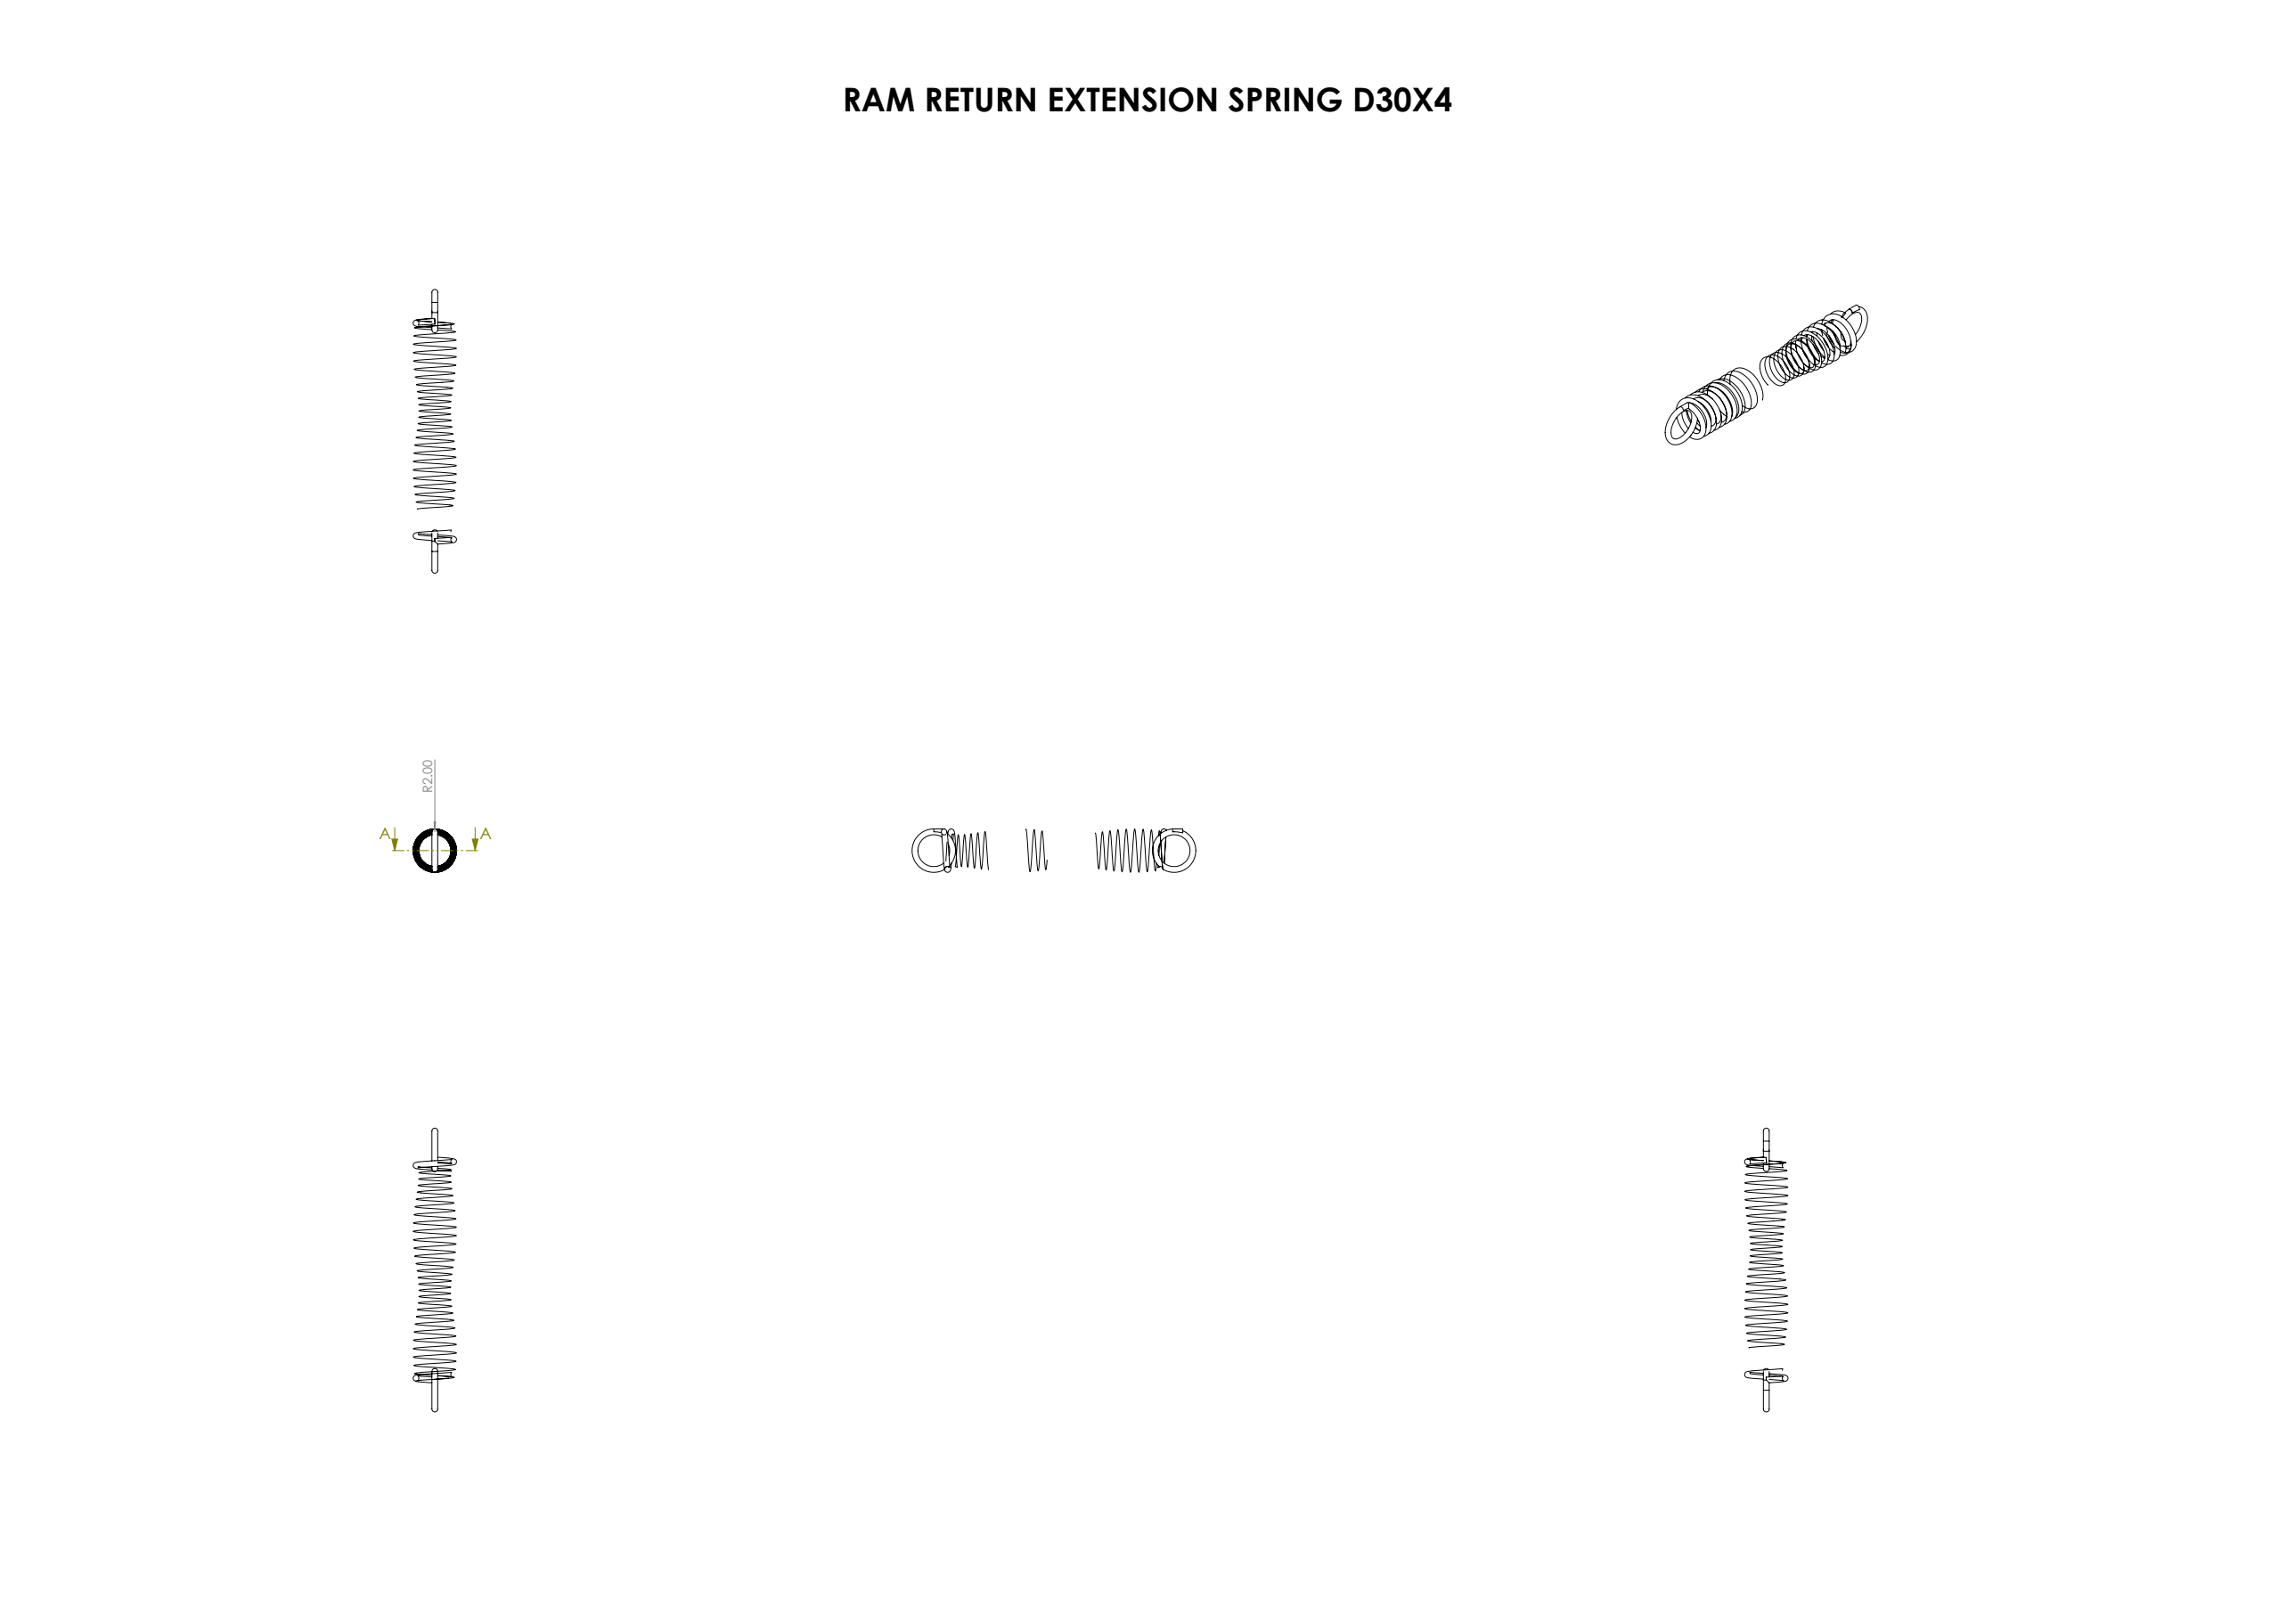
ISO-10303-21;
HEADER;
/* Generated by software containing ST-Developer
 * from STEP Tools, Inc. (www.steptools.com) 
 */

FILE_DESCRIPTION(
/* description */ (''),
/* implementation_level */ '2;1');

FILE_NAME(
/* name */ '14_Ram_Return_Extension_Spring_D30x4.step',
/* time_stamp */ '2026-10-20T10:03:03-07:00',
/* author */ (''),
/* organization */ (''),
/* preprocessor_version */ 'ST-DEVELOPER v20.2',
/* originating_system */ 'Autodesk Translation Framework v15.15.0.0',
/* authorisation */ '');

FILE_SCHEMA (('AUTOMOTIVE_DESIGN { 1 0 10303 214 3 1 1 }'));
ENDSEC;

DATA;
#10=MECHANICAL_DESIGN_GEOMETRIC_PRESENTATION_REPRESENTATION('',(#536),#71492);
#378=TOROIDAL_SURFACE('',#30165,1.30000000000001,0.199999999999999);
#379=TOROIDAL_SURFACE('',#30175,1.29999999999998,0.199999999999999);
#393=SHAPE_REPRESENTATION_RELATIONSHIP('SRR','None',#71614,#412);
#412=ADVANCED_BREP_SHAPE_REPRESENTATION('',(#431),#71484);
#431=MANIFOLD_SOLID_BREP('Spring',#28470);
#536=STYLED_ITEM('',(#71887),#431);
#890=B_SPLINE_CURVE_WITH_KNOTS('',3,(#50566,#50567,#50568,#50569,#50570,
#50571,#50572,#50573,#50574,#50575,#50576,#50577),.UNSPECIFIED.,.F.,.F.,
(4,2,2,2,2,4),(-0.933147704973241,-0.868188382212497,-0.834902175531159,
-0.786275576815645,-0.713790971965885,-0.697816473428944),.UNSPECIFIED.);
#891=B_SPLINE_CURVE_WITH_KNOTS('',3,(#50579,#50580,#50581,#50582,#50583,
#50584),.UNSPECIFIED.,.F.,.F.,(4,2,4),(1.52674033862511,1.66437329412415,
1.90849204295496),.UNSPECIFIED.);
#892=B_SPLINE_CURVE_WITH_KNOTS('',3,(#50585,#50586,#50587,#50588,#50589,
#50590,#50591,#50592,#50593,#50594,#50595,#50596,#50597,#50598,#50599,#50600,
#50601,#50602,#50603,#50604,#50605,#50606,#50607,#50608,#50609,#50610,#50611,
#50612,#50613,#50614,#50615,#50616,#50617,#50618,#50619,#50620,#50621,#50622,
#50623,#50624),.UNSPECIFIED.,.F.,.F.,(4,2,2,2,2,2,2,2,2,2,2,2,2,2,2,2,2,
2,2,4),(-0.697816473428944,-0.641492100456325,-0.561892654258354,-0.487270261093736,
-0.415523326738581,-0.352999977835186,-0.297288562200619,-0.245809461273269,
-0.188090467029938,-0.125165205371812,-0.0693938271837363,-0.0288166579795215,
-0.011031688571819,-0.00807673967083518,-0.00722367058716677,-0.00670135601612909,
-0.00622856149277745,-0.00563313335098952,-0.00468105421360917,0.),
 .UNSPECIFIED.);
#893=B_SPLINE_CURVE_WITH_KNOTS('',3,(#50626,#50627,#50628,#50629,#50630,
#50631,#50632,#50633,#50634,#50635,#50636,#50637,#50638,#50639,#50640,#50641,
#50642,#50643,#50644,#50645,#50646,#50647,#50648,#50649,#50650,#50651,#50652,
#50653,#50654,#50655,#50656,#50657,#50658,#50659,#50660,#50661,#50662,#50663,
#50664,#50665,#50666,#50667,#50668,#50669,#50670,#50671,#50672,#50673,#50674,
#50675,#50676,#50677,#50678,#50679,#50680,#50681,#50682,#50683,#50684,#50685,
#50686,#50687,#50688,#50689,#50690,#50691,#50692,#50693,#50694,#50695,#50696,
#50697,#50698,#50699,#50700,#50701,#50702,#50703),.UNSPECIFIED.,.T.,.F.,
(4,2,2,2,2,2,2,2,2,2,2,2,2,2,2,2,2,2,2,2,2,2,2,2,2,2,2,2,2,2,2,2,2,2,2,
2,2,2,4),(-1.16741385635012,-1.10893818912616,-1.06985976541729,-1.01498651099856,
-0.957285325740818,-0.898716427496627,-0.845101968396542,-0.7947628116729,
-0.745735950293246,-0.70071813649017,-0.666843371188012,-0.652997165338416,
-0.650589913669786,-0.649860176796543,-0.649408501557424,-0.649035642498711,
-0.64859072183499,-0.64786537956541,-0.645071095706766,-0.607574421195404,
-0.548734010794119,-0.48697591956556,-0.422962984513004,-0.359428990992207,
-0.305338489109769,-0.258926095287273,-0.213872662481025,-0.174949340171218,
-0.126693953481541,-0.0878751286972278,-0.0691962799768968,-0.066111534629531,
-0.0652308285619241,-0.0646975390346177,-0.0642131862427494,-0.0636068772368167,
-0.0626447206708484,-0.0580389183869797,0.),.UNSPECIFIED.);
#894=B_SPLINE_CURVE_WITH_KNOTS('',3,(#50706,#50707,#50708,#50709,#50710,
#50711),.UNSPECIFIED.,.F.,.F.,(4,2,4),(0.,0.505462201201323,0.508054856552492),
 .UNSPECIFIED.);
#895=B_SPLINE_CURVE_WITH_KNOTS('',3,(#50713,#50714,#50715,#50716,#50717,
#50718,#50719,#50720,#50721,#50722,#50723,#50724,#50725,#50726,#50727,#50728,
#50729,#50730,#50731),.UNSPECIFIED.,.F.,.F.,(4,2,2,2,3,2,2,2,4),(-0.23884634225481,
-0.226840467123682,-0.146855278175233,-0.0717726254858313,0.,0.0717726254858312,
0.146855278175234,0.226840467123682,0.238846342254813),.UNSPECIFIED.);
#896=B_SPLINE_CURVE_WITH_KNOTS('',3,(#50733,#50734,#50735,#50736,#50737,
#50738),.UNSPECIFIED.,.F.,.F.,(4,2,4),(-0.00355989556968658,0.,0.694034650560975),
 .UNSPECIFIED.);
#897=B_SPLINE_CURVE_WITH_KNOTS('',3,(#50740,#50741,#50742,#50743,#50744,
#50745),.UNSPECIFIED.,.F.,.F.,(4,2,4),(0.,0.0964705143506219,0.100030271138855),
 .UNSPECIFIED.);
#898=B_SPLINE_CURVE_WITH_KNOTS('',3,(#50747,#50748,#50749,#50750,#50751,
#50752,#50753,#50754,#50755,#50756,#50757,#50758,#50759,#50760,#50761,#50762,
#50763,#50764,#50765),.UNSPECIFIED.,.F.,.F.,(4,2,2,2,3,2,2,2,4),(0.891901698199051,
0.964304578588269,1.03849807176645,1.11257300217037,1.18656345354505,1.26055390491972,
1.33462883532365,1.40882232850183,1.48122520889105),.UNSPECIFIED.);
#899=B_SPLINE_CURVE_WITH_KNOTS('',3,(#50766,#50767,#50768,#50769,#50770,
#50771),.UNSPECIFIED.,.F.,.F.,(4,2,4),(-0.00355989556973241,0.,0.0964742753718417),
 .UNSPECIFIED.);
#900=B_SPLINE_CURVE_WITH_KNOTS('',3,(#50787,#50788,#50789,#50790,#50791,
#50792),.UNSPECIFIED.,.F.,.F.,(4,2,4),(9.80464399094971E-6,0.571610756625481,
0.573957203361489),.UNSPECIFIED.);
#901=B_SPLINE_CURVE_WITH_KNOTS('',3,(#50794,#50795,#50796,#50797,#50798,
#50799,#50800,#50801,#50802,#50803,#50804),.UNSPECIFIED.,.F.,.F.,(4,3,2,
2,4),(-0.000224177666558713,0.,0.070831562509613,0.146325160065373,0.2126836341045),
 .UNSPECIFIED.);
#902=B_SPLINE_CURVE_WITH_KNOTS('',3,(#50806,#50807,#50808,#50809,#50810,
#50811),.UNSPECIFIED.,.F.,.F.,(4,2,4),(5.93567910240686,6.07331205917363,
6.14204532250066),.UNSPECIFIED.);
#903=B_SPLINE_CURVE_WITH_KNOTS('',3,(#50813,#50814,#50815,#50816,#50817,
#50818,#50819,#50820,#50821,#50822,#50823,#50824,#50825,#50826,#50827,#50828,
#50829,#50830,#50831,#50832,#50833,#50834,#50835,#50836,#50837,#50838),
 .UNSPECIFIED.,.F.,.F.,(4,2,2,2,2,2,2,2,2,2,2,2,4),(-0.217220359894287,
-0.188091234086745,-0.125165638249208,-0.0693942084995795,-0.0288171491726731,
-0.0110319711967647,-0.00807696643551894,-0.00722387847193592,-0.00670155176446524,
-0.00622874591968683,-0.00563330291795246,-0.0046811987490239,0.),
 .UNSPECIFIED.);
#904=B_SPLINE_CURVE_WITH_KNOTS('',3,(#50840,#50841,#50842,#50843,#50844,
#50845,#50846,#50847,#50848,#50849,#50850,#50851,#50852,#50853,#50854,#50855,
#50856,#50857),.UNSPECIFIED.,.F.,.F.,(4,2,2,2,2,2,2,2,4),(-0.631559418815847,
-0.620592602298802,-0.55666742562014,-0.487473041324762,-0.420697012696697,
-0.353000616097942,-0.297289069423837,-0.245809975607455,-0.217220359894287),
 .UNSPECIFIED.);
#905=B_SPLINE_CURVE_WITH_KNOTS('',3,(#50858,#50859,#50860,#50861,#50862,
#50863),.UNSPECIFIED.,.F.,.F.,(4,2,4),(-0.00341976532710713,0.,0.574420226027791),
 .UNSPECIFIED.);
#906=B_SPLINE_CURVE_WITH_KNOTS('',3,(#50865,#50866,#50867,#50868,#50869,
#50870,#50871,#50872,#50873,#50874,#50875,#50876,#50877,#50878,#50879,#50880,
#50881,#50882,#50883,#50884,#50885,#50886,#50887,#50888,#50889,#50890,#50891,
#50892,#50893,#50894,#50895,#50896,#50897,#50898,#50899,#50900,#50901,#50902,
#50903,#50904,#50905,#50906,#50907,#50908,#50909,#50910,#50911,#50912,#50913,
#50914,#50915,#50916,#50917,#50918,#50919,#50920,#50921,#50922,#50923,#50924,
#50925,#50926,#50927,#50928,#50929,#50930,#50931,#50932,#50933,#50934,#50935,
#50936,#50937,#50938,#50939,#50940,#50941,#50942),.UNSPECIFIED.,.T.,.F.,
(4,2,2,2,2,2,2,2,2,2,2,2,2,2,2,2,2,2,2,2,2,2,2,2,2,2,2,2,2,2,2,2,2,2,2,
2,2,2,4),(-1.17168724851018,-1.13237503013972,-1.09879160541631,-1.03889691152247,
-0.981512507143146,-0.933213815656585,-0.888967230915786,-0.842464807937823,
-0.794362427770576,-0.753634236924923,-0.729805391435721,-0.726300945076248,
-0.725393129119785,-0.724861929520477,-0.724439462673908,-0.723953337160863,
-0.723043143227618,-0.7198098911947,-0.676758603427299,-0.614155893881885,
-0.553909544915966,-0.497500965420826,-0.437567654472521,-0.378252271962478,
-0.324152481036834,-0.273011005634134,-0.22337038625395,-0.178756642448113,
-0.146924605801202,-0.134819177627514,-0.133668424425745,-0.133121159543081,
-0.132739051473177,-0.132344954721629,-0.131807139835994,-0.130466280257678,
-0.116500318328084,-0.0541945170664063,0.),.UNSPECIFIED.);
#907=B_SPLINE_CURVE_WITH_KNOTS('',3,(#50950,#50951,#50952,#50953,#50954,
#50955,#50956,#50957,#50958,#50959,#50960,#50961,#50962,#50963,#50964,#50965),
 .UNSPECIFIED.,.F.,.F.,(4,2,2,2,2,2,2,4),(-0.892813994576797,-0.891702748036019,
-0.737380938279843,-0.613095387365794,-0.519181223685694,-0.442588537124146,
-0.369088033168532,-0.363543775985196),.UNSPECIFIED.);
#908=B_SPLINE_CURVE_WITH_KNOTS('',3,(#56488,#56489,#56490,#56491,#56492,
#56493,#56494,#56495,#56496,#56497,#56498,#56499,#56500,#56501,#56502,#56503,
#56504,#56505,#56506,#56507,#56508,#56509,#56510,#56511,#56512,#56513,#56514,
#56515,#56516,#56517,#56518,#56519,#56520,#56521,#56522,#56523,#56524,#56525,
#56526,#56527,#56528,#56529,#56530,#56531,#56532,#56533,#56534,#56535,#56536,
#56537,#56538,#56539,#56540,#56541,#56542,#56543,#56544,#56545,#56546,#56547,
#56548,#56549,#56550,#56551,#56552,#56553,#56554,#56555,#56556,#56557,#56558,
#56559,#56560,#56561,#56562,#56563,#56564,#56565,#56566,#56567,#56568,#56569,
#56570,#56571,#56572,#56573,#56574,#56575,#56576,#56577,#56578,#56579,#56580,
#56581,#56582,#56583,#56584,#56585,#56586,#56587,#56588,#56589,#56590,#56591,
#56592,#56593,#56594,#56595,#56596,#56597,#56598,#56599,#56600,#56601,#56602,
#56603,#56604,#56605,#56606,#56607,#56608,#56609,#56610,#56611,#56612,#56613,
#56614,#56615,#56616,#56617,#56618,#56619,#56620,#56621,#56622,#56623,#56624,
#56625,#56626,#56627,#56628,#56629,#56630,#56631,#56632,#56633,#56634,#56635,
#56636,#56637,#56638,#56639,#56640,#56641,#56642,#56643,#56644,#56645,#56646,
#56647,#56648,#56649,#56650,#56651,#56652,#56653,#56654,#56655,#56656,#56657,
#56658,#56659,#56660,#56661,#56662,#56663,#56664,#56665,#56666,#56667,#56668,
#56669,#56670,#56671,#56672,#56673,#56674,#56675,#56676,#56677,#56678,#56679,
#56680,#56681,#56682,#56683,#56684,#56685,#56686,#56687,#56688,#56689,#56690,
#56691,#56692,#56693,#56694,#56695,#56696,#56697,#56698,#56699,#56700,#56701,
#56702,#56703,#56704,#56705,#56706,#56707,#56708,#56709,#56710,#56711,#56712,
#56713,#56714,#56715,#56716,#56717,#56718,#56719,#56720,#56721,#56722,#56723,
#56724,#56725,#56726,#56727,#56728,#56729,#56730,#56731,#56732,#56733,#56734,
#56735,#56736,#56737,#56738,#56739,#56740,#56741,#56742,#56743,#56744,#56745,
#56746,#56747,#56748,#56749,#56750,#56751,#56752,#56753,#56754,#56755,#56756,
#56757,#56758,#56759,#56760,#56761,#56762,#56763,#56764,#56765,#56766,#56767,
#56768,#56769,#56770,#56771,#56772,#56773,#56774,#56775,#56776,#56777,#56778,
#56779,#56780,#56781,#56782,#56783,#56784,#56785,#56786,#56787,#56788,#56789,
#56790,#56791,#56792,#56793,#56794,#56795,#56796,#56797,#56798,#56799,#56800,
#56801,#56802,#56803,#56804,#56805,#56806,#56807,#56808,#56809,#56810,#56811,
#56812,#56813,#56814,#56815,#56816,#56817,#56818,#56819,#56820,#56821,#56822,
#56823,#56824,#56825,#56826,#56827,#56828,#56829,#56830,#56831,#56832,#56833,
#56834,#56835,#56836,#56837,#56838,#56839,#56840,#56841,#56842,#56843,#56844,
#56845,#56846,#56847,#56848,#56849,#56850,#56851,#56852,#56853,#56854,#56855,
#56856,#56857,#56858,#56859,#56860,#56861,#56862,#56863,#56864,#56865,#56866,
#56867,#56868,#56869,#56870,#56871,#56872,#56873,#56874,#56875,#56876,#56877,
#56878,#56879,#56880,#56881,#56882,#56883,#56884,#56885,#56886,#56887,#56888,
#56889,#56890,#56891,#56892,#56893,#56894,#56895,#56896,#56897,#56898,#56899,
#56900,#56901,#56902,#56903,#56904,#56905,#56906,#56907,#56908,#56909,#56910,
#56911,#56912,#56913,#56914,#56915,#56916,#56917,#56918,#56919,#56920,#56921,
#56922,#56923,#56924,#56925,#56926,#56927,#56928,#56929,#56930,#56931,#56932,
#56933,#56934,#56935,#56936,#56937,#56938,#56939,#56940,#56941,#56942,#56943,
#56944,#56945,#56946,#56947,#56948,#56949,#56950,#56951,#56952,#56953,#56954,
#56955,#56956,#56957,#56958,#56959,#56960,#56961,#56962,#56963,#56964,#56965,
#56966,#56967,#56968,#56969,#56970,#56971,#56972,#56973,#56974,#56975,#56976,
#56977,#56978,#56979,#56980,#56981,#56982,#56983,#56984,#56985,#56986,#56987,
#56988,#56989),.UNSPECIFIED.,.F.,.F.,(4,1,1,1,1,1,1,1,1,1,1,1,1,1,1,1,1,
1,1,1,1,1,1,1,1,1,1,1,1,1,1,1,1,1,1,1,1,1,1,1,1,1,1,1,1,1,1,1,1,1,1,1,1,
1,1,1,1,1,1,1,1,1,1,1,1,1,1,1,1,1,1,1,1,1,1,1,1,1,1,1,1,1,1,1,1,1,1,1,1,
1,1,1,1,1,1,1,1,1,1,1,1,1,1,1,1,1,1,1,1,1,1,1,1,1,1,1,1,1,1,1,1,1,1,1,1,
1,1,1,1,1,1,1,1,1,1,1,1,1,1,1,1,1,1,1,1,1,1,1,1,1,1,1,1,1,1,1,1,1,1,1,1,
1,1,1,1,1,1,1,1,1,1,1,1,1,1,1,1,1,1,1,1,1,1,1,1,1,1,1,1,1,1,1,1,1,1,1,1,
1,1,1,1,1,1,1,1,1,1,1,1,1,1,1,1,1,1,1,1,1,1,1,1,1,1,1,1,1,1,1,1,1,1,1,1,
1,1,1,1,1,1,1,1,1,1,1,1,1,1,1,1,1,1,1,1,1,1,1,1,1,1,1,1,1,1,1,1,1,1,1,1,
1,1,1,1,1,1,1,1,1,1,1,1,1,1,1,1,1,1,1,1,1,1,1,1,1,1,1,1,1,1,1,1,1,1,1,1,
1,1,1,1,1,1,1,1,1,1,1,1,1,1,1,1,1,1,1,1,1,1,1,1,1,1,1,1,1,1,1,1,1,1,1,1,
1,1,1,1,1,1,1,1,1,1,1,1,1,1,1,1,1,1,1,1,1,1,1,1,1,1,1,1,1,1,1,1,1,1,1,1,
1,1,1,1,1,1,1,1,1,1,1,1,1,1,1,1,1,1,1,1,1,1,1,1,1,1,1,1,1,1,1,1,1,1,1,1,
1,1,1,1,1,1,1,1,1,1,1,1,1,1,1,1,1,1,1,1,1,1,1,1,1,1,1,1,1,1,1,1,1,1,1,1,
1,1,1,1,1,1,1,1,1,1,1,1,1,1,1,1,1,1,1,1,1,1,1,1,1,1,1,1,1,1,1,1,1,1,1,1,
1,1,1,1,1,1,1,1,1,1,1,1,1,1,4),(0.000669054243018642,0.00167410714285714,
0.00223214285714286,0.00334821428571429,0.00446428571428571,0.00558035714285714,
0.00669642857142857,0.00892857142857143,0.0111607142857143,0.0133928571428571,
0.015625,0.0178571428571429,0.0200892857142857,0.0223214285714286,0.0245535714285714,
0.0267857142857143,0.0290178571428571,0.03125,0.0334821428571429,0.0357142857142857,
0.0379464285714286,0.0401785714285714,0.0424107142857143,0.0446428571428571,
0.046875,0.0491071428571428,0.0513392857142857,0.0535714285714286,0.0558035714285714,
0.0580357142857143,0.0602678571428571,0.0625,0.0647321428571428,0.0669642857142857,
0.0680803571428572,0.0691964285714286,0.0714285714285714,0.0736607142857143,
0.0758928571428571,0.078125,0.0803571428571428,0.0825892857142857,0.0848214285714286,
0.0870535714285714,0.0892857142857143,0.0915178571428571,0.09375,0.0959821428571428,
0.0982142857142857,0.100446428571429,0.102678571428571,0.104910714285714,
0.107142857142857,0.109375,0.111607142857143,0.113839285714286,0.116071428571429,
0.118303571428571,0.119419642857143,0.120535714285714,0.122767857142857,
0.125,0.127232142857143,0.129464285714286,0.131696428571429,0.133928571428571,
0.136160714285714,0.138392857142857,0.140625,0.142857142857143,0.144345238095238,
0.145833333333333,0.146205357142857,0.146577380952381,0.146949404761905,
0.147321428571429,0.148809523809524,0.150297619047619,0.151785714285714,
0.15327380952381,0.154761904761905,0.15625,0.157738095238095,0.160714285714286,
0.162202380952381,0.162946428571429,0.163690476190476,0.165178571428571,
0.165550595238095,0.165922619047619,0.166294642857143,0.166480654761905,
0.166666666666667,0.169312169312169,0.171957671957672,0.172839506172839,
0.173721340388007,0.174162257495591,0.174603174603175,0.177248677248677,
0.17989417989418,0.182539682539683,0.18452380952381,0.186507936507937,0.188492063492063,
0.19047619047619,0.191468253968254,0.192460317460317,0.193452380952381,
0.193948412698413,0.194444444444444,0.196428571428571,0.198412698412698,
0.200396825396825,0.202380952380952,0.202876984126984,0.203373015873016,
0.204365079365079,0.206349206349206,0.206597222222222,0.206845238095238,
0.207093253968254,0.20734126984127,0.207589285714286,0.207837301587302,
0.208333333333333,0.21031746031746,0.212301587301587,0.214285714285714,
0.216269841269841,0.218253968253968,0.220238095238095,0.222222222222222,
0.222883597883598,0.223544973544974,0.224867724867725,0.227513227513228,
0.23015873015873,0.232804232804233,0.235449735449735,0.238095238095238,
0.239583333333333,0.241071428571429,0.244047619047619,0.247023809523809,
0.25,0.25297619047619,0.255952380952381,0.258928571428571,0.260416666666667,
0.261904761904762,0.263392857142857,0.264880952380952,0.267857142857143,
0.270833333333333,0.273809523809524,0.276785714285714,0.279761904761905,
0.282738095238095,0.285714285714286,0.288690476190476,0.291666666666667,
0.294642857142857,0.297619047619048,0.300595238095238,0.303571428571429,
0.306547619047619,0.30952380952381,0.3125,0.31547619047619,0.318452380952381,
0.321428571428571,0.324404761904762,0.327380952380952,0.328869047619048,
0.330357142857143,0.333333333333333,0.336309523809524,0.339285714285714,
0.342261904761905,0.345238095238095,0.348214285714286,0.351190476190476,
0.354166666666667,0.357142857142857,0.360119047619048,0.363095238095238,
0.366071428571428,0.367559523809524,0.369047619047619,0.370535714285714,
0.37202380952381,0.373511904761905,0.375,0.376488095238095,0.37797619047619,
0.378720238095238,0.379464285714286,0.380952380952381,0.383928571428571,
0.386904761904762,0.389880952380952,0.391369047619048,0.392113095238095,
0.392857142857143,0.394345238095238,0.395833333333333,0.398809523809524,
0.401785714285714,0.404761904761905,0.407738095238095,0.40922619047619,
0.410714285714286,0.411458333333333,0.411830357142857,0.412202380952381,
0.412946428571429,0.413690476190476,0.415178571428571,0.416666666666667,
0.418154761904762,0.419642857142857,0.421130952380952,0.422619047619048,
0.424107142857143,0.425595238095238,0.427083333333333,0.427827380952381,
0.428571428571429,0.430803571428571,0.433035714285714,0.435267857142857,
0.4375,0.439732142857143,0.441964285714286,0.444196428571429,0.446428571428571,
0.447544642857143,0.448660714285714,0.450892857142857,0.453125,0.455357142857143,
0.457589285714286,0.459821428571429,0.462053571428571,0.464285714285714,
0.466517857142857,0.46875,0.470982142857143,0.472098214285714,0.473214285714286,
0.475446428571429,0.477678571428571,0.479910714285714,0.482142857142857,
0.484375,0.486607142857143,0.488839285714286,0.491071428571429,0.493303571428571,
0.495535714285714,0.497767857142857,0.5,0.502232142857143,0.504464285714286,
0.506696428571429,0.508928571428571,0.511160714285714,0.513392857142857,
0.515625,0.517857142857143,0.520089285714286,0.522321428571428,0.524553571428571,
0.526785714285714,0.529017857142857,0.53125,0.533482142857143,0.535714285714286,
0.537946428571429,0.540178571428571,0.542410714285714,0.544642857142857,
0.545200892857143,0.545758928571429,0.546875,0.549107142857143,0.551339285714286,
0.553571428571429,0.555803571428571,0.558035714285714,0.560267857142857,
0.5625,0.564732142857143,0.566964285714286,0.569196428571429,0.571428571428571,
0.573660714285714,0.575892857142857,0.578125,0.580357142857143,0.582589285714286,
0.584821428571428,0.587053571428571,0.589285714285714,0.591517857142857,
0.59375,0.595982142857143,0.598214285714286,0.600446428571428,0.602678571428571,
0.604910714285714,0.607142857142857,0.609375,0.611607142857143,0.613839285714286,
0.616071428571429,0.618303571428571,0.620535714285714,0.622767857142857,
0.625,0.627232142857143,0.629464285714286,0.631696428571429,0.633928571428571,
0.636160714285714,0.638392857142857,0.640625,0.642857142857143,0.644345238095238,
0.645833333333333,0.648809523809524,0.651785714285714,0.654761904761905,
0.657738095238095,0.660714285714286,0.663690476190476,0.665178571428571,
0.666666666666667,0.667989417989418,0.669312169312169,0.671957671957672,
0.674603174603175,0.675925925925926,0.677248677248677,0.67989417989418,
0.682539682539682,0.684523809523809,0.686507936507936,0.688492063492063,
0.69047619047619,0.692460317460317,0.694444444444444,0.696428571428571,
0.697420634920635,0.698412698412698,0.701058201058201,0.703703703703704,
0.705026455026455,0.706349206349206,0.707671957671958,0.71031746031746,
0.712301587301587,0.714285714285714,0.716517857142857,0.71875,0.720982142857143,
0.72265625,0.723214285714286,0.724702380952381,0.726190476190476,0.727678571428571,
0.729166666666667,0.730654761904762,0.732142857142857,0.733258928571428,
0.734375,0.736607142857143,0.738839285714286,0.741071428571428,0.743303571428571,
0.745535714285714,0.747767857142857,0.75,0.752232142857143,0.754464285714286,
0.756696428571428,0.758928571428571,0.761160714285714,0.763392857142857,
0.765625,0.767857142857143,0.770089285714286,0.772321428571428,0.774553571428571,
0.776785714285714,0.779017857142857,0.78125,0.783482142857143,0.785714285714286,
0.787946428571428,0.790178571428571,0.792410714285714,0.794642857142857,
0.796875,0.799107142857143,0.801339285714286,0.803571428571428,0.805803571428571,
0.808035714285714,0.810267857142857,0.8125,0.814732142857143,0.816964285714286,
0.819196428571429,0.821428571428571,0.823660714285714,0.825892857142857,
0.828125,0.830357142857143,0.832589285714286,0.834821428571428,0.837053571428571,
0.839285714285714,0.841517857142857,0.84375,0.845982142857143,0.848214285714286,
0.850446428571428,0.852678571428571,0.854910714285714,0.857142857142857,
0.859375,0.861607142857143,0.863839285714286,0.866071428571429,0.868303571428571,
0.870535714285714,0.872767857142857,0.875,0.877232142857143,0.879464285714286,
0.881696428571429,0.883928571428571,0.886160714285714,0.888392857142857,
0.890625,0.892857142857143,0.895089285714286,0.897321428571428,0.899553571428571,
0.901785714285714,0.904017857142857,0.90625,0.908482142857143,0.910714285714286,
0.912946428571429,0.915178571428571,0.917410714285714,0.919642857142857,
0.921875,0.922991071428571,0.924107142857143,0.926339285714286,0.928571428571429,
0.930803571428571,0.933035714285714,0.935267857142857,0.9375,0.939732142857143,
0.941964285714286,0.944196428571429,0.946428571428571,0.948660714285714,
0.950892857142857,0.953125,0.955357142857143,0.957589285714286,0.959821428571429,
0.962053571428571,0.964285714285714,0.966517857142857,0.96875,0.970982142857143,
0.973214285714286,0.975446428571429,0.977678571428572,0.979910714285714,
0.982142857142857,0.984375,0.986607142857143,0.988839285714286,0.991071428571429,
0.993303571428571,0.994419642857143,0.995535714285714,0.996651785714286,
0.997767857142857,0.998883928571429,0.999194256023389),.UNSPECIFIED.);
#1461=B_SPLINE_SURFACE_WITH_KNOTS('',3,3,((#50966,#50967,#50968,#50969,
#50970,#50971,#50972,#50973,#50974,#50975,#50976,#50977,#50978,#50979,#50980,
#50981,#50982,#50983,#50984,#50985,#50986,#50987,#50988,#50989,#50990,#50991,
#50992,#50993,#50994,#50995,#50996,#50997,#50998,#50999,#51000,#51001,#51002,
#51003,#51004,#51005,#51006,#51007,#51008,#51009,#51010,#51011,#51012,#51013,
#51014,#51015,#51016,#51017,#51018,#51019,#51020,#51021,#51022,#51023,#51024,
#51025,#51026,#51027,#51028,#51029,#51030,#51031,#51032,#51033,#51034,#51035,
#51036,#51037,#51038,#51039,#51040,#51041,#51042,#51043,#51044,#51045,#51046,
#51047,#51048,#51049,#51050,#51051,#51052,#51053,#51054,#51055,#51056,#51057,
#51058,#51059,#51060,#51061,#51062,#51063,#51064,#51065,#51066,#51067,#51068,
#51069,#51070,#51071,#51072,#51073,#51074,#51075,#51076,#51077,#51078,#51079,
#51080,#51081,#51082,#51083,#51084,#51085,#51086,#51087,#51088,#51089,#51090,
#51091,#51092,#51093,#51094,#51095,#51096,#51097,#51098,#51099,#51100,#51101,
#51102,#51103,#51104,#51105,#51106,#51107,#51108,#51109,#51110,#51111,#51112,
#51113,#51114,#51115,#51116,#51117,#51118,#51119,#51120,#51121,#51122,#51123,
#51124,#51125,#51126,#51127,#51128,#51129,#51130,#51131,#51132,#51133,#51134,
#51135,#51136,#51137,#51138,#51139,#51140,#51141,#51142,#51143,#51144,#51145,
#51146,#51147,#51148,#51149,#51150,#51151,#51152,#51153,#51154,#51155,#51156,
#51157,#51158,#51159,#51160,#51161,#51162,#51163,#51164,#51165,#51166,#51167,
#51168,#51169,#51170,#51171,#51172,#51173,#51174,#51175,#51176,#51177,#51178,
#51179,#51180,#51181,#51182,#51183,#51184,#51185,#51186,#51187,#51188,#51189,
#51190,#51191,#51192,#51193,#51194,#51195,#51196,#51197,#51198,#51199,#51200,
#51201,#51202,#51203,#51204,#51205,#51206,#51207,#51208,#51209,#51210,#51211,
#51212,#51213,#51214,#51215,#51216,#51217,#51218,#51219,#51220,#51221,#51222,
#51223,#51224,#51225,#51226,#51227,#51228,#51229,#51230,#51231,#51232,#51233,
#51234,#51235,#51236,#51237,#51238,#51239,#51240,#51241,#51242,#51243,#51244,
#51245,#51246,#51247,#51248,#51249,#51250,#51251,#51252,#51253,#51254,#51255,
#51256,#51257,#51258,#51259,#51260,#51261,#51262,#51263,#51264,#51265,#51266,
#51267,#51268,#51269,#51270,#51271,#51272,#51273,#51274,#51275,#51276,#51277,
#51278,#51279,#51280,#51281,#51282,#51283,#51284,#51285,#51286,#51287,#51288,
#51289,#51290,#51291,#51292,#51293,#51294,#51295,#51296,#51297,#51298,#51299,
#51300,#51301,#51302,#51303,#51304,#51305,#51306,#51307,#51308,#51309,#51310,
#51311,#51312,#51313,#51314,#51315,#51316,#51317,#51318,#51319,#51320,#51321,
#51322,#51323,#51324,#51325,#51326,#51327,#51328,#51329,#51330,#51331,#51332,
#51333,#51334,#51335,#51336,#51337,#51338,#51339,#51340,#51341,#51342,#51343,
#51344,#51345,#51346,#51347,#51348,#51349,#51350,#51351,#51352,#51353,#51354,
#51355,#51356,#51357,#51358,#51359,#51360,#51361,#51362,#51363,#51364,#51365,
#51366,#51367,#51368,#51369,#51370,#51371,#51372,#51373,#51374,#51375,#51376,
#51377,#51378,#51379,#51380,#51381,#51382,#51383,#51384,#51385,#51386,#51387,
#51388,#51389,#51390,#51391,#51392,#51393,#51394,#51395,#51396,#51397,#51398,
#51399,#51400,#51401,#51402,#51403,#51404,#51405,#51406,#51407,#51408,#51409,
#51410,#51411,#51412,#51413,#51414,#51415,#51416,#51417,#51418,#51419,#51420,
#51421,#51422,#51423,#51424,#51425,#51426,#51427,#51428,#51429,#51430,#51431,
#51432,#51433,#51434,#51435,#51436,#51437,#51438,#51439,#51440,#51441,#51442,
#51443,#51444,#51445,#51446,#51447,#51448,#51449,#51450,#51451,#51452,#51453,
#51454,#51455,#51456,#51457,#51458,#51459,#51460,#51461,#51462,#51463,#51464,
#51465,#51466,#51467),(#51468,#51469,#51470,#51471,#51472,#51473,#51474,
#51475,#51476,#51477,#51478,#51479,#51480,#51481,#51482,#51483,#51484,#51485,
#51486,#51487,#51488,#51489,#51490,#51491,#51492,#51493,#51494,#51495,#51496,
#51497,#51498,#51499,#51500,#51501,#51502,#51503,#51504,#51505,#51506,#51507,
#51508,#51509,#51510,#51511,#51512,#51513,#51514,#51515,#51516,#51517,#51518,
#51519,#51520,#51521,#51522,#51523,#51524,#51525,#51526,#51527,#51528,#51529,
#51530,#51531,#51532,#51533,#51534,#51535,#51536,#51537,#51538,#51539,#51540,
#51541,#51542,#51543,#51544,#51545,#51546,#51547,#51548,#51549,#51550,#51551,
#51552,#51553,#51554,#51555,#51556,#51557,#51558,#51559,#51560,#51561,#51562,
#51563,#51564,#51565,#51566,#51567,#51568,#51569,#51570,#51571,#51572,#51573,
#51574,#51575,#51576,#51577,#51578,#51579,#51580,#51581,#51582,#51583,#51584,
#51585,#51586,#51587,#51588,#51589,#51590,#51591,#51592,#51593,#51594,#51595,
#51596,#51597,#51598,#51599,#51600,#51601,#51602,#51603,#51604,#51605,#51606,
#51607,#51608,#51609,#51610,#51611,#51612,#51613,#51614,#51615,#51616,#51617,
#51618,#51619,#51620,#51621,#51622,#51623,#51624,#51625,#51626,#51627,#51628,
#51629,#51630,#51631,#51632,#51633,#51634,#51635,#51636,#51637,#51638,#51639,
#51640,#51641,#51642,#51643,#51644,#51645,#51646,#51647,#51648,#51649,#51650,
#51651,#51652,#51653,#51654,#51655,#51656,#51657,#51658,#51659,#51660,#51661,
#51662,#51663,#51664,#51665,#51666,#51667,#51668,#51669,#51670,#51671,#51672,
#51673,#51674,#51675,#51676,#51677,#51678,#51679,#51680,#51681,#51682,#51683,
#51684,#51685,#51686,#51687,#51688,#51689,#51690,#51691,#51692,#51693,#51694,
#51695,#51696,#51697,#51698,#51699,#51700,#51701,#51702,#51703,#51704,#51705,
#51706,#51707,#51708,#51709,#51710,#51711,#51712,#51713,#51714,#51715,#51716,
#51717,#51718,#51719,#51720,#51721,#51722,#51723,#51724,#51725,#51726,#51727,
#51728,#51729,#51730,#51731,#51732,#51733,#51734,#51735,#51736,#51737,#51738,
#51739,#51740,#51741,#51742,#51743,#51744,#51745,#51746,#51747,#51748,#51749,
#51750,#51751,#51752,#51753,#51754,#51755,#51756,#51757,#51758,#51759,#51760,
#51761,#51762,#51763,#51764,#51765,#51766,#51767,#51768,#51769,#51770,#51771,
#51772,#51773,#51774,#51775,#51776,#51777,#51778,#51779,#51780,#51781,#51782,
#51783,#51784,#51785,#51786,#51787,#51788,#51789,#51790,#51791,#51792,#51793,
#51794,#51795,#51796,#51797,#51798,#51799,#51800,#51801,#51802,#51803,#51804,
#51805,#51806,#51807,#51808,#51809,#51810,#51811,#51812,#51813,#51814,#51815,
#51816,#51817,#51818,#51819,#51820,#51821,#51822,#51823,#51824,#51825,#51826,
#51827,#51828,#51829,#51830,#51831,#51832,#51833,#51834,#51835,#51836,#51837,
#51838,#51839,#51840,#51841,#51842,#51843,#51844,#51845,#51846,#51847,#51848,
#51849,#51850,#51851,#51852,#51853,#51854,#51855,#51856,#51857,#51858,#51859,
#51860,#51861,#51862,#51863,#51864,#51865,#51866,#51867,#51868,#51869,#51870,
#51871,#51872,#51873,#51874,#51875,#51876,#51877,#51878,#51879,#51880,#51881,
#51882,#51883,#51884,#51885,#51886,#51887,#51888,#51889,#51890,#51891,#51892,
#51893,#51894,#51895,#51896,#51897,#51898,#51899,#51900,#51901,#51902,#51903,
#51904,#51905,#51906,#51907,#51908,#51909,#51910,#51911,#51912,#51913,#51914,
#51915,#51916,#51917,#51918,#51919,#51920,#51921,#51922,#51923,#51924,#51925,
#51926,#51927,#51928,#51929,#51930,#51931,#51932,#51933,#51934,#51935,#51936,
#51937,#51938,#51939,#51940,#51941,#51942,#51943,#51944,#51945,#51946,#51947,
#51948,#51949,#51950,#51951,#51952,#51953,#51954,#51955,#51956,#51957,#51958,
#51959,#51960,#51961,#51962,#51963,#51964,#51965,#51966,#51967,#51968,#51969),
(#51970,#51971,#51972,#51973,#51974,#51975,#51976,#51977,#51978,#51979,
#51980,#51981,#51982,#51983,#51984,#51985,#51986,#51987,#51988,#51989,#51990,
#51991,#51992,#51993,#51994,#51995,#51996,#51997,#51998,#51999,#52000,#52001,
#52002,#52003,#52004,#52005,#52006,#52007,#52008,#52009,#52010,#52011,#52012,
#52013,#52014,#52015,#52016,#52017,#52018,#52019,#52020,#52021,#52022,#52023,
#52024,#52025,#52026,#52027,#52028,#52029,#52030,#52031,#52032,#52033,#52034,
#52035,#52036,#52037,#52038,#52039,#52040,#52041,#52042,#52043,#52044,#52045,
#52046,#52047,#52048,#52049,#52050,#52051,#52052,#52053,#52054,#52055,#52056,
#52057,#52058,#52059,#52060,#52061,#52062,#52063,#52064,#52065,#52066,#52067,
#52068,#52069,#52070,#52071,#52072,#52073,#52074,#52075,#52076,#52077,#52078,
#52079,#52080,#52081,#52082,#52083,#52084,#52085,#52086,#52087,#52088,#52089,
#52090,#52091,#52092,#52093,#52094,#52095,#52096,#52097,#52098,#52099,#52100,
#52101,#52102,#52103,#52104,#52105,#52106,#52107,#52108,#52109,#52110,#52111,
#52112,#52113,#52114,#52115,#52116,#52117,#52118,#52119,#52120,#52121,#52122,
#52123,#52124,#52125,#52126,#52127,#52128,#52129,#52130,#52131,#52132,#52133,
#52134,#52135,#52136,#52137,#52138,#52139,#52140,#52141,#52142,#52143,#52144,
#52145,#52146,#52147,#52148,#52149,#52150,#52151,#52152,#52153,#52154,#52155,
#52156,#52157,#52158,#52159,#52160,#52161,#52162,#52163,#52164,#52165,#52166,
#52167,#52168,#52169,#52170,#52171,#52172,#52173,#52174,#52175,#52176,#52177,
#52178,#52179,#52180,#52181,#52182,#52183,#52184,#52185,#52186,#52187,#52188,
#52189,#52190,#52191,#52192,#52193,#52194,#52195,#52196,#52197,#52198,#52199,
#52200,#52201,#52202,#52203,#52204,#52205,#52206,#52207,#52208,#52209,#52210,
#52211,#52212,#52213,#52214,#52215,#52216,#52217,#52218,#52219,#52220,#52221,
#52222,#52223,#52224,#52225,#52226,#52227,#52228,#52229,#52230,#52231,#52232,
#52233,#52234,#52235,#52236,#52237,#52238,#52239,#52240,#52241,#52242,#52243,
#52244,#52245,#52246,#52247,#52248,#52249,#52250,#52251,#52252,#52253,#52254,
#52255,#52256,#52257,#52258,#52259,#52260,#52261,#52262,#52263,#52264,#52265,
#52266,#52267,#52268,#52269,#52270,#52271,#52272,#52273,#52274,#52275,#52276,
#52277,#52278,#52279,#52280,#52281,#52282,#52283,#52284,#52285,#52286,#52287,
#52288,#52289,#52290,#52291,#52292,#52293,#52294,#52295,#52296,#52297,#52298,
#52299,#52300,#52301,#52302,#52303,#52304,#52305,#52306,#52307,#52308,#52309,
#52310,#52311,#52312,#52313,#52314,#52315,#52316,#52317,#52318,#52319,#52320,
#52321,#52322,#52323,#52324,#52325,#52326,#52327,#52328,#52329,#52330,#52331,
#52332,#52333,#52334,#52335,#52336,#52337,#52338,#52339,#52340,#52341,#52342,
#52343,#52344,#52345,#52346,#52347,#52348,#52349,#52350,#52351,#52352,#52353,
#52354,#52355,#52356,#52357,#52358,#52359,#52360,#52361,#52362,#52363,#52364,
#52365,#52366,#52367,#52368,#52369,#52370,#52371,#52372,#52373,#52374,#52375,
#52376,#52377,#52378,#52379,#52380,#52381,#52382,#52383,#52384,#52385,#52386,
#52387,#52388,#52389,#52390,#52391,#52392,#52393,#52394,#52395,#52396,#52397,
#52398,#52399,#52400,#52401,#52402,#52403,#52404,#52405,#52406,#52407,#52408,
#52409,#52410,#52411,#52412,#52413,#52414,#52415,#52416,#52417,#52418,#52419,
#52420,#52421,#52422,#52423,#52424,#52425,#52426,#52427,#52428,#52429,#52430,
#52431,#52432,#52433,#52434,#52435,#52436,#52437,#52438,#52439,#52440,#52441,
#52442,#52443,#52444,#52445,#52446,#52447,#52448,#52449,#52450,#52451,#52452,
#52453,#52454,#52455,#52456,#52457,#52458,#52459,#52460,#52461,#52462,#52463,
#52464,#52465,#52466,#52467,#52468,#52469,#52470,#52471),(#52472,#52473,
#52474,#52475,#52476,#52477,#52478,#52479,#52480,#52481,#52482,#52483,#52484,
#52485,#52486,#52487,#52488,#52489,#52490,#52491,#52492,#52493,#52494,#52495,
#52496,#52497,#52498,#52499,#52500,#52501,#52502,#52503,#52504,#52505,#52506,
#52507,#52508,#52509,#52510,#52511,#52512,#52513,#52514,#52515,#52516,#52517,
#52518,#52519,#52520,#52521,#52522,#52523,#52524,#52525,#52526,#52527,#52528,
#52529,#52530,#52531,#52532,#52533,#52534,#52535,#52536,#52537,#52538,#52539,
#52540,#52541,#52542,#52543,#52544,#52545,#52546,#52547,#52548,#52549,#52550,
#52551,#52552,#52553,#52554,#52555,#52556,#52557,#52558,#52559,#52560,#52561,
#52562,#52563,#52564,#52565,#52566,#52567,#52568,#52569,#52570,#52571,#52572,
#52573,#52574,#52575,#52576,#52577,#52578,#52579,#52580,#52581,#52582,#52583,
#52584,#52585,#52586,#52587,#52588,#52589,#52590,#52591,#52592,#52593,#52594,
#52595,#52596,#52597,#52598,#52599,#52600,#52601,#52602,#52603,#52604,#52605,
#52606,#52607,#52608,#52609,#52610,#52611,#52612,#52613,#52614,#52615,#52616,
#52617,#52618,#52619,#52620,#52621,#52622,#52623,#52624,#52625,#52626,#52627,
#52628,#52629,#52630,#52631,#52632,#52633,#52634,#52635,#52636,#52637,#52638,
#52639,#52640,#52641,#52642,#52643,#52644,#52645,#52646,#52647,#52648,#52649,
#52650,#52651,#52652,#52653,#52654,#52655,#52656,#52657,#52658,#52659,#52660,
#52661,#52662,#52663,#52664,#52665,#52666,#52667,#52668,#52669,#52670,#52671,
#52672,#52673,#52674,#52675,#52676,#52677,#52678,#52679,#52680,#52681,#52682,
#52683,#52684,#52685,#52686,#52687,#52688,#52689,#52690,#52691,#52692,#52693,
#52694,#52695,#52696,#52697,#52698,#52699,#52700,#52701,#52702,#52703,#52704,
#52705,#52706,#52707,#52708,#52709,#52710,#52711,#52712,#52713,#52714,#52715,
#52716,#52717,#52718,#52719,#52720,#52721,#52722,#52723,#52724,#52725,#52726,
#52727,#52728,#52729,#52730,#52731,#52732,#52733,#52734,#52735,#52736,#52737,
#52738,#52739,#52740,#52741,#52742,#52743,#52744,#52745,#52746,#52747,#52748,
#52749,#52750,#52751,#52752,#52753,#52754,#52755,#52756,#52757,#52758,#52759,
#52760,#52761,#52762,#52763,#52764,#52765,#52766,#52767,#52768,#52769,#52770,
#52771,#52772,#52773,#52774,#52775,#52776,#52777,#52778,#52779,#52780,#52781,
#52782,#52783,#52784,#52785,#52786,#52787,#52788,#52789,#52790,#52791,#52792,
#52793,#52794,#52795,#52796,#52797,#52798,#52799,#52800,#52801,#52802,#52803,
#52804,#52805,#52806,#52807,#52808,#52809,#52810,#52811,#52812,#52813,#52814,
#52815,#52816,#52817,#52818,#52819,#52820,#52821,#52822,#52823,#52824,#52825,
#52826,#52827,#52828,#52829,#52830,#52831,#52832,#52833,#52834,#52835,#52836,
#52837,#52838,#52839,#52840,#52841,#52842,#52843,#52844,#52845,#52846,#52847,
#52848,#52849,#52850,#52851,#52852,#52853,#52854,#52855,#52856,#52857,#52858,
#52859,#52860,#52861,#52862,#52863,#52864,#52865,#52866,#52867,#52868,#52869,
#52870,#52871,#52872,#52873,#52874,#52875,#52876,#52877,#52878,#52879,#52880,
#52881,#52882,#52883,#52884,#52885,#52886,#52887,#52888,#52889,#52890,#52891,
#52892,#52893,#52894,#52895,#52896,#52897,#52898,#52899,#52900,#52901,#52902,
#52903,#52904,#52905,#52906,#52907,#52908,#52909,#52910,#52911,#52912,#52913,
#52914,#52915,#52916,#52917,#52918,#52919,#52920,#52921,#52922,#52923,#52924,
#52925,#52926,#52927,#52928,#52929,#52930,#52931,#52932,#52933,#52934,#52935,
#52936,#52937,#52938,#52939,#52940,#52941,#52942,#52943,#52944,#52945,#52946,
#52947,#52948,#52949,#52950,#52951,#52952,#52953,#52954,#52955,#52956,#52957,
#52958,#52959,#52960,#52961,#52962,#52963,#52964,#52965,#52966,#52967,#52968,
#52969,#52970,#52971,#52972,#52973),(#52974,#52975,#52976,#52977,#52978,
#52979,#52980,#52981,#52982,#52983,#52984,#52985,#52986,#52987,#52988,#52989,
#52990,#52991,#52992,#52993,#52994,#52995,#52996,#52997,#52998,#52999,#53000,
#53001,#53002,#53003,#53004,#53005,#53006,#53007,#53008,#53009,#53010,#53011,
#53012,#53013,#53014,#53015,#53016,#53017,#53018,#53019,#53020,#53021,#53022,
#53023,#53024,#53025,#53026,#53027,#53028,#53029,#53030,#53031,#53032,#53033,
#53034,#53035,#53036,#53037,#53038,#53039,#53040,#53041,#53042,#53043,#53044,
#53045,#53046,#53047,#53048,#53049,#53050,#53051,#53052,#53053,#53054,#53055,
#53056,#53057,#53058,#53059,#53060,#53061,#53062,#53063,#53064,#53065,#53066,
#53067,#53068,#53069,#53070,#53071,#53072,#53073,#53074,#53075,#53076,#53077,
#53078,#53079,#53080,#53081,#53082,#53083,#53084,#53085,#53086,#53087,#53088,
#53089,#53090,#53091,#53092,#53093,#53094,#53095,#53096,#53097,#53098,#53099,
#53100,#53101,#53102,#53103,#53104,#53105,#53106,#53107,#53108,#53109,#53110,
#53111,#53112,#53113,#53114,#53115,#53116,#53117,#53118,#53119,#53120,#53121,
#53122,#53123,#53124,#53125,#53126,#53127,#53128,#53129,#53130,#53131,#53132,
#53133,#53134,#53135,#53136,#53137,#53138,#53139,#53140,#53141,#53142,#53143,
#53144,#53145,#53146,#53147,#53148,#53149,#53150,#53151,#53152,#53153,#53154,
#53155,#53156,#53157,#53158,#53159,#53160,#53161,#53162,#53163,#53164,#53165,
#53166,#53167,#53168,#53169,#53170,#53171,#53172,#53173,#53174,#53175,#53176,
#53177,#53178,#53179,#53180,#53181,#53182,#53183,#53184,#53185,#53186,#53187,
#53188,#53189,#53190,#53191,#53192,#53193,#53194,#53195,#53196,#53197,#53198,
#53199,#53200,#53201,#53202,#53203,#53204,#53205,#53206,#53207,#53208,#53209,
#53210,#53211,#53212,#53213,#53214,#53215,#53216,#53217,#53218,#53219,#53220,
#53221,#53222,#53223,#53224,#53225,#53226,#53227,#53228,#53229,#53230,#53231,
#53232,#53233,#53234,#53235,#53236,#53237,#53238,#53239,#53240,#53241,#53242,
#53243,#53244,#53245,#53246,#53247,#53248,#53249,#53250,#53251,#53252,#53253,
#53254,#53255,#53256,#53257,#53258,#53259,#53260,#53261,#53262,#53263,#53264,
#53265,#53266,#53267,#53268,#53269,#53270,#53271,#53272,#53273,#53274,#53275,
#53276,#53277,#53278,#53279,#53280,#53281,#53282,#53283,#53284,#53285,#53286,
#53287,#53288,#53289,#53290,#53291,#53292,#53293,#53294,#53295,#53296,#53297,
#53298,#53299,#53300,#53301,#53302,#53303,#53304,#53305,#53306,#53307,#53308,
#53309,#53310,#53311,#53312,#53313,#53314,#53315,#53316,#53317,#53318,#53319,
#53320,#53321,#53322,#53323,#53324,#53325,#53326,#53327,#53328,#53329,#53330,
#53331,#53332,#53333,#53334,#53335,#53336,#53337,#53338,#53339,#53340,#53341,
#53342,#53343,#53344,#53345,#53346,#53347,#53348,#53349,#53350,#53351,#53352,
#53353,#53354,#53355,#53356,#53357,#53358,#53359,#53360,#53361,#53362,#53363,
#53364,#53365,#53366,#53367,#53368,#53369,#53370,#53371,#53372,#53373,#53374,
#53375,#53376,#53377,#53378,#53379,#53380,#53381,#53382,#53383,#53384,#53385,
#53386,#53387,#53388,#53389,#53390,#53391,#53392,#53393,#53394,#53395,#53396,
#53397,#53398,#53399,#53400,#53401,#53402,#53403,#53404,#53405,#53406,#53407,
#53408,#53409,#53410,#53411,#53412,#53413,#53414,#53415,#53416,#53417,#53418,
#53419,#53420,#53421,#53422,#53423,#53424,#53425,#53426,#53427,#53428,#53429,
#53430,#53431,#53432,#53433,#53434,#53435,#53436,#53437,#53438,#53439,#53440,
#53441,#53442,#53443,#53444,#53445,#53446,#53447,#53448,#53449,#53450,#53451,
#53452,#53453,#53454,#53455,#53456,#53457,#53458,#53459,#53460,#53461,#53462,
#53463,#53464,#53465,#53466,#53467,#53468,#53469,#53470,#53471,#53472,#53473,
#53474,#53475),(#53476,#53477,#53478,#53479,#53480,#53481,#53482,#53483,
#53484,#53485,#53486,#53487,#53488,#53489,#53490,#53491,#53492,#53493,#53494,
#53495,#53496,#53497,#53498,#53499,#53500,#53501,#53502,#53503,#53504,#53505,
#53506,#53507,#53508,#53509,#53510,#53511,#53512,#53513,#53514,#53515,#53516,
#53517,#53518,#53519,#53520,#53521,#53522,#53523,#53524,#53525,#53526,#53527,
#53528,#53529,#53530,#53531,#53532,#53533,#53534,#53535,#53536,#53537,#53538,
#53539,#53540,#53541,#53542,#53543,#53544,#53545,#53546,#53547,#53548,#53549,
#53550,#53551,#53552,#53553,#53554,#53555,#53556,#53557,#53558,#53559,#53560,
#53561,#53562,#53563,#53564,#53565,#53566,#53567,#53568,#53569,#53570,#53571,
#53572,#53573,#53574,#53575,#53576,#53577,#53578,#53579,#53580,#53581,#53582,
#53583,#53584,#53585,#53586,#53587,#53588,#53589,#53590,#53591,#53592,#53593,
#53594,#53595,#53596,#53597,#53598,#53599,#53600,#53601,#53602,#53603,#53604,
#53605,#53606,#53607,#53608,#53609,#53610,#53611,#53612,#53613,#53614,#53615,
#53616,#53617,#53618,#53619,#53620,#53621,#53622,#53623,#53624,#53625,#53626,
#53627,#53628,#53629,#53630,#53631,#53632,#53633,#53634,#53635,#53636,#53637,
#53638,#53639,#53640,#53641,#53642,#53643,#53644,#53645,#53646,#53647,#53648,
#53649,#53650,#53651,#53652,#53653,#53654,#53655,#53656,#53657,#53658,#53659,
#53660,#53661,#53662,#53663,#53664,#53665,#53666,#53667,#53668,#53669,#53670,
#53671,#53672,#53673,#53674,#53675,#53676,#53677,#53678,#53679,#53680,#53681,
#53682,#53683,#53684,#53685,#53686,#53687,#53688,#53689,#53690,#53691,#53692,
#53693,#53694,#53695,#53696,#53697,#53698,#53699,#53700,#53701,#53702,#53703,
#53704,#53705,#53706,#53707,#53708,#53709,#53710,#53711,#53712,#53713,#53714,
#53715,#53716,#53717,#53718,#53719,#53720,#53721,#53722,#53723,#53724,#53725,
#53726,#53727,#53728,#53729,#53730,#53731,#53732,#53733,#53734,#53735,#53736,
#53737,#53738,#53739,#53740,#53741,#53742,#53743,#53744,#53745,#53746,#53747,
#53748,#53749,#53750,#53751,#53752,#53753,#53754,#53755,#53756,#53757,#53758,
#53759,#53760,#53761,#53762,#53763,#53764,#53765,#53766,#53767,#53768,#53769,
#53770,#53771,#53772,#53773,#53774,#53775,#53776,#53777,#53778,#53779,#53780,
#53781,#53782,#53783,#53784,#53785,#53786,#53787,#53788,#53789,#53790,#53791,
#53792,#53793,#53794,#53795,#53796,#53797,#53798,#53799,#53800,#53801,#53802,
#53803,#53804,#53805,#53806,#53807,#53808,#53809,#53810,#53811,#53812,#53813,
#53814,#53815,#53816,#53817,#53818,#53819,#53820,#53821,#53822,#53823,#53824,
#53825,#53826,#53827,#53828,#53829,#53830,#53831,#53832,#53833,#53834,#53835,
#53836,#53837,#53838,#53839,#53840,#53841,#53842,#53843,#53844,#53845,#53846,
#53847,#53848,#53849,#53850,#53851,#53852,#53853,#53854,#53855,#53856,#53857,
#53858,#53859,#53860,#53861,#53862,#53863,#53864,#53865,#53866,#53867,#53868,
#53869,#53870,#53871,#53872,#53873,#53874,#53875,#53876,#53877,#53878,#53879,
#53880,#53881,#53882,#53883,#53884,#53885,#53886,#53887,#53888,#53889,#53890,
#53891,#53892,#53893,#53894,#53895,#53896,#53897,#53898,#53899,#53900,#53901,
#53902,#53903,#53904,#53905,#53906,#53907,#53908,#53909,#53910,#53911,#53912,
#53913,#53914,#53915,#53916,#53917,#53918,#53919,#53920,#53921,#53922,#53923,
#53924,#53925,#53926,#53927,#53928,#53929,#53930,#53931,#53932,#53933,#53934,
#53935,#53936,#53937,#53938,#53939,#53940,#53941,#53942,#53943,#53944,#53945,
#53946,#53947,#53948,#53949,#53950,#53951,#53952,#53953,#53954,#53955,#53956,
#53957,#53958,#53959,#53960,#53961,#53962,#53963,#53964,#53965,#53966,#53967,
#53968,#53969,#53970,#53971,#53972,#53973,#53974,#53975,#53976,#53977),
(#53978,#53979,#53980,#53981,#53982,#53983,#53984,#53985,#53986,#53987,
#53988,#53989,#53990,#53991,#53992,#53993,#53994,#53995,#53996,#53997,#53998,
#53999,#54000,#54001,#54002,#54003,#54004,#54005,#54006,#54007,#54008,#54009,
#54010,#54011,#54012,#54013,#54014,#54015,#54016,#54017,#54018,#54019,#54020,
#54021,#54022,#54023,#54024,#54025,#54026,#54027,#54028,#54029,#54030,#54031,
#54032,#54033,#54034,#54035,#54036,#54037,#54038,#54039,#54040,#54041,#54042,
#54043,#54044,#54045,#54046,#54047,#54048,#54049,#54050,#54051,#54052,#54053,
#54054,#54055,#54056,#54057,#54058,#54059,#54060,#54061,#54062,#54063,#54064,
#54065,#54066,#54067,#54068,#54069,#54070,#54071,#54072,#54073,#54074,#54075,
#54076,#54077,#54078,#54079,#54080,#54081,#54082,#54083,#54084,#54085,#54086,
#54087,#54088,#54089,#54090,#54091,#54092,#54093,#54094,#54095,#54096,#54097,
#54098,#54099,#54100,#54101,#54102,#54103,#54104,#54105,#54106,#54107,#54108,
#54109,#54110,#54111,#54112,#54113,#54114,#54115,#54116,#54117,#54118,#54119,
#54120,#54121,#54122,#54123,#54124,#54125,#54126,#54127,#54128,#54129,#54130,
#54131,#54132,#54133,#54134,#54135,#54136,#54137,#54138,#54139,#54140,#54141,
#54142,#54143,#54144,#54145,#54146,#54147,#54148,#54149,#54150,#54151,#54152,
#54153,#54154,#54155,#54156,#54157,#54158,#54159,#54160,#54161,#54162,#54163,
#54164,#54165,#54166,#54167,#54168,#54169,#54170,#54171,#54172,#54173,#54174,
#54175,#54176,#54177,#54178,#54179,#54180,#54181,#54182,#54183,#54184,#54185,
#54186,#54187,#54188,#54189,#54190,#54191,#54192,#54193,#54194,#54195,#54196,
#54197,#54198,#54199,#54200,#54201,#54202,#54203,#54204,#54205,#54206,#54207,
#54208,#54209,#54210,#54211,#54212,#54213,#54214,#54215,#54216,#54217,#54218,
#54219,#54220,#54221,#54222,#54223,#54224,#54225,#54226,#54227,#54228,#54229,
#54230,#54231,#54232,#54233,#54234,#54235,#54236,#54237,#54238,#54239,#54240,
#54241,#54242,#54243,#54244,#54245,#54246,#54247,#54248,#54249,#54250,#54251,
#54252,#54253,#54254,#54255,#54256,#54257,#54258,#54259,#54260,#54261,#54262,
#54263,#54264,#54265,#54266,#54267,#54268,#54269,#54270,#54271,#54272,#54273,
#54274,#54275,#54276,#54277,#54278,#54279,#54280,#54281,#54282,#54283,#54284,
#54285,#54286,#54287,#54288,#54289,#54290,#54291,#54292,#54293,#54294,#54295,
#54296,#54297,#54298,#54299,#54300,#54301,#54302,#54303,#54304,#54305,#54306,
#54307,#54308,#54309,#54310,#54311,#54312,#54313,#54314,#54315,#54316,#54317,
#54318,#54319,#54320,#54321,#54322,#54323,#54324,#54325,#54326,#54327,#54328,
#54329,#54330,#54331,#54332,#54333,#54334,#54335,#54336,#54337,#54338,#54339,
#54340,#54341,#54342,#54343,#54344,#54345,#54346,#54347,#54348,#54349,#54350,
#54351,#54352,#54353,#54354,#54355,#54356,#54357,#54358,#54359,#54360,#54361,
#54362,#54363,#54364,#54365,#54366,#54367,#54368,#54369,#54370,#54371,#54372,
#54373,#54374,#54375,#54376,#54377,#54378,#54379,#54380,#54381,#54382,#54383,
#54384,#54385,#54386,#54387,#54388,#54389,#54390,#54391,#54392,#54393,#54394,
#54395,#54396,#54397,#54398,#54399,#54400,#54401,#54402,#54403,#54404,#54405,
#54406,#54407,#54408,#54409,#54410,#54411,#54412,#54413,#54414,#54415,#54416,
#54417,#54418,#54419,#54420,#54421,#54422,#54423,#54424,#54425,#54426,#54427,
#54428,#54429,#54430,#54431,#54432,#54433,#54434,#54435,#54436,#54437,#54438,
#54439,#54440,#54441,#54442,#54443,#54444,#54445,#54446,#54447,#54448,#54449,
#54450,#54451,#54452,#54453,#54454,#54455,#54456,#54457,#54458,#54459,#54460,
#54461,#54462,#54463,#54464,#54465,#54466,#54467,#54468,#54469,#54470,#54471,
#54472,#54473,#54474,#54475,#54476,#54477,#54478,#54479),(#54480,#54481,
#54482,#54483,#54484,#54485,#54486,#54487,#54488,#54489,#54490,#54491,#54492,
#54493,#54494,#54495,#54496,#54497,#54498,#54499,#54500,#54501,#54502,#54503,
#54504,#54505,#54506,#54507,#54508,#54509,#54510,#54511,#54512,#54513,#54514,
#54515,#54516,#54517,#54518,#54519,#54520,#54521,#54522,#54523,#54524,#54525,
#54526,#54527,#54528,#54529,#54530,#54531,#54532,#54533,#54534,#54535,#54536,
#54537,#54538,#54539,#54540,#54541,#54542,#54543,#54544,#54545,#54546,#54547,
#54548,#54549,#54550,#54551,#54552,#54553,#54554,#54555,#54556,#54557,#54558,
#54559,#54560,#54561,#54562,#54563,#54564,#54565,#54566,#54567,#54568,#54569,
#54570,#54571,#54572,#54573,#54574,#54575,#54576,#54577,#54578,#54579,#54580,
#54581,#54582,#54583,#54584,#54585,#54586,#54587,#54588,#54589,#54590,#54591,
#54592,#54593,#54594,#54595,#54596,#54597,#54598,#54599,#54600,#54601,#54602,
#54603,#54604,#54605,#54606,#54607,#54608,#54609,#54610,#54611,#54612,#54613,
#54614,#54615,#54616,#54617,#54618,#54619,#54620,#54621,#54622,#54623,#54624,
#54625,#54626,#54627,#54628,#54629,#54630,#54631,#54632,#54633,#54634,#54635,
#54636,#54637,#54638,#54639,#54640,#54641,#54642,#54643,#54644,#54645,#54646,
#54647,#54648,#54649,#54650,#54651,#54652,#54653,#54654,#54655,#54656,#54657,
#54658,#54659,#54660,#54661,#54662,#54663,#54664,#54665,#54666,#54667,#54668,
#54669,#54670,#54671,#54672,#54673,#54674,#54675,#54676,#54677,#54678,#54679,
#54680,#54681,#54682,#54683,#54684,#54685,#54686,#54687,#54688,#54689,#54690,
#54691,#54692,#54693,#54694,#54695,#54696,#54697,#54698,#54699,#54700,#54701,
#54702,#54703,#54704,#54705,#54706,#54707,#54708,#54709,#54710,#54711,#54712,
#54713,#54714,#54715,#54716,#54717,#54718,#54719,#54720,#54721,#54722,#54723,
#54724,#54725,#54726,#54727,#54728,#54729,#54730,#54731,#54732,#54733,#54734,
#54735,#54736,#54737,#54738,#54739,#54740,#54741,#54742,#54743,#54744,#54745,
#54746,#54747,#54748,#54749,#54750,#54751,#54752,#54753,#54754,#54755,#54756,
#54757,#54758,#54759,#54760,#54761,#54762,#54763,#54764,#54765,#54766,#54767,
#54768,#54769,#54770,#54771,#54772,#54773,#54774,#54775,#54776,#54777,#54778,
#54779,#54780,#54781,#54782,#54783,#54784,#54785,#54786,#54787,#54788,#54789,
#54790,#54791,#54792,#54793,#54794,#54795,#54796,#54797,#54798,#54799,#54800,
#54801,#54802,#54803,#54804,#54805,#54806,#54807,#54808,#54809,#54810,#54811,
#54812,#54813,#54814,#54815,#54816,#54817,#54818,#54819,#54820,#54821,#54822,
#54823,#54824,#54825,#54826,#54827,#54828,#54829,#54830,#54831,#54832,#54833,
#54834,#54835,#54836,#54837,#54838,#54839,#54840,#54841,#54842,#54843,#54844,
#54845,#54846,#54847,#54848,#54849,#54850,#54851,#54852,#54853,#54854,#54855,
#54856,#54857,#54858,#54859,#54860,#54861,#54862,#54863,#54864,#54865,#54866,
#54867,#54868,#54869,#54870,#54871,#54872,#54873,#54874,#54875,#54876,#54877,
#54878,#54879,#54880,#54881,#54882,#54883,#54884,#54885,#54886,#54887,#54888,
#54889,#54890,#54891,#54892,#54893,#54894,#54895,#54896,#54897,#54898,#54899,
#54900,#54901,#54902,#54903,#54904,#54905,#54906,#54907,#54908,#54909,#54910,
#54911,#54912,#54913,#54914,#54915,#54916,#54917,#54918,#54919,#54920,#54921,
#54922,#54923,#54924,#54925,#54926,#54927,#54928,#54929,#54930,#54931,#54932,
#54933,#54934,#54935,#54936,#54937,#54938,#54939,#54940,#54941,#54942,#54943,
#54944,#54945,#54946,#54947,#54948,#54949,#54950,#54951,#54952,#54953,#54954,
#54955,#54956,#54957,#54958,#54959,#54960,#54961,#54962,#54963,#54964,#54965,
#54966,#54967,#54968,#54969,#54970,#54971,#54972,#54973,#54974,#54975,#54976,
#54977,#54978,#54979,#54980,#54981),(#54982,#54983,#54984,#54985,#54986,
#54987,#54988,#54989,#54990,#54991,#54992,#54993,#54994,#54995,#54996,#54997,
#54998,#54999,#55000,#55001,#55002,#55003,#55004,#55005,#55006,#55007,#55008,
#55009,#55010,#55011,#55012,#55013,#55014,#55015,#55016,#55017,#55018,#55019,
#55020,#55021,#55022,#55023,#55024,#55025,#55026,#55027,#55028,#55029,#55030,
#55031,#55032,#55033,#55034,#55035,#55036,#55037,#55038,#55039,#55040,#55041,
#55042,#55043,#55044,#55045,#55046,#55047,#55048,#55049,#55050,#55051,#55052,
#55053,#55054,#55055,#55056,#55057,#55058,#55059,#55060,#55061,#55062,#55063,
#55064,#55065,#55066,#55067,#55068,#55069,#55070,#55071,#55072,#55073,#55074,
#55075,#55076,#55077,#55078,#55079,#55080,#55081,#55082,#55083,#55084,#55085,
#55086,#55087,#55088,#55089,#55090,#55091,#55092,#55093,#55094,#55095,#55096,
#55097,#55098,#55099,#55100,#55101,#55102,#55103,#55104,#55105,#55106,#55107,
#55108,#55109,#55110,#55111,#55112,#55113,#55114,#55115,#55116,#55117,#55118,
#55119,#55120,#55121,#55122,#55123,#55124,#55125,#55126,#55127,#55128,#55129,
#55130,#55131,#55132,#55133,#55134,#55135,#55136,#55137,#55138,#55139,#55140,
#55141,#55142,#55143,#55144,#55145,#55146,#55147,#55148,#55149,#55150,#55151,
#55152,#55153,#55154,#55155,#55156,#55157,#55158,#55159,#55160,#55161,#55162,
#55163,#55164,#55165,#55166,#55167,#55168,#55169,#55170,#55171,#55172,#55173,
#55174,#55175,#55176,#55177,#55178,#55179,#55180,#55181,#55182,#55183,#55184,
#55185,#55186,#55187,#55188,#55189,#55190,#55191,#55192,#55193,#55194,#55195,
#55196,#55197,#55198,#55199,#55200,#55201,#55202,#55203,#55204,#55205,#55206,
#55207,#55208,#55209,#55210,#55211,#55212,#55213,#55214,#55215,#55216,#55217,
#55218,#55219,#55220,#55221,#55222,#55223,#55224,#55225,#55226,#55227,#55228,
#55229,#55230,#55231,#55232,#55233,#55234,#55235,#55236,#55237,#55238,#55239,
#55240,#55241,#55242,#55243,#55244,#55245,#55246,#55247,#55248,#55249,#55250,
#55251,#55252,#55253,#55254,#55255,#55256,#55257,#55258,#55259,#55260,#55261,
#55262,#55263,#55264,#55265,#55266,#55267,#55268,#55269,#55270,#55271,#55272,
#55273,#55274,#55275,#55276,#55277,#55278,#55279,#55280,#55281,#55282,#55283,
#55284,#55285,#55286,#55287,#55288,#55289,#55290,#55291,#55292,#55293,#55294,
#55295,#55296,#55297,#55298,#55299,#55300,#55301,#55302,#55303,#55304,#55305,
#55306,#55307,#55308,#55309,#55310,#55311,#55312,#55313,#55314,#55315,#55316,
#55317,#55318,#55319,#55320,#55321,#55322,#55323,#55324,#55325,#55326,#55327,
#55328,#55329,#55330,#55331,#55332,#55333,#55334,#55335,#55336,#55337,#55338,
#55339,#55340,#55341,#55342,#55343,#55344,#55345,#55346,#55347,#55348,#55349,
#55350,#55351,#55352,#55353,#55354,#55355,#55356,#55357,#55358,#55359,#55360,
#55361,#55362,#55363,#55364,#55365,#55366,#55367,#55368,#55369,#55370,#55371,
#55372,#55373,#55374,#55375,#55376,#55377,#55378,#55379,#55380,#55381,#55382,
#55383,#55384,#55385,#55386,#55387,#55388,#55389,#55390,#55391,#55392,#55393,
#55394,#55395,#55396,#55397,#55398,#55399,#55400,#55401,#55402,#55403,#55404,
#55405,#55406,#55407,#55408,#55409,#55410,#55411,#55412,#55413,#55414,#55415,
#55416,#55417,#55418,#55419,#55420,#55421,#55422,#55423,#55424,#55425,#55426,
#55427,#55428,#55429,#55430,#55431,#55432,#55433,#55434,#55435,#55436,#55437,
#55438,#55439,#55440,#55441,#55442,#55443,#55444,#55445,#55446,#55447,#55448,
#55449,#55450,#55451,#55452,#55453,#55454,#55455,#55456,#55457,#55458,#55459,
#55460,#55461,#55462,#55463,#55464,#55465,#55466,#55467,#55468,#55469,#55470,
#55471,#55472,#55473,#55474,#55475,#55476,#55477,#55478,#55479,#55480,#55481,
#55482,#55483),(#55484,#55485,#55486,#55487,#55488,#55489,#55490,#55491,
#55492,#55493,#55494,#55495,#55496,#55497,#55498,#55499,#55500,#55501,#55502,
#55503,#55504,#55505,#55506,#55507,#55508,#55509,#55510,#55511,#55512,#55513,
#55514,#55515,#55516,#55517,#55518,#55519,#55520,#55521,#55522,#55523,#55524,
#55525,#55526,#55527,#55528,#55529,#55530,#55531,#55532,#55533,#55534,#55535,
#55536,#55537,#55538,#55539,#55540,#55541,#55542,#55543,#55544,#55545,#55546,
#55547,#55548,#55549,#55550,#55551,#55552,#55553,#55554,#55555,#55556,#55557,
#55558,#55559,#55560,#55561,#55562,#55563,#55564,#55565,#55566,#55567,#55568,
#55569,#55570,#55571,#55572,#55573,#55574,#55575,#55576,#55577,#55578,#55579,
#55580,#55581,#55582,#55583,#55584,#55585,#55586,#55587,#55588,#55589,#55590,
#55591,#55592,#55593,#55594,#55595,#55596,#55597,#55598,#55599,#55600,#55601,
#55602,#55603,#55604,#55605,#55606,#55607,#55608,#55609,#55610,#55611,#55612,
#55613,#55614,#55615,#55616,#55617,#55618,#55619,#55620,#55621,#55622,#55623,
#55624,#55625,#55626,#55627,#55628,#55629,#55630,#55631,#55632,#55633,#55634,
#55635,#55636,#55637,#55638,#55639,#55640,#55641,#55642,#55643,#55644,#55645,
#55646,#55647,#55648,#55649,#55650,#55651,#55652,#55653,#55654,#55655,#55656,
#55657,#55658,#55659,#55660,#55661,#55662,#55663,#55664,#55665,#55666,#55667,
#55668,#55669,#55670,#55671,#55672,#55673,#55674,#55675,#55676,#55677,#55678,
#55679,#55680,#55681,#55682,#55683,#55684,#55685,#55686,#55687,#55688,#55689,
#55690,#55691,#55692,#55693,#55694,#55695,#55696,#55697,#55698,#55699,#55700,
#55701,#55702,#55703,#55704,#55705,#55706,#55707,#55708,#55709,#55710,#55711,
#55712,#55713,#55714,#55715,#55716,#55717,#55718,#55719,#55720,#55721,#55722,
#55723,#55724,#55725,#55726,#55727,#55728,#55729,#55730,#55731,#55732,#55733,
#55734,#55735,#55736,#55737,#55738,#55739,#55740,#55741,#55742,#55743,#55744,
#55745,#55746,#55747,#55748,#55749,#55750,#55751,#55752,#55753,#55754,#55755,
#55756,#55757,#55758,#55759,#55760,#55761,#55762,#55763,#55764,#55765,#55766,
#55767,#55768,#55769,#55770,#55771,#55772,#55773,#55774,#55775,#55776,#55777,
#55778,#55779,#55780,#55781,#55782,#55783,#55784,#55785,#55786,#55787,#55788,
#55789,#55790,#55791,#55792,#55793,#55794,#55795,#55796,#55797,#55798,#55799,
#55800,#55801,#55802,#55803,#55804,#55805,#55806,#55807,#55808,#55809,#55810,
#55811,#55812,#55813,#55814,#55815,#55816,#55817,#55818,#55819,#55820,#55821,
#55822,#55823,#55824,#55825,#55826,#55827,#55828,#55829,#55830,#55831,#55832,
#55833,#55834,#55835,#55836,#55837,#55838,#55839,#55840,#55841,#55842,#55843,
#55844,#55845,#55846,#55847,#55848,#55849,#55850,#55851,#55852,#55853,#55854,
#55855,#55856,#55857,#55858,#55859,#55860,#55861,#55862,#55863,#55864,#55865,
#55866,#55867,#55868,#55869,#55870,#55871,#55872,#55873,#55874,#55875,#55876,
#55877,#55878,#55879,#55880,#55881,#55882,#55883,#55884,#55885,#55886,#55887,
#55888,#55889,#55890,#55891,#55892,#55893,#55894,#55895,#55896,#55897,#55898,
#55899,#55900,#55901,#55902,#55903,#55904,#55905,#55906,#55907,#55908,#55909,
#55910,#55911,#55912,#55913,#55914,#55915,#55916,#55917,#55918,#55919,#55920,
#55921,#55922,#55923,#55924,#55925,#55926,#55927,#55928,#55929,#55930,#55931,
#55932,#55933,#55934,#55935,#55936,#55937,#55938,#55939,#55940,#55941,#55942,
#55943,#55944,#55945,#55946,#55947,#55948,#55949,#55950,#55951,#55952,#55953,
#55954,#55955,#55956,#55957,#55958,#55959,#55960,#55961,#55962,#55963,#55964,
#55965,#55966,#55967,#55968,#55969,#55970,#55971,#55972,#55973,#55974,#55975,
#55976,#55977,#55978,#55979,#55980,#55981,#55982,#55983,#55984,#55985),
(#55986,#55987,#55988,#55989,#55990,#55991,#55992,#55993,#55994,#55995,
#55996,#55997,#55998,#55999,#56000,#56001,#56002,#56003,#56004,#56005,#56006,
#56007,#56008,#56009,#56010,#56011,#56012,#56013,#56014,#56015,#56016,#56017,
#56018,#56019,#56020,#56021,#56022,#56023,#56024,#56025,#56026,#56027,#56028,
#56029,#56030,#56031,#56032,#56033,#56034,#56035,#56036,#56037,#56038,#56039,
#56040,#56041,#56042,#56043,#56044,#56045,#56046,#56047,#56048,#56049,#56050,
#56051,#56052,#56053,#56054,#56055,#56056,#56057,#56058,#56059,#56060,#56061,
#56062,#56063,#56064,#56065,#56066,#56067,#56068,#56069,#56070,#56071,#56072,
#56073,#56074,#56075,#56076,#56077,#56078,#56079,#56080,#56081,#56082,#56083,
#56084,#56085,#56086,#56087,#56088,#56089,#56090,#56091,#56092,#56093,#56094,
#56095,#56096,#56097,#56098,#56099,#56100,#56101,#56102,#56103,#56104,#56105,
#56106,#56107,#56108,#56109,#56110,#56111,#56112,#56113,#56114,#56115,#56116,
#56117,#56118,#56119,#56120,#56121,#56122,#56123,#56124,#56125,#56126,#56127,
#56128,#56129,#56130,#56131,#56132,#56133,#56134,#56135,#56136,#56137,#56138,
#56139,#56140,#56141,#56142,#56143,#56144,#56145,#56146,#56147,#56148,#56149,
#56150,#56151,#56152,#56153,#56154,#56155,#56156,#56157,#56158,#56159,#56160,
#56161,#56162,#56163,#56164,#56165,#56166,#56167,#56168,#56169,#56170,#56171,
#56172,#56173,#56174,#56175,#56176,#56177,#56178,#56179,#56180,#56181,#56182,
#56183,#56184,#56185,#56186,#56187,#56188,#56189,#56190,#56191,#56192,#56193,
#56194,#56195,#56196,#56197,#56198,#56199,#56200,#56201,#56202,#56203,#56204,
#56205,#56206,#56207,#56208,#56209,#56210,#56211,#56212,#56213,#56214,#56215,
#56216,#56217,#56218,#56219,#56220,#56221,#56222,#56223,#56224,#56225,#56226,
#56227,#56228,#56229,#56230,#56231,#56232,#56233,#56234,#56235,#56236,#56237,
#56238,#56239,#56240,#56241,#56242,#56243,#56244,#56245,#56246,#56247,#56248,
#56249,#56250,#56251,#56252,#56253,#56254,#56255,#56256,#56257,#56258,#56259,
#56260,#56261,#56262,#56263,#56264,#56265,#56266,#56267,#56268,#56269,#56270,
#56271,#56272,#56273,#56274,#56275,#56276,#56277,#56278,#56279,#56280,#56281,
#56282,#56283,#56284,#56285,#56286,#56287,#56288,#56289,#56290,#56291,#56292,
#56293,#56294,#56295,#56296,#56297,#56298,#56299,#56300,#56301,#56302,#56303,
#56304,#56305,#56306,#56307,#56308,#56309,#56310,#56311,#56312,#56313,#56314,
#56315,#56316,#56317,#56318,#56319,#56320,#56321,#56322,#56323,#56324,#56325,
#56326,#56327,#56328,#56329,#56330,#56331,#56332,#56333,#56334,#56335,#56336,
#56337,#56338,#56339,#56340,#56341,#56342,#56343,#56344,#56345,#56346,#56347,
#56348,#56349,#56350,#56351,#56352,#56353,#56354,#56355,#56356,#56357,#56358,
#56359,#56360,#56361,#56362,#56363,#56364,#56365,#56366,#56367,#56368,#56369,
#56370,#56371,#56372,#56373,#56374,#56375,#56376,#56377,#56378,#56379,#56380,
#56381,#56382,#56383,#56384,#56385,#56386,#56387,#56388,#56389,#56390,#56391,
#56392,#56393,#56394,#56395,#56396,#56397,#56398,#56399,#56400,#56401,#56402,
#56403,#56404,#56405,#56406,#56407,#56408,#56409,#56410,#56411,#56412,#56413,
#56414,#56415,#56416,#56417,#56418,#56419,#56420,#56421,#56422,#56423,#56424,
#56425,#56426,#56427,#56428,#56429,#56430,#56431,#56432,#56433,#56434,#56435,
#56436,#56437,#56438,#56439,#56440,#56441,#56442,#56443,#56444,#56445,#56446,
#56447,#56448,#56449,#56450,#56451,#56452,#56453,#56454,#56455,#56456,#56457,
#56458,#56459,#56460,#56461,#56462,#56463,#56464,#56465,#56466,#56467,#56468,
#56469,#56470,#56471,#56472,#56473,#56474,#56475,#56476,#56477,#56478,#56479,
#56480,#56481,#56482,#56483,#56484,#56485,#56486,#56487)),.UNSPECIFIED.,
 .T.,.F.,.F.,(4,1,1,1,1,1,1,1,4),(4,1,1,1,1,1,1,1,1,1,1,1,1,1,1,1,1,1,1,
1,1,1,1,1,1,1,1,1,1,1,1,1,1,1,1,1,1,1,1,1,1,1,1,1,1,1,1,1,1,1,1,1,1,1,1,
1,1,1,1,1,1,1,1,1,1,1,1,1,1,1,1,1,1,1,1,1,1,1,1,1,1,1,1,1,1,1,1,1,1,1,1,
1,1,1,1,1,1,1,1,1,1,1,1,1,1,1,1,1,1,1,1,1,1,1,1,1,1,1,1,1,1,1,1,1,1,1,1,
1,1,1,1,1,1,1,1,1,1,1,1,1,1,1,1,1,1,1,1,1,1,1,1,1,1,1,1,1,1,1,1,1,1,1,1,
1,1,1,1,1,1,1,1,1,1,1,1,1,1,1,1,1,1,1,1,1,1,1,1,1,1,1,1,1,1,1,1,1,1,1,1,
1,1,1,1,1,1,1,1,1,1,1,1,1,1,1,1,1,1,1,1,1,1,1,1,1,1,1,1,1,1,1,1,1,1,1,1,
1,1,1,1,1,1,1,1,1,1,1,1,1,1,1,1,1,1,1,1,1,1,1,1,1,1,1,1,1,1,1,1,1,1,1,1,
1,1,1,1,1,1,1,1,1,1,1,1,1,1,1,1,1,1,1,1,1,1,1,1,1,1,1,1,1,1,1,1,1,1,1,1,
1,1,1,1,1,1,1,1,1,1,1,1,1,1,1,1,1,1,1,1,1,1,1,1,1,1,1,1,1,1,1,1,1,1,1,1,
1,1,1,1,1,1,1,1,1,1,1,1,1,1,1,1,1,1,1,1,1,1,1,1,1,1,1,1,1,1,1,1,1,1,1,1,
1,1,1,1,1,1,1,1,1,1,1,1,1,1,1,1,1,1,1,1,1,1,1,1,1,1,1,1,1,1,1,1,1,1,1,1,
1,1,1,1,1,1,1,1,1,1,1,1,1,1,1,1,1,1,1,1,1,1,1,1,1,1,1,1,1,1,1,1,1,1,1,1,
1,1,1,1,1,1,1,1,1,1,1,1,1,1,1,1,1,1,1,1,1,1,1,1,1,1,1,1,1,1,1,1,1,1,1,1,
1,1,1,1,1,1,1,1,1,1,1,1,4),(-3.14159265358979,-2.24399475256414,-1.34639685153848,
-0.448798950512828,0.448798950512828,1.34639685153848,1.5707963267949,2.24399475256414,
3.14159265358979),(0.,0.00167410714285714,0.00223214285714286,0.00334821428571429,
0.00446428571428571,0.00558035714285714,0.00669642857142857,0.00892857142857143,
0.0111607142857143,0.0133928571428571,0.015625,0.0178571428571429,0.0200892857142857,
0.0223214285714286,0.0245535714285714,0.0267857142857143,0.0290178571428571,
0.03125,0.0334821428571429,0.0357142857142857,0.0379464285714286,0.0401785714285714,
0.0424107142857143,0.0446428571428571,0.046875,0.0491071428571428,0.0513392857142857,
0.0535714285714286,0.0558035714285714,0.0580357142857143,0.0602678571428571,
0.0625,0.0647321428571428,0.0669642857142857,0.0680803571428572,0.0691964285714286,
0.0714285714285714,0.0736607142857143,0.0758928571428571,0.078125,0.0803571428571428,
0.0825892857142857,0.0848214285714286,0.0870535714285714,0.0892857142857143,
0.0915178571428571,0.09375,0.0959821428571428,0.0982142857142857,0.100446428571429,
0.102678571428571,0.104910714285714,0.107142857142857,0.109375,0.111607142857143,
0.113839285714286,0.116071428571429,0.118303571428571,0.119419642857143,
0.120535714285714,0.122767857142857,0.125,0.127232142857143,0.129464285714286,
0.131696428571429,0.133928571428571,0.136160714285714,0.138392857142857,
0.140625,0.142857142857143,0.144345238095238,0.145833333333333,0.146205357142857,
0.146577380952381,0.146949404761905,0.147321428571429,0.148809523809524,
0.150297619047619,0.151785714285714,0.15327380952381,0.154761904761905,
0.15625,0.157738095238095,0.160714285714286,0.162202380952381,0.162946428571429,
0.163690476190476,0.165178571428571,0.165550595238095,0.165922619047619,
0.166294642857143,0.166480654761905,0.166666666666667,0.169312169312169,
0.171957671957672,0.172839506172839,0.173721340388007,0.174162257495591,
0.174603174603175,0.177248677248677,0.17989417989418,0.182539682539683,
0.18452380952381,0.186507936507937,0.188492063492063,0.19047619047619,0.191468253968254,
0.192460317460317,0.193452380952381,0.193948412698413,0.194444444444444,
0.196428571428571,0.198412698412698,0.200396825396825,0.202380952380952,
0.202876984126984,0.203373015873016,0.204365079365079,0.206349206349206,
0.206597222222222,0.206845238095238,0.207093253968254,0.20734126984127,
0.207589285714286,0.207837301587302,0.208333333333333,0.21031746031746,
0.212301587301587,0.214285714285714,0.216269841269841,0.218253968253968,
0.220238095238095,0.222222222222222,0.222883597883598,0.223544973544974,
0.224867724867725,0.227513227513228,0.23015873015873,0.232804232804233,
0.235449735449735,0.238095238095238,0.239583333333333,0.241071428571429,
0.244047619047619,0.247023809523809,0.25,0.25297619047619,0.255952380952381,
0.258928571428571,0.260416666666667,0.261904761904762,0.263392857142857,
0.264880952380952,0.267857142857143,0.270833333333333,0.273809523809524,
0.276785714285714,0.279761904761905,0.282738095238095,0.285714285714286,
0.288690476190476,0.291666666666667,0.294642857142857,0.297619047619048,
0.300595238095238,0.303571428571429,0.306547619047619,0.30952380952381,
0.3125,0.31547619047619,0.318452380952381,0.321428571428571,0.324404761904762,
0.327380952380952,0.328869047619048,0.330357142857143,0.333333333333333,
0.336309523809524,0.339285714285714,0.342261904761905,0.345238095238095,
0.348214285714286,0.351190476190476,0.354166666666667,0.357142857142857,
0.360119047619048,0.363095238095238,0.366071428571428,0.367559523809524,
0.369047619047619,0.370535714285714,0.37202380952381,0.373511904761905,
0.375,0.376488095238095,0.37797619047619,0.378720238095238,0.379464285714286,
0.380952380952381,0.383928571428571,0.386904761904762,0.389880952380952,
0.391369047619048,0.392113095238095,0.392857142857143,0.394345238095238,
0.395833333333333,0.398809523809524,0.401785714285714,0.404761904761905,
0.407738095238095,0.40922619047619,0.410714285714286,0.411458333333333,
0.411830357142857,0.412202380952381,0.412946428571429,0.413690476190476,
0.415178571428571,0.416666666666667,0.418154761904762,0.419642857142857,
0.421130952380952,0.422619047619048,0.424107142857143,0.425595238095238,
0.427083333333333,0.427827380952381,0.428571428571429,0.430803571428571,
0.433035714285714,0.435267857142857,0.4375,0.439732142857143,0.441964285714286,
0.444196428571429,0.446428571428571,0.447544642857143,0.448660714285714,
0.450892857142857,0.453125,0.455357142857143,0.457589285714286,0.459821428571429,
0.462053571428571,0.464285714285714,0.466517857142857,0.46875,0.470982142857143,
0.472098214285714,0.473214285714286,0.475446428571429,0.477678571428571,
0.479910714285714,0.482142857142857,0.484375,0.486607142857143,0.488839285714286,
0.491071428571429,0.493303571428571,0.495535714285714,0.497767857142857,
0.5,0.502232142857143,0.504464285714286,0.506696428571429,0.508928571428571,
0.511160714285714,0.513392857142857,0.515625,0.517857142857143,0.520089285714286,
0.522321428571428,0.524553571428571,0.526785714285714,0.529017857142857,
0.53125,0.533482142857143,0.535714285714286,0.537946428571429,0.540178571428571,
0.542410714285714,0.544642857142857,0.545200892857143,0.545758928571429,
0.546875,0.549107142857143,0.551339285714286,0.553571428571429,0.555803571428571,
0.558035714285714,0.560267857142857,0.5625,0.564732142857143,0.566964285714286,
0.569196428571429,0.571428571428571,0.573660714285714,0.575892857142857,
0.578125,0.580357142857143,0.582589285714286,0.584821428571428,0.587053571428571,
0.589285714285714,0.591517857142857,0.59375,0.595982142857143,0.598214285714286,
0.600446428571428,0.602678571428571,0.604910714285714,0.607142857142857,
0.609375,0.611607142857143,0.613839285714286,0.616071428571429,0.618303571428571,
0.620535714285714,0.622767857142857,0.625,0.627232142857143,0.629464285714286,
0.631696428571429,0.633928571428571,0.636160714285714,0.638392857142857,
0.640625,0.642857142857143,0.644345238095238,0.645833333333333,0.648809523809524,
0.651785714285714,0.654761904761905,0.657738095238095,0.660714285714286,
0.663690476190476,0.665178571428571,0.666666666666667,0.667989417989418,
0.669312169312169,0.671957671957672,0.674603174603175,0.675925925925926,
0.677248677248677,0.67989417989418,0.682539682539682,0.684523809523809,
0.686507936507936,0.688492063492063,0.69047619047619,0.692460317460317,
0.694444444444444,0.696428571428571,0.697420634920635,0.698412698412698,
0.701058201058201,0.703703703703704,0.705026455026455,0.706349206349206,
0.707671957671958,0.71031746031746,0.712301587301587,0.714285714285714,
0.716517857142857,0.71875,0.720982142857143,0.72265625,0.723214285714286,
0.724702380952381,0.726190476190476,0.727678571428571,0.729166666666667,
0.730654761904762,0.732142857142857,0.733258928571428,0.734375,0.736607142857143,
0.738839285714286,0.741071428571428,0.743303571428571,0.745535714285714,
0.747767857142857,0.75,0.752232142857143,0.754464285714286,0.756696428571428,
0.758928571428571,0.761160714285714,0.763392857142857,0.765625,0.767857142857143,
0.770089285714286,0.772321428571428,0.774553571428571,0.776785714285714,
0.779017857142857,0.78125,0.783482142857143,0.785714285714286,0.787946428571428,
0.790178571428571,0.792410714285714,0.794642857142857,0.796875,0.799107142857143,
0.801339285714286,0.803571428571428,0.805803571428571,0.808035714285714,
0.810267857142857,0.8125,0.814732142857143,0.816964285714286,0.819196428571429,
0.821428571428571,0.823660714285714,0.825892857142857,0.828125,0.830357142857143,
0.832589285714286,0.834821428571428,0.837053571428571,0.839285714285714,
0.841517857142857,0.84375,0.845982142857143,0.848214285714286,0.850446428571428,
0.852678571428571,0.854910714285714,0.857142857142857,0.859375,0.861607142857143,
0.863839285714286,0.866071428571429,0.868303571428571,0.870535714285714,
0.872767857142857,0.875,0.877232142857143,0.879464285714286,0.881696428571429,
0.883928571428571,0.886160714285714,0.888392857142857,0.890625,0.892857142857143,
0.895089285714286,0.897321428571428,0.899553571428571,0.901785714285714,
0.904017857142857,0.90625,0.908482142857143,0.910714285714286,0.912946428571429,
0.915178571428571,0.917410714285714,0.919642857142857,0.921875,0.922991071428571,
0.924107142857143,0.926339285714286,0.928571428571429,0.930803571428571,
0.933035714285714,0.935267857142857,0.9375,0.939732142857143,0.941964285714286,
0.944196428571429,0.946428571428571,0.948660714285714,0.950892857142857,
0.953125,0.955357142857143,0.957589285714286,0.959821428571429,0.962053571428571,
0.964285714285714,0.966517857142857,0.96875,0.970982142857143,0.973214285714286,
0.975446428571429,0.977678571428572,0.979910714285714,0.982142857142857,
0.984375,0.986607142857143,0.988839285714286,0.991071428571429,0.993303571428571,
0.994419642857143,0.995535714285714,0.996651785714286,0.997767857142857,
0.998883928571429,1.),.UNSPECIFIED.);
#1682=CYLINDRICAL_SURFACE('',#30170,0.199999999999999);
#1683=CYLINDRICAL_SURFACE('',#30183,0.199999999999999);
#1967=FACE_BOUND('',#5744,.T.);
#1968=FACE_BOUND('',#5745,.T.);
#1969=FACE_BOUND('',#5746,.T.);
#1970=FACE_BOUND('',#5752,.T.);
#1971=FACE_BOUND('',#5753,.T.);
#1972=FACE_BOUND('',#5758,.T.);
#1973=FACE_BOUND('',#5759,.T.);
#2523=CIRCLE('',#30166,0.199999999999999);
#2524=CIRCLE('',#30167,1.10000000000001);
#2525=CIRCLE('',#30169,0.199999999999999);
#2526=CIRCLE('',#30171,0.199999999999999);
#2527=CIRCLE('',#30174,0.2);
#2528=CIRCLE('',#30176,0.199999999999999);
#2529=CIRCLE('',#30177,1.09999999999999);
#2530=CIRCLE('',#30178,0.199999999999999);
#2531=CIRCLE('',#30180,0.2);
#2532=CIRCLE('',#30182,0.199999999999999);
#4070=FACE_OUTER_BOUND('',#5743,.T.);
#4071=FACE_OUTER_BOUND('',#5747,.T.);
#4072=FACE_OUTER_BOUND('',#5748,.T.);
#4073=FACE_OUTER_BOUND('',#5749,.T.);
#4074=FACE_OUTER_BOUND('',#5750,.T.);
#4075=FACE_OUTER_BOUND('',#5751,.T.);
#4076=FACE_OUTER_BOUND('',#5754,.T.);
#4077=FACE_OUTER_BOUND('',#5755,.T.);
#4078=FACE_OUTER_BOUND('',#5756,.T.);
#4079=FACE_OUTER_BOUND('',#5757,.T.);
#5743=EDGE_LOOP('',(#23601,#23602,#23603,#23604));
#5744=EDGE_LOOP('',(#23605,#23606,#23607));
#5745=EDGE_LOOP('',(#23608));
#5746=EDGE_LOOP('',(#23609,#23610,#23611,#23612,#23613,#23614));
#5747=EDGE_LOOP('',(#23615,#23616));
#5748=EDGE_LOOP('',(#23617,#23618,#23619,#23620,#23621,#23622));
#5749=EDGE_LOOP('',(#23623,#23624));
#5750=EDGE_LOOP('',(#23625,#23626));
#5751=EDGE_LOOP('',(#23627,#23628,#23629,#23630));
#5752=EDGE_LOOP('',(#23631,#23632,#23633,#23634,#23635,#23636,#23637));
#5753=EDGE_LOOP('',(#23638));
#5754=EDGE_LOOP('',(#23639,#23640,#23641));
#5755=EDGE_LOOP('',(#23642,#23643,#23644));
#5756=EDGE_LOOP('',(#23645,#23646,#23647,#23648,#23649));
#5757=EDGE_LOOP('',(#23650,#23651,#23652,#23653,#23654,#23655,#23656,#23657,
#23658));
#5758=EDGE_LOOP('',(#23659));
#5759=EDGE_LOOP('',(#23660));
#8242=LINE('',#50945,#10730);
#10730=VECTOR('',#35779,1.);
#13057=VERTEX_POINT('',#50561);
#13058=VERTEX_POINT('',#50564);
#13059=VERTEX_POINT('',#50565);
#13060=VERTEX_POINT('',#50578);
#13061=VERTEX_POINT('',#50625);
#13062=VERTEX_POINT('',#50704);
#13063=VERTEX_POINT('',#50705);
#13064=VERTEX_POINT('',#50712);
#13065=VERTEX_POINT('',#50732);
#13066=VERTEX_POINT('',#50739);
#13067=VERTEX_POINT('',#50746);
#13068=VERTEX_POINT('',#50780);
#13069=VERTEX_POINT('',#50783);
#13070=VERTEX_POINT('',#50784);
#13071=VERTEX_POINT('',#50786);
#13072=VERTEX_POINT('',#50793);
#13073=VERTEX_POINT('',#50805);
#13074=VERTEX_POINT('',#50812);
#13075=VERTEX_POINT('',#50839);
#13076=VERTEX_POINT('',#50864);
#13077=VERTEX_POINT('',#50944);
#16684=EDGE_CURVE('',#13057,#13057,#2523,.T.);
#16685=EDGE_CURVE('',#13057,#13057,#2524,.T.);
#16686=EDGE_CURVE('',#13058,#13059,#890,.T.);
#16687=EDGE_CURVE('',#13060,#13058,#891,.T.);
#16688=EDGE_CURVE('',#13059,#13060,#892,.T.);
#16689=EDGE_CURVE('',#13061,#13061,#893,.T.);
#16690=EDGE_CURVE('',#13062,#13063,#894,.T.);
#16691=EDGE_CURVE('',#13064,#13062,#895,.T.);
#16692=EDGE_CURVE('',#13065,#13064,#896,.T.);
#16693=EDGE_CURVE('',#13066,#13065,#897,.T.);
#16694=EDGE_CURVE('',#13067,#13066,#898,.T.);
#16695=EDGE_CURVE('',#13063,#13067,#899,.T.);
#16696=EDGE_CURVE('',#13066,#13067,#2525,.T.);
#16697=EDGE_CURVE('',#13064,#13062,#2526,.T.);
#16698=EDGE_CURVE('',#13060,#13058,#2527,.T.);
#16699=EDGE_CURVE('',#13068,#13068,#2528,.T.);
#16700=EDGE_CURVE('',#13068,#13068,#2529,.T.);
#16701=EDGE_CURVE('',#13069,#13070,#2530,.T.);
#16702=EDGE_CURVE('',#13071,#13070,#900,.T.);
#16703=EDGE_CURVE('',#13072,#13071,#901,.T.);
#16704=EDGE_CURVE('',#13073,#13072,#902,.T.);
#16705=EDGE_CURVE('',#13074,#13073,#903,.T.);
#16706=EDGE_CURVE('',#13075,#13074,#904,.T.);
#16707=EDGE_CURVE('',#13069,#13075,#905,.T.);
#16708=EDGE_CURVE('',#13076,#13076,#906,.T.);
#16709=EDGE_CURVE('',#13072,#13077,#8242,.T.);
#16710=EDGE_CURVE('',#13077,#13073,#2531,.T.);
#16711=EDGE_CURVE('',#13077,#13071,#2532,.T.);
#16712=EDGE_CURVE('',#13077,#13075,#907,.T.);
#16713=EDGE_CURVE('',#13059,#13074,#908,.T.);
#23601=ORIENTED_EDGE('',*,*,#16684,.F.);
#23602=ORIENTED_EDGE('',*,*,#16685,.T.);
#23603=ORIENTED_EDGE('',*,*,#16684,.T.);
#23604=ORIENTED_EDGE('',*,*,#16685,.F.);
#23605=ORIENTED_EDGE('',*,*,#16686,.F.);
#23606=ORIENTED_EDGE('',*,*,#16687,.F.);
#23607=ORIENTED_EDGE('',*,*,#16688,.F.);
#23608=ORIENTED_EDGE('',*,*,#16689,.F.);
#23609=ORIENTED_EDGE('',*,*,#16690,.F.);
#23610=ORIENTED_EDGE('',*,*,#16691,.F.);
#23611=ORIENTED_EDGE('',*,*,#16692,.F.);
#23612=ORIENTED_EDGE('',*,*,#16693,.F.);
#23613=ORIENTED_EDGE('',*,*,#16694,.F.);
#23614=ORIENTED_EDGE('',*,*,#16695,.F.);
#23615=ORIENTED_EDGE('',*,*,#16694,.T.);
#23616=ORIENTED_EDGE('',*,*,#16696,.T.);
#23617=ORIENTED_EDGE('',*,*,#16690,.T.);
#23618=ORIENTED_EDGE('',*,*,#16695,.T.);
#23619=ORIENTED_EDGE('',*,*,#16696,.F.);
#23620=ORIENTED_EDGE('',*,*,#16693,.T.);
#23621=ORIENTED_EDGE('',*,*,#16692,.T.);
#23622=ORIENTED_EDGE('',*,*,#16697,.T.);
#23623=ORIENTED_EDGE('',*,*,#16691,.T.);
#23624=ORIENTED_EDGE('',*,*,#16697,.F.);
#23625=ORIENTED_EDGE('',*,*,#16687,.T.);
#23626=ORIENTED_EDGE('',*,*,#16698,.F.);
#23627=ORIENTED_EDGE('',*,*,#16699,.F.);
#23628=ORIENTED_EDGE('',*,*,#16700,.T.);
#23629=ORIENTED_EDGE('',*,*,#16699,.T.);
#23630=ORIENTED_EDGE('',*,*,#16700,.F.);
#23631=ORIENTED_EDGE('',*,*,#16701,.T.);
#23632=ORIENTED_EDGE('',*,*,#16702,.F.);
#23633=ORIENTED_EDGE('',*,*,#16703,.F.);
#23634=ORIENTED_EDGE('',*,*,#16704,.F.);
#23635=ORIENTED_EDGE('',*,*,#16705,.F.);
#23636=ORIENTED_EDGE('',*,*,#16706,.F.);
#23637=ORIENTED_EDGE('',*,*,#16707,.F.);
#23638=ORIENTED_EDGE('',*,*,#16708,.F.);
#23639=ORIENTED_EDGE('',*,*,#16704,.T.);
#23640=ORIENTED_EDGE('',*,*,#16709,.T.);
#23641=ORIENTED_EDGE('',*,*,#16710,.T.);
#23642=ORIENTED_EDGE('',*,*,#16703,.T.);
#23643=ORIENTED_EDGE('',*,*,#16711,.F.);
#23644=ORIENTED_EDGE('',*,*,#16709,.F.);
#23645=ORIENTED_EDGE('',*,*,#16702,.T.);
#23646=ORIENTED_EDGE('',*,*,#16701,.F.);
#23647=ORIENTED_EDGE('',*,*,#16707,.T.);
#23648=ORIENTED_EDGE('',*,*,#16712,.F.);
#23649=ORIENTED_EDGE('',*,*,#16711,.T.);
#23650=ORIENTED_EDGE('',*,*,#16688,.T.);
#23651=ORIENTED_EDGE('',*,*,#16698,.T.);
#23652=ORIENTED_EDGE('',*,*,#16686,.T.);
#23653=ORIENTED_EDGE('',*,*,#16713,.T.);
#23654=ORIENTED_EDGE('',*,*,#16705,.T.);
#23655=ORIENTED_EDGE('',*,*,#16710,.F.);
#23656=ORIENTED_EDGE('',*,*,#16712,.T.);
#23657=ORIENTED_EDGE('',*,*,#16706,.T.);
#23658=ORIENTED_EDGE('',*,*,#16713,.F.);
#23659=ORIENTED_EDGE('',*,*,#16689,.T.);
#23660=ORIENTED_EDGE('',*,*,#16708,.T.);
#26747=PLANE('',#30168);
#26748=PLANE('',#30172);
#26749=PLANE('',#30173);
#26750=PLANE('',#30179);
#26751=PLANE('',#30181);
#27978=ADVANCED_FACE('',(#4070,#1967,#1968,#1969),#378,.T.);
#27979=ADVANCED_FACE('',(#4071),#26747,.T.);
#27980=ADVANCED_FACE('',(#4072),#1682,.T.);
#27981=ADVANCED_FACE('',(#4073),#26748,.F.);
#27982=ADVANCED_FACE('',(#4074),#26749,.F.);
#27983=ADVANCED_FACE('',(#4075,#1970,#1971),#379,.T.);
#27984=ADVANCED_FACE('',(#4076),#26750,.T.);
#27985=ADVANCED_FACE('',(#4077),#26751,.F.);
#27986=ADVANCED_FACE('',(#4078),#1683,.T.);
#27987=ADVANCED_FACE('',(#4079,#1972,#1973),#1461,.T.);
#28470=CLOSED_SHELL('',(#27978,#27979,#27980,#27981,#27982,#27983,#27984,
#27985,#27986,#27987));
#30164=AXIS2_PLACEMENT_3D('',#50559,#35747,#35748);
#30165=AXIS2_PLACEMENT_3D('',#50560,#35749,#35750);
#30166=AXIS2_PLACEMENT_3D('',#50562,#35751,#35752);
#30167=AXIS2_PLACEMENT_3D('',#50563,#35753,#35754);
#30168=AXIS2_PLACEMENT_3D('',#50772,#35755,#35756);
#30169=AXIS2_PLACEMENT_3D('',#50773,#35757,#35758);
#30170=AXIS2_PLACEMENT_3D('',#50774,#35759,#35760);
#30171=AXIS2_PLACEMENT_3D('',#50775,#35761,#35762);
#30172=AXIS2_PLACEMENT_3D('',#50776,#35763,#35764);
#30173=AXIS2_PLACEMENT_3D('',#50777,#35765,#35766);
#30174=AXIS2_PLACEMENT_3D('',#50778,#35767,#35768);
#30175=AXIS2_PLACEMENT_3D('',#50779,#35769,#35770);
#30176=AXIS2_PLACEMENT_3D('',#50781,#35771,#35772);
#30177=AXIS2_PLACEMENT_3D('',#50782,#35773,#35774);
#30178=AXIS2_PLACEMENT_3D('',#50785,#35775,#35776);
#30179=AXIS2_PLACEMENT_3D('',#50943,#35777,#35778);
#30180=AXIS2_PLACEMENT_3D('',#50946,#35780,#35781);
#30181=AXIS2_PLACEMENT_3D('',#50947,#35782,#35783);
#30182=AXIS2_PLACEMENT_3D('',#50948,#35784,#35785);
#30183=AXIS2_PLACEMENT_3D('',#50949,#35786,#35787);
#35747=DIRECTION('axis',(0.,0.,1.));
#35748=DIRECTION('refdir',(1.,0.,0.));
#35749=DIRECTION('center_axis',(-1.,0.,0.));
#35750=DIRECTION('ref_axis',(0.,0.,1.));
#35751=DIRECTION('center_axis',(0.,-1.,1.22464679914735E-16));
#35752=DIRECTION('ref_axis',(0.,-1.22464679914735E-16,-1.));
#35753=DIRECTION('center_axis',(1.,0.,0.));
#35754=DIRECTION('ref_axis',(0.,0.,1.));
#35755=DIRECTION('center_axis',(0.,0.,1.));
#35756=DIRECTION('ref_axis',(1.,0.,0.));
#35757=DIRECTION('center_axis',(0.,0.,1.));
#35758=DIRECTION('ref_axis',(1.,0.,0.));
#35759=DIRECTION('center_axis',(0.,0.,1.));
#35760=DIRECTION('ref_axis',(6.9217303377289E-15,1.,0.));
#35761=DIRECTION('center_axis',(0.,0.,1.));
#35762=DIRECTION('ref_axis',(1.,0.,0.));
#35763=DIRECTION('center_axis',(0.,0.,1.));
#35764=DIRECTION('ref_axis',(1.,0.,0.));
#35765=DIRECTION('center_axis',(-0.998217224866142,-0.00840157766811335,
0.0590913316250743));
#35766=DIRECTION('ref_axis',(0.059089238754932,0.000497329455335615,0.998252580525979));
#35767=DIRECTION('center_axis',(-0.998217224866142,-0.00840157766811335,
0.0590913316250743));
#35768=DIRECTION('ref_axis',(0.059089238754932,0.000497329455335615,0.998252580525979));
#35769=DIRECTION('center_axis',(-1.,0.,0.));
#35770=DIRECTION('ref_axis',(0.,0.,1.));
#35771=DIRECTION('center_axis',(0.,-1.,1.22464679914735E-16));
#35772=DIRECTION('ref_axis',(0.,-1.22464679914735E-16,-1.));
#35773=DIRECTION('center_axis',(1.,0.,0.));
#35774=DIRECTION('ref_axis',(0.,0.,1.));
#35775=DIRECTION('center_axis',(0.,0.,1.));
#35776=DIRECTION('ref_axis',(1.,0.,0.));
#35777=DIRECTION('center_axis',(-0.998217224843264,0.00840157766999991,
0.059091332011291));
#35778=DIRECTION('ref_axis',(0.0434273377103988,0.781407112236281,0.622508627479124));
#35779=DIRECTION('',(0.00841628444953835,0.999964582450831,0.));
#35780=DIRECTION('center_axis',(-0.998217224843264,0.00840157766999991,
0.059091332011291));
#35781=DIRECTION('ref_axis',(0.0434273377103987,0.781407112236281,0.622508627479124));
#35782=DIRECTION('center_axis',(0.,0.,1.));
#35783=DIRECTION('ref_axis',(1.,0.,0.));
#35784=DIRECTION('center_axis',(0.,0.,1.));
#35785=DIRECTION('ref_axis',(1.,0.,0.));
#35786=DIRECTION('center_axis',(0.,0.,1.));
#35787=DIRECTION('ref_axis',(-0.116141449894828,0.993232683522007,0.));
#50559=CARTESIAN_POINT('',(0.,0.,0.));
#50560=CARTESIAN_POINT('Origin',(18.5,0.,112.2));
#50561=CARTESIAN_POINT('',(18.5,-1.3471114790621E-16,111.1));
#50562=CARTESIAN_POINT('Origin',(18.5,-1.59204083889157E-16,110.9));
#50563=CARTESIAN_POINT('Origin',(18.5,0.,112.2));
#50564=CARTESIAN_POINT('',(18.4890127645178,1.40327133104537,112.729078050442));
#50565=CARTESIAN_POINT('',(18.319456010528,1.28858936270501,112.710548943691));
#50566=CARTESIAN_POINT('Ctrl Pts',(18.4890127645179,1.40327133104537,112.729078050442));
#50567=CARTESIAN_POINT('Ctrl Pts',(18.4690263934393,1.40191965211474,112.729546131244));
#50568=CARTESIAN_POINT('Ctrl Pts',(18.4493212209946,1.39790528142896,112.728584539615));
#50569=CARTESIAN_POINT('Ctrl Pts',(18.4209570524527,1.38778681836775,112.725655461841));
#50570=CARTESIAN_POINT('Ctrl Pts',(18.4116376687533,1.38366754929998,112.724420014907));
#50571=CARTESIAN_POINT('Ctrl Pts',(18.3896234532527,1.37182981375427,112.721060426925));
#50572=CARTESIAN_POINT('Ctrl Pts',(18.3774391567708,1.36337398597481,112.718799423342));
#50573=CARTESIAN_POINT('Ctrl Pts',(18.3498687355444,1.33884907188722,112.713621176115));
#50574=CARTESIAN_POINT('Ctrl Pts',(18.336256526853,1.32144069956727,112.710998260207));
#50575=CARTESIAN_POINT('Ctrl Pts',(18.3235239190592,1.29743221003086,112.710422570251));
#50576=CARTESIAN_POINT('Ctrl Pts',(18.3214048000438,1.29303642396641,112.710425791665));
#50577=CARTESIAN_POINT('Ctrl Pts',(18.3194560105972,1.28858936267476,112.710548943694));
#50578=CARTESIAN_POINT('',(18.5113942828676,1.21414296988455,113.080274071063));
#50579=CARTESIAN_POINT('Ctrl Pts',(18.5113942828676,1.21414296988456,113.080274071063));
#50580=CARTESIAN_POINT('Ctrl Pts',(18.5088122202491,1.24297666449313,113.040755400683));
#50581=CARTESIAN_POINT('Ctrl Pts',(18.5062148178964,1.26920627329322,113.000607351763));
#50582=CARTESIAN_POINT('Ctrl Pts',(18.4991940978944,1.33379276118183,112.891190706973));
#50583=CARTESIAN_POINT('Ctrl Pts',(18.4941783520461,1.37233329581525,112.811940460321));
#50584=CARTESIAN_POINT('Ctrl Pts',(18.4890127645178,1.40327133104537,112.729078050442));
#50585=CARTESIAN_POINT('Ctrl Pts',(18.3194560105972,1.28858936267476,112.710548943694));
#50586=CARTESIAN_POINT('Ctrl Pts',(18.3125847874797,1.27290950028387,112.710983164576));
#50587=CARTESIAN_POINT('Ctrl Pts',(18.3078358917878,1.25658996219521,112.712903987457));
#50588=CARTESIAN_POINT('Ctrl Pts',(18.3004473473152,1.21660861827732,112.722513325201));
#50589=CARTESIAN_POINT('Ctrl Pts',(18.2997088045305,1.19414451241967,112.731937704259));
#50590=CARTESIAN_POINT('Ctrl Pts',(18.3004369338146,1.15445099754945,112.757978862924));
#50591=CARTESIAN_POINT('Ctrl Pts',(18.3017489050252,1.13676465318605,112.774251060074));
#50592=CARTESIAN_POINT('Ctrl Pts',(18.302877988022,1.10764815299686,112.813536422119));
#50593=CARTESIAN_POINT('Ctrl Pts',(18.3026076034137,1.09682243884728,112.835175108492));
#50594=CARTESIAN_POINT('Ctrl Pts',(18.3011018541119,1.08399515770366,112.877971837947));
#50595=CARTESIAN_POINT('Ctrl Pts',(18.3000617770382,1.08107707365306,112.8987227829));
#50596=CARTESIAN_POINT('Ctrl Pts',(18.2999496538779,1.08205742545304,112.937854988679));
#50597=CARTESIAN_POINT('Ctrl Pts',(18.3007063184796,1.08525286840353,112.955989495));
#50598=CARTESIAN_POINT('Ctrl Pts',(18.3061260446686,1.096731305641,112.989071009869));
#50599=CARTESIAN_POINT('Ctrl Pts',(18.3103918083809,1.10435368484628,113.003441617128));
#50600=CARTESIAN_POINT('Ctrl Pts',(18.3243235188135,1.12376946338441,113.030471066797));
#50601=CARTESIAN_POINT('Ctrl Pts',(18.3341715042768,1.13533680110265,113.041892724703));
#50602=CARTESIAN_POINT('Ctrl Pts',(18.3597300671205,1.15942054077883,113.060869791061));
#50603=CARTESIAN_POINT('Ctrl Pts',(18.3754928067062,1.17154637795889,113.06771640348));
#50604=CARTESIAN_POINT('Ctrl Pts',(18.4086123435342,1.19100145104539,113.076651626788));
#50605=CARTESIAN_POINT('Ctrl Pts',(18.42545279698,1.1986529463623,113.079161175487));
#50606=CARTESIAN_POINT('Ctrl Pts',(18.456006836579,1.20821075735755,113.081440251631));
#50607=CARTESIAN_POINT('Ctrl Pts',(18.4692450945303,1.21109268178609,113.081759893621));
#50608=CARTESIAN_POINT('Ctrl Pts',(18.4885594461377,1.21339556016075,113.081448360779));
#50609=CARTESIAN_POINT('Ctrl Pts',(18.4944680194924,1.21385046309689,113.081249263501));
#50610=CARTESIAN_POINT('Ctrl Pts',(18.5013683698457,1.2140880273455,113.080899240207));
#50611=CARTESIAN_POINT('Ctrl Pts',(18.5023515795956,1.21411493937423,113.080846578183));
#50612=CARTESIAN_POINT('Ctrl Pts',(18.5036186445213,1.21414067372742,113.080775120454));
#50613=CARTESIAN_POINT('Ctrl Pts',(18.5039024894183,1.21414586005045,113.080758880334));
#50614=CARTESIAN_POINT('Ctrl Pts',(18.5043601203964,1.21415328867356,113.080732322449));
#50615=CARTESIAN_POINT('Ctrl Pts',(18.5045339082962,1.21415589277799,113.080722149835));
#50616=CARTESIAN_POINT('Ctrl Pts',(18.5048650036164,1.21416044065514,113.080702603299));
#50617=CARTESIAN_POINT('Ctrl Pts',(18.5050223111988,1.2141624236228,113.080693245104));
#50618=CARTESIAN_POINT('Ctrl Pts',(18.5053777240491,1.21416650212218,113.080671940352));
#50619=CARTESIAN_POINT('Ctrl Pts',(18.5055758277641,1.21416849343679,113.080659952045));
#50620=CARTESIAN_POINT('Ctrl Pts',(18.506090684748,1.21417293573454,113.080628500922));
#50621=CARTESIAN_POINT('Ctrl Pts',(18.5064074300013,1.21417494759492,113.080608862259));
#50622=CARTESIAN_POINT('Ctrl Pts',(18.508281420334,1.21418258364059,113.080490957723));
#50623=CARTESIAN_POINT('Ctrl Pts',(18.5098382130404,1.21417149237957,113.080386007052));
#50624=CARTESIAN_POINT('Ctrl Pts',(18.5113942828676,1.21414296988457,113.080274071063));
#50625=CARTESIAN_POINT('',(18.4283983699428,-1.10353994944975,113.19629633455));
#50626=CARTESIAN_POINT('Ctrl Pts',(18.4283983699428,-1.10353994944975,113.19629633455));
#50627=CARTESIAN_POINT('Ctrl Pts',(18.4105198342568,-1.10089569222145,113.188995676694));
#50628=CARTESIAN_POINT('Ctrl Pts',(18.3941523472385,-1.0974343046632,113.178993223828));
#50629=CARTESIAN_POINT('Ctrl Pts',(18.3704482929768,-1.0926857775768,113.157487700559));
#50630=CARTESIAN_POINT('Ctrl Pts',(18.3621213729005,-1.09112416856474,113.147761481668));
#50631=CARTESIAN_POINT('Ctrl Pts',(18.3449405301417,-1.08954139537506,113.121843290511));
#50632=CARTESIAN_POINT('Ctrl Pts',(18.3377217530226,-1.09048349674533,113.105395217439));
#50633=CARTESIAN_POINT('Ctrl Pts',(18.3272950132282,-1.09831932583815,113.070458177645));
#50634=CARTESIAN_POINT('Ctrl Pts',(18.3245022186406,-1.105373859452,113.052740657108));
#50635=CARTESIAN_POINT('Ctrl Pts',(18.3225000351569,-1.12537512884119,113.019809315101));
#50636=CARTESIAN_POINT('Ctrl Pts',(18.3233523412292,-1.13826827821126,113.004880872036));
#50637=CARTESIAN_POINT('Ctrl Pts',(18.3289022498025,-1.16639544953706,112.981146943516));
#50638=CARTESIAN_POINT('Ctrl Pts',(18.3332624135526,-1.18111489654657,112.972087482887));
#50639=CARTESIAN_POINT('Ctrl Pts',(18.3462969200968,-1.21017577871147,112.95892257907));
#50640=CARTESIAN_POINT('Ctrl Pts',(18.354504490354,-1.22399099626671,112.954742637065));
#50641=CARTESIAN_POINT('Ctrl Pts',(18.3751075959529,-1.24919519347668,112.949602689716));
#50642=CARTESIAN_POINT('Ctrl Pts',(18.3870279922863,-1.26018142477218,112.948629677876));
#50643=CARTESIAN_POINT('Ctrl Pts',(18.4129303458512,-1.27763043969617,112.948272440024));
#50644=CARTESIAN_POINT('Ctrl Pts',(18.4264110510245,-1.28422160833404,112.948763783935));
#50645=CARTESIAN_POINT('Ctrl Pts',(18.4512911255684,-1.29245398632846,112.949998556834));
#50646=CARTESIAN_POINT('Ctrl Pts',(18.4623104342892,-1.29489482010847,112.950651159398));
#50647=CARTESIAN_POINT('Ctrl Pts',(18.4780470056916,-1.29677491735672,112.951605478321));
#50648=CARTESIAN_POINT('Ctrl Pts',(18.4826341413343,-1.29713514230962,112.9518872744));
#50649=CARTESIAN_POINT('Ctrl Pts',(18.4880284340617,-1.29734074235437,112.952220771697));
#50650=CARTESIAN_POINT('Ctrl Pts',(18.488827627531,-1.2973655996001,112.952270241262));
#50651=CARTESIAN_POINT('Ctrl Pts',(18.4898693403749,-1.29739070377487,112.952334798159));
#50652=CARTESIAN_POINT('Ctrl Pts',(18.4901116962636,-1.29739602991256,112.952349822748));
#50653=CARTESIAN_POINT('Ctrl Pts',(18.4905041039374,-1.29740382086684,112.952374158247));
#50654=CARTESIAN_POINT('Ctrl Pts',(18.4906541429139,-1.29740660272727,112.952383465081));
#50655=CARTESIAN_POINT('Ctrl Pts',(18.4909280661229,-1.2974113217336,112.952400460104));
#50656=CARTESIAN_POINT('Ctrl Pts',(18.4910519467619,-1.29741332159137,112.952408147421));
#50657=CARTESIAN_POINT('Ctrl Pts',(18.4913236721632,-1.29741741357458,112.952425012176));
#50658=CARTESIAN_POINT('Ctrl Pts',(18.4914715201352,-1.29741944881729,112.952434190402));
#50659=CARTESIAN_POINT('Ctrl Pts',(18.4918604345446,-1.2974242994241,112.952458338957));
#50660=CARTESIAN_POINT('Ctrl Pts',(18.4921015111322,-1.29742679784955,112.952473313199));
#50661=CARTESIAN_POINT('Ctrl Pts',(18.4932714054423,-1.29743645539092,112.952546005746));
#50662=CARTESIAN_POINT('Ctrl Pts',(18.4942003175021,-1.29743657969559,112.952603802859));
#50663=CARTESIAN_POINT('Ctrl Pts',(18.5075944890952,-1.29732965474523,112.953438376998));
#50664=CARTESIAN_POINT('Ctrl Pts',(18.5200262878613,-1.29587261084622,112.954217675423));
#50665=CARTESIAN_POINT('Ctrl Pts',(18.5512344998855,-1.28871955431818,112.956380272165));
#50666=CARTESIAN_POINT('Ctrl Pts',(18.5693512045022,-1.28113646088861,112.957809120227));
#50667=CARTESIAN_POINT('Ctrl Pts',(18.6029398590356,-1.25971666804792,112.96256925626));
#50668=CARTESIAN_POINT('Ctrl Pts',(18.6176809713591,-1.24594235305202,112.965938249525));
#50669=CARTESIAN_POINT('Ctrl Pts',(18.6422007479794,-1.21409417011734,112.977393937126));
#50670=CARTESIAN_POINT('Ctrl Pts',(18.6512073945201,-1.19667462941293,112.985433472284));
#50671=CARTESIAN_POINT('Ctrl Pts',(18.6635070263108,-1.16275079443269,113.007644142204));
#50672=CARTESIAN_POINT('Ctrl Pts',(18.6667151219446,-1.14676806040784,113.021491299409));
#50673=CARTESIAN_POINT('Ctrl Pts',(18.6681181165073,-1.12186304344204,113.05156803892));
#50674=CARTESIAN_POINT('Ctrl Pts',(18.6669824740447,-1.11233764280274,113.067026820135));
#50675=CARTESIAN_POINT('Ctrl Pts',(18.6608198607348,-1.0995005522286,113.097149717965));
#50676=CARTESIAN_POINT('Ctrl Pts',(18.6563998349178,-1.09560335823169,113.111344641313));
#50677=CARTESIAN_POINT('Ctrl Pts',(18.6435144213581,-1.09173897964326,113.138488335518));
#50678=CARTESIAN_POINT('Ctrl Pts',(18.6354331643911,-1.09172221268073,113.150854236727));
#50679=CARTESIAN_POINT('Ctrl Pts',(18.6166910806198,-1.09379506873728,113.171324492591));
#50680=CARTESIAN_POINT('Ctrl Pts',(18.6068447744918,-1.09554575910708,113.179430674276));
#50681=CARTESIAN_POINT('Ctrl Pts',(18.5825339836664,-1.09986755155098,113.194519964973));
#50682=CARTESIAN_POINT('Ctrl Pts',(18.5678269514339,-1.10245959900021,113.200594508659));
#50683=CARTESIAN_POINT('Ctrl Pts',(18.5399706841515,-1.10605222763602,113.20788137288));
#50684=CARTESIAN_POINT('Ctrl Pts',(18.5271604037061,-1.10726480039516,113.209790754062));
#50685=CARTESIAN_POINT('Ctrl Pts',(18.5080211320997,-1.10820521807391,113.210786846784));
#50686=CARTESIAN_POINT('Ctrl Pts',(18.5017820858503,-1.10837943502796,113.210822647527));
#50687=CARTESIAN_POINT('Ctrl Pts',(18.4945234270871,-1.1084222163849,113.210536072413));
#50688=CARTESIAN_POINT('Ctrl Pts',(18.4934948042869,-1.10842454994123,113.210487758034));
#50689=CARTESIAN_POINT('Ctrl Pts',(18.4921729528856,-1.10842274722134,113.210415775184));
#50690=CARTESIAN_POINT('Ctrl Pts',(18.4918793902317,-1.10842204234513,113.210399161215));
#50691=CARTESIAN_POINT('Ctrl Pts',(18.4914080950982,-1.10842042156096,113.210371480633));
#50692=CARTESIAN_POINT('Ctrl Pts',(18.491230346989,-1.10841969856969,113.210360810743));
#50693=CARTESIAN_POINT('Ctrl Pts',(18.4908911653357,-1.10841810568575,113.210340010881));
#50694=CARTESIAN_POINT('Ctrl Pts',(18.4907297304023,-1.10841725535653,113.210329921146));
#50695=CARTESIAN_POINT('Ctrl Pts',(18.4903662148411,-1.10841513294104,113.210306773437));
#50696=CARTESIAN_POINT('Ctrl Pts',(18.4901641385227,-1.1084138085915,113.210293608004));
#50697=CARTESIAN_POINT('Ctrl Pts',(18.4896414017413,-1.10841000877977,113.210258780781));
#50698=CARTESIAN_POINT('Ctrl Pts',(18.489320764701,-1.10840731400558,113.210236668325));
#50699=CARTESIAN_POINT('Ctrl Pts',(18.4874654483094,-1.10838961412012,113.210104375723));
#50700=CARTESIAN_POINT('Ctrl Pts',(18.4859319332317,-1.10836663760827,113.20997783395));
#50701=CARTESIAN_POINT('Ctrl Pts',(18.4650966690796,-1.10794123351876,113.208024364095));
#50702=CARTESIAN_POINT('Ctrl Pts',(18.4461433726562,-1.10616445698858,113.203542464532));
#50703=CARTESIAN_POINT('Ctrl Pts',(18.4283983699427,-1.10353994944975,113.19629633455));
#50704=CARTESIAN_POINT('',(18.3123644474208,1.23076923076922,111.6));
#50705=CARTESIAN_POINT('',(18.3,1.3,112.2));
#50706=CARTESIAN_POINT('Ctrl Pts',(18.3123644474208,1.23076923076924,111.6));
#50707=CARTESIAN_POINT('Ctrl Pts',(18.2984337402964,1.26852550530057,111.763610522969));
#50708=CARTESIAN_POINT('Ctrl Pts',(18.3000000038754,1.29968079467276,111.965095195088));
#50709=CARTESIAN_POINT('Ctrl Pts',(18.299999999995,1.29999918730283,112.197626492492));
#50710=CARTESIAN_POINT('Ctrl Pts',(18.3,1.3,112.198813368143));
#50711=CARTESIAN_POINT('Ctrl Pts',(18.3,1.3,112.2));
#50712=CARTESIAN_POINT('',(18.6876355525792,1.23076923076922,111.6));
#50713=CARTESIAN_POINT('Ctrl Pts',(18.6876355525792,1.23076923076922,111.6));
#50714=CARTESIAN_POINT('Ctrl Pts',(18.6863212589794,1.23473208763278,111.6));
#50715=CARTESIAN_POINT('Ctrl Pts',(18.6849243200251,1.23859136984675,111.6));
#50716=CARTESIAN_POINT('Ctrl Pts',(18.6737631989001,1.26715167689378,111.6));
#50717=CARTESIAN_POINT('Ctrl Pts',(18.6568893055075,1.29433425576249,111.6));
#50718=CARTESIAN_POINT('Ctrl Pts',(18.6213508157909,1.3318682066872,111.6));
#50719=CARTESIAN_POINT('Ctrl Pts',(18.5969013940152,1.3493098388476,111.6));
#50720=CARTESIAN_POINT('Ctrl Pts',(18.5520128528442,1.3688365799757,111.6));
#50721=CARTESIAN_POINT('Ctrl Pts',(18.5239242084953,1.37477270848677,111.6));
#50722=CARTESIAN_POINT('Ctrl Pts',(18.5,1.37477270848677,111.6));
#50723=CARTESIAN_POINT('Ctrl Pts',(18.4760757915047,1.37477270848677,111.6));
#50724=CARTESIAN_POINT('Ctrl Pts',(18.4479871471558,1.3688365799757,111.6));
#50725=CARTESIAN_POINT('Ctrl Pts',(18.4030986059848,1.3493098388476,111.6));
#50726=CARTESIAN_POINT('Ctrl Pts',(18.3786491842091,1.3318682066872,111.6));
#50727=CARTESIAN_POINT('Ctrl Pts',(18.3431106944925,1.29433425576249,111.6));
#50728=CARTESIAN_POINT('Ctrl Pts',(18.3262368010999,1.26715167689378,111.6));
#50729=CARTESIAN_POINT('Ctrl Pts',(18.3150756799749,1.23859136984675,111.6));
#50730=CARTESIAN_POINT('Ctrl Pts',(18.3136787410206,1.23473208763278,111.6));
#50731=CARTESIAN_POINT('Ctrl Pts',(18.3123644474208,1.23076923076922,111.6));
#50732=CARTESIAN_POINT('',(18.7,1.3,112.2));
#50733=CARTESIAN_POINT('Ctrl Pts',(18.7,1.3,112.2));
#50734=CARTESIAN_POINT('Ctrl Pts',(18.7,1.3,112.198813368143));
#50735=CARTESIAN_POINT('Ctrl Pts',(18.700000000005,1.29999918730283,112.197626492492));
#50736=CARTESIAN_POINT('Ctrl Pts',(18.6999999961246,1.29968079467278,111.965095195094));
#50737=CARTESIAN_POINT('Ctrl Pts',(18.7015662597039,1.26852550530162,111.763610522974));
#50738=CARTESIAN_POINT('Ctrl Pts',(18.6876355525792,1.23076923076923,111.6));
#50739=CARTESIAN_POINT('',(18.6999907542242,1.29807692307696,112.3));
#50740=CARTESIAN_POINT('Ctrl Pts',(18.6999907542242,1.29807692307696,112.3));
#50741=CARTESIAN_POINT('Ctrl Pts',(18.7000026383082,1.29931281067831,112.267866922365));
#50742=CARTESIAN_POINT('Ctrl Pts',(18.6999999994485,1.29995353020451,112.235718199897));
#50743=CARTESIAN_POINT('Ctrl Pts',(18.700000000005,1.29999918730283,112.202373507508));
#50744=CARTESIAN_POINT('Ctrl Pts',(18.7,1.3,112.201186631857));
#50745=CARTESIAN_POINT('Ctrl Pts',(18.7,1.3,112.2));
#50746=CARTESIAN_POINT('',(18.3000092457758,1.29807692307696,112.3));
#50747=CARTESIAN_POINT('Ctrl Pts',(18.3000092457758,1.29807692307696,112.3));
#50748=CARTESIAN_POINT('Ctrl Pts',(18.3002426875627,1.32242567789215,112.3));
#50749=CARTESIAN_POINT('Ctrl Pts',(18.3060316768999,1.35067447040255,112.3));
#50750=CARTESIAN_POINT('Ctrl Pts',(18.3247081897855,1.39582998875735,112.3));
#50751=CARTESIAN_POINT('Ctrl Pts',(18.3411747406685,1.42052008010624,112.3));
#50752=CARTESIAN_POINT('Ctrl Pts',(18.3760974271551,1.45549178160028,112.3));
#50753=CARTESIAN_POINT('Ctrl Pts',(18.4007210413769,1.47197246341128,112.3));
#50754=CARTESIAN_POINT('Ctrl Pts',(18.4463107520171,1.49088031549837,112.3));
#50755=CARTESIAN_POINT('Ctrl Pts',(18.4753365162084,1.49666295470959,112.3));
#50756=CARTESIAN_POINT('Ctrl Pts',(18.5,1.49666295470959,112.3));
#50757=CARTESIAN_POINT('Ctrl Pts',(18.5246634837916,1.49666295470959,112.3));
#50758=CARTESIAN_POINT('Ctrl Pts',(18.5536892479829,1.49088031549837,112.3));
#50759=CARTESIAN_POINT('Ctrl Pts',(18.5992789586231,1.47197246341128,112.3));
#50760=CARTESIAN_POINT('Ctrl Pts',(18.6239025728449,1.45549178160028,112.3));
#50761=CARTESIAN_POINT('Ctrl Pts',(18.6588252593315,1.42052008010624,112.3));
#50762=CARTESIAN_POINT('Ctrl Pts',(18.6752918102145,1.39582998875735,112.3));
#50763=CARTESIAN_POINT('Ctrl Pts',(18.6939683231001,1.35067447040255,112.3));
#50764=CARTESIAN_POINT('Ctrl Pts',(18.6997573124373,1.32242567789215,112.3));
#50765=CARTESIAN_POINT('Ctrl Pts',(18.6999907542242,1.29807692307696,112.3));
#50766=CARTESIAN_POINT('Ctrl Pts',(18.3,1.3,112.2));
#50767=CARTESIAN_POINT('Ctrl Pts',(18.3,1.3,112.201186631857));
#50768=CARTESIAN_POINT('Ctrl Pts',(18.299999999995,1.29999918730283,112.202373507508));
#50769=CARTESIAN_POINT('Ctrl Pts',(18.3000000005515,1.29995353020451,112.235718199897));
#50770=CARTESIAN_POINT('Ctrl Pts',(18.2999973616918,1.2993128106783,112.267866922365));
#50771=CARTESIAN_POINT('Ctrl Pts',(18.3000092457758,1.29807692307696,112.3));
#50772=CARTESIAN_POINT('Origin',(18.5,1.3,112.3));
#50773=CARTESIAN_POINT('Origin',(18.5,1.3,112.3));
#50774=CARTESIAN_POINT('Origin',(18.5,1.3,111.6));
#50775=CARTESIAN_POINT('Origin',(18.5,1.3,111.6));
#50776=CARTESIAN_POINT('Origin',(18.5,1.3,111.6));
#50777=CARTESIAN_POINT('Origin',(18.5,1.3,112.9));
#50778=CARTESIAN_POINT('Origin',(18.5,1.3,112.9));
#50779=CARTESIAN_POINT('Origin',(18.5,0.,128.8));
#50780=CARTESIAN_POINT('',(18.5,-1.34711147906207E-16,127.7));
#50781=CARTESIAN_POINT('Origin',(18.5,-1.59204083889153E-16,127.5));
#50782=CARTESIAN_POINT('Origin',(18.5,0.,128.8));
#50783=CARTESIAN_POINT('',(18.7,1.3,128.8));
#50784=CARTESIAN_POINT('',(18.3,1.3,128.8));
#50785=CARTESIAN_POINT('Origin',(18.5,1.3,128.8));
#50786=CARTESIAN_POINT('',(18.3235897901759,1.20576923076922,128.1));
#50787=CARTESIAN_POINT('Ctrl Pts',(18.3235897901759,1.20576923076922,128.1));
#50788=CARTESIAN_POINT('Ctrl Pts',(18.2973822762268,1.25483253644383,128.282235135363));
#50789=CARTESIAN_POINT('Ctrl Pts',(18.3000000041203,1.29963250090516,128.518892224432));
#50790=CARTESIAN_POINT('Ctrl Pts',(18.2999999999958,1.29999925015416,128.797720020479));
#50791=CARTESIAN_POINT('Ctrl Pts',(18.3,1.3,128.798860078224));
#50792=CARTESIAN_POINT('Ctrl Pts',(18.3,1.3,128.8));
#50793=CARTESIAN_POINT('',(18.5002243000221,1.32664977393096,128.1));
#50794=CARTESIAN_POINT('Ctrl Pts',(18.5002243000221,1.32664977393096,128.1));
#50795=CARTESIAN_POINT('Ctrl Pts',(18.5001494926749,1.32664986879001,128.1));
#50796=CARTESIAN_POINT('Ctrl Pts',(18.5000747258889,1.32664991614213,128.1));
#50797=CARTESIAN_POINT('Ctrl Pts',(18.5,1.32664991614213,128.1));
#50798=CARTESIAN_POINT('Ctrl Pts',(18.4763894791635,1.32664991614213,128.1));
#50799=CARTESIAN_POINT('Ctrl Pts',(18.4486985736677,1.32065396814081,128.1));
#50800=CARTESIAN_POINT('Ctrl Pts',(18.4041135913171,1.30087556631979,128.1));
#50801=CARTESIAN_POINT('Ctrl Pts',(18.3797528378326,1.28303070674698,128.1));
#50802=CARTESIAN_POINT('Ctrl Pts',(18.3476245045884,1.24833850134275,128.1));
#50803=CARTESIAN_POINT('Ctrl Pts',(18.3333992207159,1.22700388737273,128.1));
#50804=CARTESIAN_POINT('Ctrl Pts',(18.3235897901759,1.20576923076922,128.1));
#50805=CARTESIAN_POINT('',(18.4886057170625,1.21414296988327,127.919725928942));
#50806=CARTESIAN_POINT('Ctrl Pts',(18.4886057170625,1.21414296988326,127.919725928942));
#50807=CARTESIAN_POINT('Ctrl Pts',(18.4911877797212,1.24297666476934,127.9592445997));
#50808=CARTESIAN_POINT('Ctrl Pts',(18.4937851821151,1.26920627380217,127.999392649018));
#50809=CARTESIAN_POINT('Ctrl Pts',(18.4975804224297,1.30412024852119,128.058540778958));
#50810=CARTESIAN_POINT('Ctrl Pts',(18.4988856330623,1.31555196810735,128.078964066341));
#50811=CARTESIAN_POINT('Ctrl Pts',(18.5002243000221,1.32664977393097,128.1));
#50812=CARTESIAN_POINT('',(18.6702841632836,1.12955615107723,127.964633341575));
#50813=CARTESIAN_POINT('Ctrl Pts',(18.6702841630468,1.12955615106615,127.964633341765));
#50814=CARTESIAN_POINT('Ctrl Pts',(18.6653387332645,1.13522043042002,127.958790838693));
#50815=CARTESIAN_POINT('Ctrl Pts',(18.6597721606308,1.14104363370426,127.953610539743));
#50816=CARTESIAN_POINT('Ctrl Pts',(18.6402703998699,1.15942016474004,127.939130439405));
#50817=CARTESIAN_POINT('Ctrl Pts',(18.6245076173094,1.17154609064284,127.932283746225));
#50818=CARTESIAN_POINT('Ctrl Pts',(18.5913880187093,1.19100127211283,127.923348439596));
#50819=CARTESIAN_POINT('Ctrl Pts',(18.5745475659151,1.19865280082519,127.920838868829));
#50820=CARTESIAN_POINT('Ctrl Pts',(18.5439935651917,1.2082106549485,127.918559765759));
#50821=CARTESIAN_POINT('Ctrl Pts',(18.5307553501655,1.2110925974478,127.918240112273));
#50822=CARTESIAN_POINT('Ctrl Pts',(18.5114409726006,1.21339552395061,127.918551626728));
#50823=CARTESIAN_POINT('Ctrl Pts',(18.5055323311222,1.21385044304153,127.918750721917));
#50824=CARTESIAN_POINT('Ctrl Pts',(18.4986318935235,1.21408801960182,127.919100745897));
#50825=CARTESIAN_POINT('Ctrl Pts',(18.4976486652827,1.21411493333287,127.919153408432));
#50826=CARTESIAN_POINT('Ctrl Pts',(18.4963815755996,1.21414066956251,127.919224867006));
#50827=CARTESIAN_POINT('Ctrl Pts',(18.4960977244373,1.21414585629502,127.919241107366));
#50828=CARTESIAN_POINT('Ctrl Pts',(18.4956400831649,1.21415328554028,127.919267665666));
#50829=CARTESIAN_POINT('Ctrl Pts',(18.495466291215,1.21415588987324,127.91927783845));
#50830=CARTESIAN_POINT('Ctrl Pts',(18.4951351880664,1.21416043816795,127.919297385324));
#50831=CARTESIAN_POINT('Ctrl Pts',(18.4949778766776,1.21416242132666,127.919306743687));
#50832=CARTESIAN_POINT('Ctrl Pts',(18.4946224550266,1.2141665002405,127.919328048841));
#50833=CARTESIAN_POINT('Ctrl Pts',(18.4944243463601,1.21416849177246,127.919340037381));
#50834=CARTESIAN_POINT('Ctrl Pts',(18.4939094760844,1.21417293460233,127.919371489148));
#50835=CARTESIAN_POINT('Ctrl Pts',(18.4935927224993,1.21417494675346,127.919391128233));
#50836=CARTESIAN_POINT('Ctrl Pts',(18.4917186757302,1.21418258432441,127.9195090358));
#50837=CARTESIAN_POINT('Ctrl Pts',(18.490161834936,1.21417149325911,127.919613989496));
#50838=CARTESIAN_POINT('Ctrl Pts',(18.4886057170625,1.21414296988326,127.919725928942));
#50839=CARTESIAN_POINT('',(18.6933911448853,1.24901112788112,128.285080457724));
#50840=CARTESIAN_POINT('Ctrl Pts',(18.6933911448858,1.24901112788106,128.285080457724));
#50841=CARTESIAN_POINT('Ctrl Pts',(18.6941695295676,1.2455347549892,128.284393845319));
#50842=CARTESIAN_POINT('Ctrl Pts',(18.6948689918491,1.2420448951124,128.28362015538));
#50843=CARTESIAN_POINT('Ctrl Pts',(18.6991384438423,1.2181470596441,128.277703499066));
#50844=CARTESIAN_POINT('Ctrl Pts',(18.700090555879,1.19846217194705,128.269752590558));
#50845=CARTESIAN_POINT('Ctrl Pts',(18.6998883984898,1.16039199645397,128.246791255634));
#50846=CARTESIAN_POINT('Ctrl Pts',(18.6985769622911,1.14211768289233,128.231171889393));
#50847=CARTESIAN_POINT('Ctrl Pts',(18.6971943128989,1.1116295024956,128.1930989791));
#50848=CARTESIAN_POINT('Ctrl Pts',(18.6972376067016,1.10002920430251,128.171906869082));
#50849=CARTESIAN_POINT('Ctrl Pts',(18.6986757815866,1.08449168880853,128.12634150471));
#50850=CARTESIAN_POINT('Ctrl Pts',(18.6999332936667,1.08103423817092,128.102989944245));
#50851=CARTESIAN_POINT('Ctrl Pts',(18.7000503625628,1.08205735198823,128.062145569422));
#50852=CARTESIAN_POINT('Ctrl Pts',(18.6992937255094,1.08525274687609,128.044011007997));
#50853=CARTESIAN_POINT('Ctrl Pts',(18.69387406073,1.09673110860034,128.01092941677));
#50854=CARTESIAN_POINT('Ctrl Pts',(18.6896083372694,1.104353449732,127.996558781634));
#50855=CARTESIAN_POINT('Ctrl Pts',(18.6793930756325,1.11858988928783,127.976739577122));
#50856=CARTESIAN_POINT('Ctrl Pts',(18.6751379969018,1.12399678168825,127.97036763392));
#50857=CARTESIAN_POINT('Ctrl Pts',(18.6702841630468,1.12955615106615,127.964633341765));
#50858=CARTESIAN_POINT('Ctrl Pts',(18.7,1.3,128.8));
#50859=CARTESIAN_POINT('Ctrl Pts',(18.7,1.3,128.798860078224));
#50860=CARTESIAN_POINT('Ctrl Pts',(18.7000000000042,1.29999925015416,128.797720020479));
#50861=CARTESIAN_POINT('Ctrl Pts',(18.699999997155,1.29974590119044,128.605106856646));
#50862=CARTESIAN_POINT('Ctrl Pts',(18.7011229833964,1.27833652849495,128.433154157275));
#50863=CARTESIAN_POINT('Ctrl Pts',(18.6933911448853,1.24901112788118,128.285080457724));
#50864=CARTESIAN_POINT('',(18.3892924448916,-1.25128032625762,128.035075233373));
#50865=CARTESIAN_POINT('Ctrl Pts',(18.3892924448916,-1.25128032625762,128.035075233373));
#50866=CARTESIAN_POINT('Ctrl Pts',(18.3798994606449,-1.24247387220421,128.03263906063));
#50867=CARTESIAN_POINT('Ctrl Pts',(18.3716813533086,-1.23279082229575,128.029561362241));
#50868=CARTESIAN_POINT('Ctrl Pts',(18.3585843738093,-1.21376562057004,128.022036324831));
#50869=CARTESIAN_POINT('Ctrl Pts',(18.3534816661773,-1.2047112654056,128.017901894435));
#50870=CARTESIAN_POINT('Ctrl Pts',(18.3416272087126,-1.17934898870496,128.004113103988));
#50871=CARTESIAN_POINT('Ctrl Pts',(18.3368687162988,-1.1633410963693,127.99285169318));
#50872=CARTESIAN_POINT('Ctrl Pts',(18.3319858487178,-1.13523495824815,127.96592156058));
#50873=CARTESIAN_POINT('Ctrl Pts',(18.3316753585454,-1.12317339172176,127.950591366736));
#50874=CARTESIAN_POINT('Ctrl Pts',(18.3352116622682,-1.10601113755093,127.919878737263));
#50875=CARTESIAN_POINT('Ctrl Pts',(18.3384075916268,-1.10019403805833,127.905051434488));
#50876=CARTESIAN_POINT('Ctrl Pts',(18.3486564892805,-1.09329953675059,127.87665371864));
#50877=CARTESIAN_POINT('Ctrl Pts',(18.3552149615871,-1.09196650404974,127.86356771344));
#50878=CARTESIAN_POINT('Ctrl Pts',(18.3728912616988,-1.09222750541447,127.838810790113));
#50879=CARTESIAN_POINT('Ctrl Pts',(18.383771728885,-1.09393068606538,127.8279088649));
#50880=CARTESIAN_POINT('Ctrl Pts',(18.409424692351,-1.09840208445071,127.809605483562));
#50881=CARTESIAN_POINT('Ctrl Pts',(18.4238896729194,-1.10110524006805,127.802632548698));
#50882=CARTESIAN_POINT('Ctrl Pts',(18.4522867719007,-1.10518160358501,127.793659605297));
#50883=CARTESIAN_POINT('Ctrl Pts',(18.4658454196017,-1.10668775670786,127.791095337941));
#50884=CARTESIAN_POINT('Ctrl Pts',(18.4876523176408,-1.10806135716137,127.789283776043));
#50885=CARTESIAN_POINT('Ctrl Pts',(18.4957622801494,-1.10835349387855,127.789104107661));
#50886=CARTESIAN_POINT('Ctrl Pts',(18.5050575455568,-1.10842097725468,127.789444840517));
#50887=CARTESIAN_POINT('Ctrl Pts',(18.5062500731142,-1.10842463446296,127.789498891965));
#50888=CARTESIAN_POINT('Ctrl Pts',(18.5077522181175,-1.10842290541232,127.789580034198));
#50889=CARTESIAN_POINT('Ctrl Pts',(18.5080615324343,-1.10842221190459,127.78959743825));
#50890=CARTESIAN_POINT('Ctrl Pts',(18.50855223089,-1.10842057420063,127.789626155808));
#50891=CARTESIAN_POINT('Ctrl Pts',(18.5087335224116,-1.10841985313119,127.789637004744));
#50892=CARTESIAN_POINT('Ctrl Pts',(18.5090592733913,-1.10841834823437,127.789656929655));
#50893=CARTESIAN_POINT('Ctrl Pts',(18.5092037035598,-1.10841760733907,127.789665915658));
#50894=CARTESIAN_POINT('Ctrl Pts',(18.509514596913,-1.10841585336197,127.789685586428));
#50895=CARTESIAN_POINT('Ctrl Pts',(18.509681076526,-1.10841481622478,127.789696321608));
#50896=CARTESIAN_POINT('Ctrl Pts',(18.5101596687195,-1.10841155216991,127.789727764983));
#50897=CARTESIAN_POINT('Ctrl Pts',(18.510471882263,-1.10840907831999,127.789748987171));
#50898=CARTESIAN_POINT('Ctrl Pts',(18.5118942490537,-1.10839623268546,127.789848916666));
#50899=CARTESIAN_POINT('Ctrl Pts',(18.5130045279313,-1.10838184132914,127.789935912113));
#50900=CARTESIAN_POINT('Ctrl Pts',(18.5289010892121,-1.10811313058816,127.791310872672));
#50901=CARTESIAN_POINT('Ctrl Pts',(18.5435288883242,-1.10706679477448,127.794167098735));
#50902=CARTESIAN_POINT('Ctrl Pts',(18.5780645770096,-1.10298841376075,127.805135758393));
#50903=CARTESIAN_POINT('Ctrl Pts',(18.5963905684292,-1.09938262181171,127.814741468509));
#50904=CARTESIAN_POINT('Ctrl Pts',(18.6270867645603,-1.09315777119027,127.838998624416));
#50905=CARTESIAN_POINT('Ctrl Pts',(18.6395729240457,-1.09053042151983,127.853385617341));
#50906=CARTESIAN_POINT('Ctrl Pts',(18.6587003172132,-1.08984138593605,127.885720048849));
#50907=CARTESIAN_POINT('Ctrl Pts',(18.6651532160224,-1.09158743291629,127.90246539444));
#50908=CARTESIAN_POINT('Ctrl Pts',(18.6742126672308,-1.10122999609394,127.937592024301));
#50909=CARTESIAN_POINT('Ctrl Pts',(18.6764218952049,-1.10933821221676,127.95526698208));
#50910=CARTESIAN_POINT('Ctrl Pts',(18.6772210972485,-1.13106051535397,127.987174545981));
#50911=CARTESIAN_POINT('Ctrl Pts',(18.6758404085021,-1.14447798380644,128.001238995918));
#50912=CARTESIAN_POINT('Ctrl Pts',(18.6691623998671,-1.17314306545758,128.023265178206));
#50913=CARTESIAN_POINT('Ctrl Pts',(18.6642428497083,-1.18785848703717,128.031478436654));
#50914=CARTESIAN_POINT('Ctrl Pts',(18.6500295363492,-1.21660724198031,128.043222559086));
#50915=CARTESIAN_POINT('Ctrl Pts',(18.6412150739195,-1.23011383168726,128.046802507509));
#50916=CARTESIAN_POINT('Ctrl Pts',(18.6195527785074,-1.25435939432101,128.050987824865));
#50917=CARTESIAN_POINT('Ctrl Pts',(18.6071944358135,-1.26474856820655,128.051626762945));
#50918=CARTESIAN_POINT('Ctrl Pts',(18.5809477583168,-1.28077826412714,128.05155359561));
#50919=CARTESIAN_POINT('Ctrl Pts',(18.5675600416982,-1.28666191306148,128.050974310672));
#50920=CARTESIAN_POINT('Ctrl Pts',(18.5435683232137,-1.29363459637126,128.049701976543));
#50921=CARTESIAN_POINT('Ctrl Pts',(18.5333148146624,-1.29560082132902,128.049086890045));
#50922=CARTESIAN_POINT('Ctrl Pts',(18.5190012477797,-1.29700506719052,128.048213240759));
#50923=CARTESIAN_POINT('Ctrl Pts',(18.5150412649157,-1.29725470226466,128.047969337274));
#50924=CARTESIAN_POINT('Ctrl Pts',(18.5106959483058,-1.29737719199358,128.047700235014));
#50925=CARTESIAN_POINT('Ctrl Pts',(18.5103183510609,-1.29738658894726,128.047676837662));
#50926=CARTESIAN_POINT('Ctrl Pts',(18.5097606195382,-1.2973986209018,128.047642259385));
#50927=CARTESIAN_POINT('Ctrl Pts',(18.5095806912436,-1.29740221955525,128.047631101249));
#50928=CARTESIAN_POINT('Ctrl Pts',(18.5092748392951,-1.29740785409831,128.047612129049));
#50929=CARTESIAN_POINT('Ctrl Pts',(18.5091489697301,-1.29741003450508,128.047604319845));
#50930=CARTESIAN_POINT('Ctrl Pts',(18.5088930397262,-1.29741418546983,128.047588438508));
#50931=CARTESIAN_POINT('Ctrl Pts',(18.5087629747962,-1.29741614724726,128.047580366003));
#50932=CARTESIAN_POINT('Ctrl Pts',(18.5084551210459,-1.29742043962893,128.047561255371));
#50933=CARTESIAN_POINT('Ctrl Pts',(18.508277286455,-1.29742264299259,128.047550213079));
#50934=CARTESIAN_POINT('Ctrl Pts',(18.5076554909947,-1.2974293779868,128.047511593851));
#50935=CARTESIAN_POINT('Ctrl Pts',(18.5072112685641,-1.29743246690907,128.047483985686));
#50936=CARTESIAN_POINT('Ctrl Pts',(18.5021353719972,-1.29744801399593,128.047168313941));
#50937=CARTESIAN_POINT('Ctrl Pts',(18.4975003376624,-1.29727471082049,128.04687828474));
#50938=CARTESIAN_POINT('Ctrl Pts',(18.4722386482183,-1.29530419319829,128.045279066271));
#50939=CARTESIAN_POINT('Ctrl Pts',(18.4520327626891,-1.28998020248121,128.044002189889));
#50940=CARTESIAN_POINT('Ctrl Pts',(18.4170565203638,-1.27354147714406,128.040503340081));
#50941=CARTESIAN_POINT('Ctrl Pts',(18.4022413006459,-1.2634206109904,128.038433660112));
#50942=CARTESIAN_POINT('Ctrl Pts',(18.3892924448916,-1.25128032625768,128.035075233373));
#50943=CARTESIAN_POINT('Origin',(18.5,1.30000000000003,128.1));
#50944=CARTESIAN_POINT('',(18.5016832568904,1.49999291649016,128.1));
#50945=CARTESIAN_POINT('',(18.5,1.30000000000001,128.1));
#50946=CARTESIAN_POINT('Origin',(18.5,1.30000000000003,128.1));
#50947=CARTESIAN_POINT('Origin',(18.5,1.3,128.1));
#50948=CARTESIAN_POINT('Origin',(18.5,1.3,128.1));
#50949=CARTESIAN_POINT('Origin',(18.5,1.3,128.1));
#50950=CARTESIAN_POINT('Ctrl Pts',(18.5016832568899,1.49999291649016,128.1));
#50951=CARTESIAN_POINT('Ctrl Pts',(18.5019060534612,1.49999104130443,128.100197947578));
#50952=CARTESIAN_POINT('Ctrl Pts',(18.5021288480507,1.49998879380848,128.100395894012));
#50953=CARTESIAN_POINT('Ctrl Pts',(18.5332913213164,1.49962235392642,128.128082945286));
#50954=CARTESIAN_POINT('Ctrl Pts',(18.5643676714885,1.49207596231939,128.155707919539));
#50955=CARTESIAN_POINT('Ctrl Pts',(18.6158401718151,1.46508561658941,128.202366702973));
#50956=CARTESIAN_POINT('Ctrl Pts',(18.6373473722111,1.44811312339091,128.222225381534));
#50957=CARTESIAN_POINT('Ctrl Pts',(18.6687008379444,1.40953464131882,128.252332431214));
#50958=CARTESIAN_POINT('Ctrl Pts',(18.6801090859612,1.39004658705681,128.263746708316));
#50959=CARTESIAN_POINT('Ctrl Pts',(18.6945636658313,1.35009248507517,128.279386999448));
#50960=CARTESIAN_POINT('Ctrl Pts',(18.69864622317,1.33076612999911,128.284423898441));
#50961=CARTESIAN_POINT('Ctrl Pts',(18.7007458372437,1.29129390710522,128.289049365168));
#50962=CARTESIAN_POINT('Ctrl Pts',(18.6989593474376,1.27195776119289,128.288754201356));
#50963=CARTESIAN_POINT('Ctrl Pts',(18.6941136437467,1.25181280973272,128.285570187084));
#50964=CARTESIAN_POINT('Ctrl Pts',(18.6937594098627,1.25040788726464,128.285332422228));
#50965=CARTESIAN_POINT('Ctrl Pts',(18.6933911448853,1.24901112788109,128.285080457724));
#50966=CARTESIAN_POINT('Ctrl Pts',(18.488182152249,1.29990053410893,112.700349483895));
#50967=CARTESIAN_POINT('Ctrl Pts',(18.3444976430382,1.29869120157713,112.70885515658));
#50968=CARTESIAN_POINT('Ctrl Pts',(18.1626414086569,1.26954424100949,112.72020028386));
#50969=CARTESIAN_POINT('Ctrl Pts',(17.9105741471188,1.1715572059241,112.7372275449));
#50970=CARTESIAN_POINT('Ctrl Pts',(17.7147016928909,1.05680544825268,112.75142581384));
#50971=CARTESIAN_POINT('Ctrl Pts',(17.5092914781924,0.870936460786282,112.768496063499));
#50972=CARTESIAN_POINT('Ctrl Pts',(17.3452643787265,0.645338607702756,112.785608543142));
#50973=CARTESIAN_POINT('Ctrl Pts',(17.1949694671818,0.305633664533222,112.808486356608));
#50974=CARTESIAN_POINT('Ctrl Pts',(17.1504041586296,-0.163958059400556,
112.8371493128));
#50975=CARTESIAN_POINT('Ctrl Pts',(17.3295581344551,-0.704127606930189,
112.871679546659));
#50976=CARTESIAN_POINT('Ctrl Pts',(17.7163063911852,-1.12497913550319,112.906352649458));
#50977=CARTESIAN_POINT('Ctrl Pts',(18.2431925961433,-1.35205912276461,112.941152109412));
#50978=CARTESIAN_POINT('Ctrl Pts',(18.8187741112765,-1.34427642838518,112.976089285723));
#50979=CARTESIAN_POINT('Ctrl Pts',(19.3432395618757,-1.10098396627254,113.011156346434));
#50980=CARTESIAN_POINT('Ctrl Pts',(19.7238494382154,-0.663159822701633,
113.046357078694));
#50981=CARTESIAN_POINT('Ctrl Pts',(19.8931314314799,-0.105956319615994,
113.08168722595));
#50982=CARTESIAN_POINT('Ctrl Pts',(19.8197719071333,0.473908286429459,113.117148366555));
#50983=CARTESIAN_POINT('Ctrl Pts',(19.514861434432,0.975046989864885,113.152737815001));
#50984=CARTESIAN_POINT('Ctrl Pts',(19.0301258646803,1.30913564752012,113.188455340763));
#50985=CARTESIAN_POINT('Ctrl Pts',(18.4491549165285,1.416472562517,113.224299311997));
#50986=CARTESIAN_POINT('Ctrl Pts',(17.8730091730699,1.27666467315962,113.260268611474));
#50987=CARTESIAN_POINT('Ctrl Pts',(17.4026034483492,0.912474225359778,113.296361769111));
#50988=CARTESIAN_POINT('Ctrl Pts',(17.1210280345443,0.386131812194797,113.332577359437));
#50989=CARTESIAN_POINT('Ctrl Pts',(17.0788544181136,-0.211299879373549,
113.368913814958));
#50990=CARTESIAN_POINT('Ctrl Pts',(17.2850565553758,-0.775695991436841,
113.405369493798));
#50991=CARTESIAN_POINT('Ctrl Pts',(17.705146965038,-1.20803167965084,113.441942712263));
#50992=CARTESIAN_POINT('Ctrl Pts',(18.2669652505624,-1.43177932086286,113.478631613973));
#50993=CARTESIAN_POINT('Ctrl Pts',(18.8730309513044,-1.40645905314605,113.51543444437));
#50994=CARTESIAN_POINT('Ctrl Pts',(19.4175618056869,-1.13497091574588,113.55234907248));
#50995=CARTESIAN_POINT('Ctrl Pts',(19.8048480383929,-0.663350581086933,
113.589373656825));
#50996=CARTESIAN_POINT('Ctrl Pts',(19.966197057422,-0.0729778537808475,
113.626505971993));
#50997=CARTESIAN_POINT('Ctrl Pts',(19.8720657245217,0.533549954628291,113.663743893195));
#50998=CARTESIAN_POINT('Ctrl Pts',(19.5374817640394,1.0501311842453,113.701085198819));
#50999=CARTESIAN_POINT('Ctrl Pts',(19.0196808505253,1.38594482959087,113.738527490934));
#51000=CARTESIAN_POINT('Ctrl Pts',(18.5101754020758,1.46526119175664,113.769811704289));
#51001=CARTESIAN_POINT('Ctrl Pts',(18.1090240872925,1.39960741569811,113.794887075397));
#51002=CARTESIAN_POINT('Ctrl Pts',(17.729655069815,1.25220225914757,113.819994103033));
#51003=CARTESIAN_POINT('Ctrl Pts',(17.3289300722954,0.923586877948104,113.851436567131));
#51004=CARTESIAN_POINT('Ctrl Pts',(17.0504721252432,0.365805609893722,113.889258509496));
#51005=CARTESIAN_POINT('Ctrl Pts',(17.0240290762783,-0.258477757917008,
113.927168961164));
#51006=CARTESIAN_POINT('Ctrl Pts',(17.2554238425403,-0.840447617959809,
113.965165177094));
#51007=CARTESIAN_POINT('Ctrl Pts',(17.7053131011304,-1.27808626113464,114.003244380208));
#51008=CARTESIAN_POINT('Ctrl Pts',(18.2959641544648,-1.49425702735341,114.041403784502));
#51009=CARTESIAN_POINT('Ctrl Pts',(18.9246622805112,-1.4502272181577,114.079640512388));
#51010=CARTESIAN_POINT('Ctrl Pts',(19.4816239236303,-1.15267110135651,114.117951609114));
#51011=CARTESIAN_POINT('Ctrl Pts',(19.8691907107327,-0.652639427392253,
114.156334167846));
#51012=CARTESIAN_POINT('Ctrl Pts',(20.0189810591327,-0.03683256961316,114.194785080069));
#51013=CARTESIAN_POINT('Ctrl Pts',(19.9039833865991,0.587522999416328,114.2333013558));
#51014=CARTESIAN_POINT('Ctrl Pts',(19.5434230734537,1.11127572106957,114.271879839515));
#51015=CARTESIAN_POINT('Ctrl Pts',(18.9995399107886,1.44259279852258,114.310517384521));
#51016=CARTESIAN_POINT('Ctrl Pts',(18.3668596633944,1.52297273199859,114.349210799966));
#51017=CARTESIAN_POINT('Ctrl Pts',(17.7556977562459,1.33767203016567,114.387956849117));
#51018=CARTESIAN_POINT('Ctrl Pts',(17.272914349715,0.918370107647551,114.426752263094));
#51019=CARTESIAN_POINT('Ctrl Pts',(17.0031861863323,0.337753138207008,114.46559374694));
#51020=CARTESIAN_POINT('Ctrl Pts',(16.9941242219495,-0.303088855509916,
114.504477951706));
#51021=CARTESIAN_POINT('Ctrl Pts',(17.2478715429229,-0.892350566926149,
114.543401543985));
#51022=CARTESIAN_POINT('Ctrl Pts',(17.720592505509,-1.32694200600498,114.582361077963));
#51023=CARTESIAN_POINT('Ctrl Pts',(18.3301332049521,-1.53077558802408,114.621353247865));
#51024=CARTESIAN_POINT('Ctrl Pts',(18.8635057740616,-1.47820468577621,114.653870882415));
#51025=CARTESIAN_POINT('Ctrl Pts',(19.2496685905278,-1.30821665552171,114.679897931973));
#51026=CARTESIAN_POINT('Ctrl Pts',(19.5923918636366,-1.06191387672613,114.705932982827));
#51027=CARTESIAN_POINT('Ctrl Pts',(19.9091081456583,-0.628734129737697,
114.738490494062));
#51028=CARTESIAN_POINT('Ctrl Pts',(20.0436482399265,0.00136013336455928,
114.777578396996));
#51029=CARTESIAN_POINT('Ctrl Pts',(19.9090928165798,0.631655323772199,114.816681421648));
#51030=CARTESIAN_POINT('Ctrl Pts',(19.5286868815429,1.1521949790643,114.855796201813));
#51031=CARTESIAN_POINT('Ctrl Pts',(18.9687372623033,1.47200625927751,114.894919129408));
#51032=CARTESIAN_POINT('Ctrl Pts',(18.3269247722238,1.53523233022917,114.934046750203));
#51033=CARTESIAN_POINT('Ctrl Pts',(17.7152334288248,1.33076841613399,114.973175454517));
#51034=CARTESIAN_POINT('Ctrl Pts',(17.2404725580255,0.894349558877001,115.012301840373));
#51035=CARTESIAN_POINT('Ctrl Pts',(16.9853446354984,0.302108848816737,115.051422158546));
#51036=CARTESIAN_POINT('Ctrl Pts',(16.9934993376988,-0.27079628228924,115.086187634404));
#51037=CARTESIAN_POINT('Ctrl Pts',(17.1704122775008,-0.733300276011371,
115.116598560424));
#51038=CARTESIAN_POINT('Ctrl Pts',(17.3615831320585,-0.98758491633179,115.136144037193));
#51039=CARTESIAN_POINT('Ctrl Pts',(17.5154254407977,-1.13081668225498,115.149171118788));
#51040=CARTESIAN_POINT('Ctrl Pts',(17.5970581795022,-1.19692836165928,115.155684477762));
#51041=CARTESIAN_POINT('Ctrl Pts',(17.6831967780099,-1.25709479715135,115.162197134421));
#51042=CARTESIAN_POINT('Ctrl Pts',(17.8633620834074,-1.36516570458449,115.175222025971));
#51043=CARTESIAN_POINT('Ctrl Pts',(18.1604819038664,-1.47854845945174,115.194753812955));
#51044=CARTESIAN_POINT('Ctrl Pts',(18.582786890695,-1.51417568969967,115.220787745291));
#51045=CARTESIAN_POINT('Ctrl Pts',(18.9983836416472,-1.43149328105734,115.246809679889));
#51046=CARTESIAN_POINT('Ctrl Pts',(19.374473528925,-1.23714016652633,115.27282057109));
#51047=CARTESIAN_POINT('Ctrl Pts',(19.6822598946567,-0.946311359030486,
115.298817689622));
#51048=CARTESIAN_POINT('Ctrl Pts',(19.8967480474023,-0.582015055171165,
115.324801432878));
#51049=CARTESIAN_POINT('Ctrl Pts',(20.0386193688326,-0.0359715504243672,
115.359425895719));
#51050=CARTESIAN_POINT('Ctrl Pts',(19.941536265269,0.535299448860012,115.394018366274));
#51051=CARTESIAN_POINT('Ctrl Pts',(19.6668198938765,0.944384240575756,115.424255526598));
#51052=CARTESIAN_POINT('Ctrl Pts',(19.4671125145751,1.13894829771433,115.44152396901));
#51053=CARTESIAN_POINT('Ctrl Pts',(19.2416596715355,1.3035791132569,115.458786271138));
#51054=CARTESIAN_POINT('Ctrl Pts',(19.0175256336374,1.40399060754221,115.473882214218));
#51055=CARTESIAN_POINT('Ctrl Pts',(18.8150509122225,1.45460978349152,115.486814484407));
#51056=CARTESIAN_POINT('Ctrl Pts',(18.7124011810244,1.4728082953005,115.493279478184));
#51057=CARTESIAN_POINT('Ctrl Pts',(18.6259805295674,1.48196183269604,115.498665769091));
#51058=CARTESIAN_POINT('Ctrl Pts',(18.5565983881251,1.48554743331276,115.502974301951));
#51059=CARTESIAN_POINT('Ctrl Pts',(18.275006635137,1.49093350233563,115.520445423601));
#51060=CARTESIAN_POINT('Ctrl Pts',(17.7643189677256,1.36044159259875,115.552131188091));
#51061=CARTESIAN_POINT('Ctrl Pts',(17.3297966145357,0.957318076594017,115.587783846009));
#51062=CARTESIAN_POINT('Ctrl Pts',(17.1366050542202,0.593850002954031,115.613220643608));
#51063=CARTESIAN_POINT('Ctrl Pts',(17.0708721336454,0.399095376421441,115.625931295202));
#51064=CARTESIAN_POINT('Ctrl Pts',(17.0385717481457,0.238286256682236,115.636095006768));
#51065=CARTESIAN_POINT('Ctrl Pts',(17.0000053948983,-0.0873641069959773,
115.656416799589));
#51066=CARTESIAN_POINT('Ctrl Pts',(17.0954817402936,-0.627463061463085,
115.689403138097));
#51067=CARTESIAN_POINT('Ctrl Pts',(17.5683032047114,-1.2202390337612,115.734986014693));
#51068=CARTESIAN_POINT('Ctrl Pts',(18.2073749791171,-1.48915585063008,115.776682365231));
#51069=CARTESIAN_POINT('Ctrl Pts',(18.827714255502,-1.46536270236631,115.81451460932));
#51070=CARTESIAN_POINT('Ctrl Pts',(19.3387291215206,-1.24252555435953,115.848504801486));
#51071=CARTESIAN_POINT('Ctrl Pts',(19.7323390465761,-0.84870905484788,115.882433969696));
#51072=CARTESIAN_POINT('Ctrl Pts',(19.917317868452,-0.424382854990528,115.910656120296));
#51073=CARTESIAN_POINT('Ctrl Pts',(19.9647758151583,-0.0623666971425709,
115.933200950891));
#51074=CARTESIAN_POINT('Ctrl Pts',(19.9494967945027,0.210678396553568,115.950093741532));
#51075=CARTESIAN_POINT('Ctrl Pts',(19.8946537689314,0.431722595099945,115.964156440341));
#51076=CARTESIAN_POINT('Ctrl Pts',(19.8267524040723,0.599946781165768,115.975398400255));
#51077=CARTESIAN_POINT('Ctrl Pts',(19.7020401592803,0.841706463647344,115.992253058882));
#51078=CARTESIAN_POINT('Ctrl Pts',(19.4317853790293,1.15561589179994,116.017502153899));
#51079=CARTESIAN_POINT('Ctrl Pts',(18.9444409086331,1.41307035879397,116.051097502054));
#51080=CARTESIAN_POINT('Ctrl Pts',(18.3979015457458,1.47453073660614,116.084620132269));
#51081=CARTESIAN_POINT('Ctrl Pts',(18.0004069582635,1.36793073631313,116.1097063674));
#51082=CARTESIAN_POINT('Ctrl Pts',(17.763366663899,1.23962198295239,116.126406802779));
#51083=CARTESIAN_POINT('Ctrl Pts',(17.6140480708204,1.1398854968943,116.137534246267));
#51084=CARTESIAN_POINT('Ctrl Pts',(17.3790836560323,0.929981622126309,116.156989690435));
#51085=CARTESIAN_POINT('Ctrl Pts',(17.2215832331742,0.679602546844773,116.175024509631));
#51086=CARTESIAN_POINT('Ctrl Pts',(17.1450352066694,0.469669982396278,116.188878617737));
#51087=CARTESIAN_POINT('Ctrl Pts',(17.1249441446997,0.405767087289566,116.193033537477));
#51088=CARTESIAN_POINT('Ctrl Pts',(17.1079301441042,0.340970796669862,116.197187251518));
#51089=CARTESIAN_POINT('Ctrl Pts',(17.0939473695056,0.275494153967272,116.201339691278));
#51090=CARTESIAN_POINT('Ctrl Pts',(17.0830227708597,0.209443458520346,116.205490910608));
#51091=CARTESIAN_POINT('Ctrl Pts',(17.0726655652121,0.120824547382831,116.211024197657));
#51092=CARTESIAN_POINT('Ctrl Pts',(17.0610173800014,-0.124379540531134,
116.226234061721));
#51093=CARTESIAN_POINT('Ctrl Pts',(17.1369245229291,-0.5249310381429,116.251084258337));
#51094=CARTESIAN_POINT('Ctrl Pts',(17.4255200195769,-0.984001270082908,
116.284135719174));
#51095=CARTESIAN_POINT('Ctrl Pts',(17.8607605682645,-1.30506353431624,116.317102617813));
#51096=CARTESIAN_POINT('Ctrl Pts',(18.3818866043649,-1.44455243472689,116.349983938512));
#51097=CARTESIAN_POINT('Ctrl Pts',(18.916470350186,-1.38418902476214,116.382777928971));
#51098=CARTESIAN_POINT('Ctrl Pts',(19.3908578736671,-1.13333494037052,116.415483428707));
#51099=CARTESIAN_POINT('Ctrl Pts',(19.662129258784,-0.817824110576332,116.440850810503));
#51100=CARTESIAN_POINT('Ctrl Pts',(19.7921004518703,-0.556121431420674,
116.458936888485));
#51101=CARTESIAN_POINT('Ctrl Pts',(19.8690655500124,-0.335782443963777,
116.473391787428));
#51102=CARTESIAN_POINT('Ctrl Pts',(19.9308282800101,0.0701141608640084,
116.498652513443));
#51103=CARTESIAN_POINT('Ctrl Pts',(19.7975561020439,0.653379656102897,116.534635638022));
#51104=CARTESIAN_POINT('Ctrl Pts',(19.3238121146665,1.18955843336623,116.577647401962));
#51105=CARTESIAN_POINT('Ctrl Pts',(18.6542573597491,1.43288587092525,116.620488268205));
#51106=CARTESIAN_POINT('Ctrl Pts',(17.9525424324882,1.32679118729713,116.663155847902));
#51107=CARTESIAN_POINT('Ctrl Pts',(17.4716228570456,0.961996366384522,116.699450989897));
#51108=CARTESIAN_POINT('Ctrl Pts',(17.2242845453766,0.540894020126181,116.729451046567));
#51109=CARTESIAN_POINT('Ctrl Pts',(17.0944240343639,0.041457592091441,116.761140226464));
#51110=CARTESIAN_POINT('Ctrl Pts',(17.2055334687691,-0.610901669378824,
116.8006093271));
#51111=CARTESIAN_POINT('Ctrl Pts',(17.7327235525077,-1.19996474577183,116.847741724244));
#51112=CARTESIAN_POINT('Ctrl Pts',(18.4886274023919,-1.41711476065944,116.894641370113));
#51113=CARTESIAN_POINT('Ctrl Pts',(19.2403913761961,-1.19999329817096,116.941306241231));
#51114=CARTESIAN_POINT('Ctrl Pts',(19.7589583230562,-0.618976305235332,
116.987734609023));
#51115=CARTESIAN_POINT('Ctrl Pts',(19.866303857657,0.0173456111094613,117.026226666982));
#51116=CARTESIAN_POINT('Ctrl Pts',(19.7405351404932,0.500732911611066,117.05690073817));
#51117=CARTESIAN_POINT('Ctrl Pts',(19.5511427517233,0.822664799957136,117.079846452937));
#51118=CARTESIAN_POINT('Ctrl Pts',(19.2800271222083,1.07822752115069,117.102732140544));
#51119=CARTESIAN_POINT('Ctrl Pts',(18.840099008821,1.30647550082486,117.13316636068));
#51120=CARTESIAN_POINT('Ctrl Pts',(18.2057864265544,1.34185814168128,117.171058787474));
#51121=CARTESIAN_POINT('Ctrl Pts',(17.5421074842011,0.974328602971076,117.216288928054));
#51122=CARTESIAN_POINT('Ctrl Pts',(17.1777038347398,0.313792671011465,117.261278280207));
#51123=CARTESIAN_POINT('Ctrl Pts',(17.2203225463522,-0.435464225919962,
117.306027156934));
#51124=CARTESIAN_POINT('Ctrl Pts',(17.652724667813,-1.04386133116569,117.350536141848));
#51125=CARTESIAN_POINT('Ctrl Pts',(18.3388239098277,-1.32745573236693,117.39480611765));
#51126=CARTESIAN_POINT('Ctrl Pts',(19.0667149711576,-1.20320856043253,117.438838249758));
#51127=CARTESIAN_POINT('Ctrl Pts',(19.6139786084161,-0.713397943859653,
117.482633994782));
#51128=CARTESIAN_POINT('Ctrl Pts',(19.8156811381899,-0.0112791664943189,
117.526195091984));
#51129=CARTESIAN_POINT('Ctrl Pts',(19.6140022601783,0.686784214414896,117.569523562413));
#51130=CARTESIAN_POINT('Ctrl Pts',(19.0747275941947,1.16798331893147,117.612621710931));
#51131=CARTESIAN_POINT('Ctrl Pts',(18.3658643708616,1.28788138840837,117.655492120034));
#51132=CARTESIAN_POINT('Ctrl Pts',(17.7053431257873,1.01371279747136,117.69813764302));
#51133=CARTESIAN_POINT('Ctrl Pts',(17.2940790801678,0.433188982502828,117.740561406275));
#51134=CARTESIAN_POINT('Ctrl Pts',(17.2549003691858,-0.273508324804743,
117.782766808914));
#51135=CARTESIAN_POINT('Ctrl Pts',(17.5959737510632,-0.889574255288579,
117.824757505323));
#51136=CARTESIAN_POINT('Ctrl Pts',(18.2094168755739,-1.22806570874149,117.866537413039));
#51137=CARTESIAN_POINT('Ctrl Pts',(18.9055013390443,-1.18847566627298,117.908110699435));
#51138=CARTESIAN_POINT('Ctrl Pts',(19.4709991235593,-0.786645501256251,
117.949481800211));
#51139=CARTESIAN_POINT('Ctrl Pts',(19.7349121554302,-0.148494032303403,
117.990655350317));
#51140=CARTESIAN_POINT('Ctrl Pts',(19.6384296844279,0.41595364745626,118.024806143826));
#51141=CARTESIAN_POINT('Ctrl Pts',(19.3912822005401,0.783910465160815,118.052032979065));
#51142=CARTESIAN_POINT('Ctrl Pts',(19.0539455301924,1.06997780245999,118.079198326187));
#51143=CARTESIAN_POINT('Ctrl Pts',(18.5086041618223,1.22692728472169,118.113040992046));
#51144=CARTESIAN_POINT('Ctrl Pts',(17.8570681242743,1.03871258992206,118.153475788182));
#51145=CARTESIAN_POINT('Ctrl Pts',(17.4074661243136,0.535028360348281,118.193739748399));
#51146=CARTESIAN_POINT('Ctrl Pts',(17.295184410072,-0.12802353903353,118.233838994046));
#51147=CARTESIAN_POINT('Ctrl Pts',(17.5518536435643,-0.746678185841251,
118.273779650817));
#51148=CARTESIAN_POINT('Ctrl Pts',(18.09623557474,-1.13252353284961,118.313568149567));
#51149=CARTESIAN_POINT('Ctrl Pts',(18.7600131800788,-1.16944565236424,118.353211038631));
#51150=CARTESIAN_POINT('Ctrl Pts',(19.3396804878931,-0.848740522078599,
118.392715097256));
#51151=CARTESIAN_POINT('Ctrl Pts',(19.6587833880623,-0.270665095166121,
118.432087186673));
#51152=CARTESIAN_POINT('Ctrl Pts',(19.6216208701028,0.386364157140476,118.471334476116));
#51153=CARTESIAN_POINT('Ctrl Pts',(19.2416211971827,0.921545428620454,118.510464030869));
#51154=CARTESIAN_POINT('Ctrl Pts',(18.7378784200697,1.12977499085113,118.542980260458));
#51155=CARTESIAN_POINT('Ctrl Pts',(18.3152260681784,1.11706291748731,118.56894164302));
#51156=CARTESIAN_POINT('Ctrl Pts',(18.013631331558,1.02122659296196,118.588388203893));
#51157=CARTESIAN_POINT('Ctrl Pts',(17.7507020897944,0.845342251383026,118.607810663731));
#51158=CARTESIAN_POINT('Ctrl Pts',(17.5469576086983,0.604112404067775,118.62721063314));
#51159=CARTESIAN_POINT('Ctrl Pts',(17.418115189222,0.316066123273868,118.646588439489));
#51160=CARTESIAN_POINT('Ctrl Pts',(17.3740914074908,0.00406156609269027,
118.665945648007));
#51161=CARTESIAN_POINT('Ctrl Pts',(17.418105330468,-0.307731076500601,118.68528270408));
#51162=CARTESIAN_POINT('Ctrl Pts',(17.5252095909573,-0.546868258948941,
118.701381492349));
#51163=CARTESIAN_POINT('Ctrl Pts',(17.6479384162453,-0.714878730507821,
118.714251085885));
#51164=CARTESIAN_POINT('Ctrl Pts',(17.7929243818857,-0.863723509943578,
118.727115583167));
#51165=CARTESIAN_POINT('Ctrl Pts',(18.0972164483336,-1.06793358028532,118.74961267773));
#51166=CARTESIAN_POINT('Ctrl Pts',(18.6276378637832,-1.15815365828481,118.781712261723));
#51167=CARTESIAN_POINT('Ctrl Pts',(19.2238118827329,-0.91106020954,118.820176086249));
#51168=CARTESIAN_POINT('Ctrl Pts',(19.5340790733567,-0.473298914368946,
118.852189669591));
#51169=CARTESIAN_POINT('Ctrl Pts',(19.6045033571726,-0.115359348913955,
118.874582530202));
#51170=CARTESIAN_POINT('Ctrl Pts',(19.6017475647411,0.0911640829913528,
118.88737350014));
#51171=CARTESIAN_POINT('Ctrl Pts',(19.5700196370974,0.29559108219492,118.900162446911));
#51172=CARTESIAN_POINT('Ctrl Pts',(19.4770780543413,0.538342967989427,118.916143236651));
#51173=CARTESIAN_POINT('Ctrl Pts',(19.2273588011135,0.871529045839169,118.941704029868));
#51174=CARTESIAN_POINT('Ctrl Pts',(18.7588367207674,1.13058490335296,118.973640684375));
#51175=CARTESIAN_POINT('Ctrl Pts',(18.1172887995021,1.09452313569986,119.011950738852));
#51176=CARTESIAN_POINT('Ctrl Pts',(17.593388380079,0.722780783019972,119.050254797413));
#51177=CARTESIAN_POINT('Ctrl Pts',(17.3886684004257,0.228286678671025,119.082177254148));
#51178=CARTESIAN_POINT('Ctrl Pts',(17.4011923319186,-0.187547154371747,
119.107720239302));
#51179=CARTESIAN_POINT('Ctrl Pts',(17.479741012236,-0.43518291567232,119.123688362763));
#51180=CARTESIAN_POINT('Ctrl Pts',(17.5695979738663,-0.592074644579124,
119.134867535548));
#51181=CARTESIAN_POINT('Ctrl Pts',(17.6297289359476,-0.675697287840335,
119.1412564699));
#51182=CARTESIAN_POINT('Ctrl Pts',(17.6957161316275,-0.754921963867992,
119.147645877012));
#51183=CARTESIAN_POINT('Ctrl Pts',(17.7882499830905,-0.84489988474299,119.155633946795));
#51184=CARTESIAN_POINT('Ctrl Pts',(17.9550205699679,-0.966828303763707,
119.168415926821));
#51185=CARTESIAN_POINT('Ctrl Pts',(18.1925073400234,-1.07312652027406,119.184398568056));
#51186=CARTESIAN_POINT('Ctrl Pts',(18.5018237176362,-1.11680179614521,119.203585076302));
#51187=CARTESIAN_POINT('Ctrl Pts',(18.8112727437243,-1.07312083019676,119.222781017226));
#51188=CARTESIAN_POINT('Ctrl Pts',(19.0966922989243,-0.945425429896232,
119.241986576724));
#51189=CARTESIAN_POINT('Ctrl Pts',(19.3357397025375,-0.743574694906012,
119.261203548649));
#51190=CARTESIAN_POINT('Ctrl Pts',(19.5096763702265,-0.483296157484075,
119.280432047793));
#51191=CARTESIAN_POINT('Ctrl Pts',(19.604829263032,-0.184805761734769,119.299674358162));
#51192=CARTESIAN_POINT('Ctrl Pts',(19.6136282032755,0.128548869667553,119.318929822438));
#51193=CARTESIAN_POINT('Ctrl Pts',(19.5483562428395,0.381754662526241,119.334989622353));
#51194=CARTESIAN_POINT('Ctrl Pts',(19.4555027014667,0.567586338753027,119.347844753828));
#51195=CARTESIAN_POINT('Ctrl Pts',(19.3083285466207,0.781707993580481,119.363921119013));
#51196=CARTESIAN_POINT('Ctrl Pts',(19.0213883195784,1.0173014385066,119.386447876364));
#51197=CARTESIAN_POINT('Ctrl Pts',(18.5601806816014,1.14326482672377,119.415452744608));
#51198=CARTESIAN_POINT('Ctrl Pts',(18.0870469004768,1.06976794361554,119.444502870166));
#51199=CARTESIAN_POINT('Ctrl Pts',(17.6845073765261,0.809000046868888,119.473601565479));
#51200=CARTESIAN_POINT('Ctrl Pts',(17.4231181242213,0.405838898540841,119.502752060927));
#51201=CARTESIAN_POINT('Ctrl Pts',(17.3490598832109,-0.0697983875198877,
119.531957712525));
#51202=CARTESIAN_POINT('Ctrl Pts',(17.4759534440631,-0.535171725229621,
119.561221496182));
#51203=CARTESIAN_POINT('Ctrl Pts',(17.7314548399343,-0.846550437506931,
119.58565944407));
#51204=CARTESIAN_POINT('Ctrl Pts',(17.999207559364,-1.0170868157945,119.605241751292));
#51205=CARTESIAN_POINT('Ctrl Pts',(18.2967905723551,-1.12863703662001,119.624846422395));
#51206=CARTESIAN_POINT('Ctrl Pts',(18.701022235534,-1.14581433888424,119.649394327387));
#51207=CARTESIAN_POINT('Ctrl Pts',(19.1533010528138,-0.965969567310355,
119.678922596865));
#51208=CARTESIAN_POINT('Ctrl Pts',(19.4935242230618,-0.616264784255005,
119.708524488639));
#51209=CARTESIAN_POINT('Ctrl Pts',(19.6616806751607,-0.15688731828813,119.738203011753));
#51210=CARTESIAN_POINT('Ctrl Pts',(19.6274500840142,0.332402173060607,119.767961008938));
#51211=CARTESIAN_POINT('Ctrl Pts',(19.3957290628344,0.766238455283539,119.797801335606));
#51212=CARTESIAN_POINT('Ctrl Pts',(19.0059018782433,1.06845895995986,119.827726746298));
#51213=CARTESIAN_POINT('Ctrl Pts',(18.5252515327408,1.18543071772727,119.857739979944));
#51214=CARTESIAN_POINT('Ctrl Pts',(18.037234743022,1.09564506473,119.887843657137));
#51215=CARTESIAN_POINT('Ctrl Pts',(17.6956019306827,0.860470084296629,119.913007640695));
#51216=CARTESIAN_POINT('Ctrl Pts',(17.4972936032911,0.600305772965447,119.93318661626));
#51217=CARTESIAN_POINT('Ctrl Pts',(17.3569038509229,0.304279815543778,119.953397785618));
#51218=CARTESIAN_POINT('Ctrl Pts',(17.3041660284991,-0.109796929925252,
119.978723169803));
#51219=CARTESIAN_POINT('Ctrl Pts',(17.4498994353956,-0.59078091166106,120.009214030095));
#51220=CARTESIAN_POINT('Ctrl Pts',(17.7804655429487,-0.971566966837065,
120.039807705564));
#51221=CARTESIAN_POINT('Ctrl Pts',(18.2393086861239,-1.18486584665598,120.07050641441));
#51222=CARTESIAN_POINT('Ctrl Pts',(18.7470163437987,-1.1921729938516,120.101312384752));
#51223=CARTESIAN_POINT('Ctrl Pts',(19.215087635489,-0.990765643040621,120.132227714623));
#51224=CARTESIAN_POINT('Ctrl Pts',(19.5613155231427,-0.614392148089554,
120.163254460057));
#51225=CARTESIAN_POINT('Ctrl Pts',(19.7242152497417,-0.127659401515012,
120.194394583265));
#51226=CARTESIAN_POINT('Ctrl Pts',(19.6739207775415,0.385049104109546,120.225649979257));
#51227=CARTESIAN_POINT('Ctrl Pts',(19.4176458057697,0.834175476321175,120.257022460356));
#51228=CARTESIAN_POINT('Ctrl Pts',(18.998699632526,1.14061462596676,120.288513762116));
#51229=CARTESIAN_POINT('Ctrl Pts',(18.4891879156563,1.24962833189955,120.320125537776));
#51230=CARTESIAN_POINT('Ctrl Pts',(17.9776202690671,1.14060959036587,120.351859359126));
#51231=CARTESIAN_POINT('Ctrl Pts',(17.5535525982464,0.830952823101709,120.383716714854));
#51232=CARTESIAN_POINT('Ctrl Pts',(17.2919248389954,0.373308289212946,120.415699010712));
#51233=CARTESIAN_POINT('Ctrl Pts',(17.2398314509524,-0.153353235375788,
120.447807567348));
#51234=CARTESIAN_POINT('Ctrl Pts',(17.4080575955601,-0.657352082285856,
120.480043619757));
#51235=CARTESIAN_POINT('Ctrl Pts',(17.7689006127485,-1.05024513051325,120.512408315922));
#51236=CARTESIAN_POINT('Ctrl Pts',(18.2607097297302,-1.26233444597482,120.544902716827));
#51237=CARTESIAN_POINT('Ctrl Pts',(18.7984052352737,-1.25502080659343,120.577527795704));
#51238=CARTESIAN_POINT('Ctrl Pts',(19.2881848794747,-1.0278144553583,120.610284437319));
#51239=CARTESIAN_POINT('Ctrl Pts',(19.6438781749597,-0.61873033468329,120.643173436616));
#51240=CARTESIAN_POINT('Ctrl Pts',(19.8020987090859,-0.0979461688159152,
120.676195498978));
#51241=CARTESIAN_POINT('Ctrl Pts',(19.7335320823132,0.444227716269205,120.709351239055));
#51242=CARTESIAN_POINT('Ctrl Pts',(19.4483480211883,0.912997875362089,120.742641182014));
#51243=CARTESIAN_POINT('Ctrl Pts',(18.9947430992497,1.22566304840365,120.776065760162));
#51244=CARTESIAN_POINT('Ctrl Pts',(18.4508057834443,1.32618611440986,120.809625317582));
#51245=CARTESIAN_POINT('Ctrl Pts',(17.9110852264692,1.19525527808251,120.843320100399));
#51246=CARTESIAN_POINT('Ctrl Pts',(17.4701505494149,0.853917314146234,120.877150274951));
#51247=CARTESIAN_POINT('Ctrl Pts',(17.2060388865232,0.360310149126953,120.911115893666));
#51248=CARTESIAN_POINT('Ctrl Pts',(17.1664153816519,-0.200398871563149,
120.945216959522));
#51249=CARTESIAN_POINT('Ctrl Pts',(17.3116264220795,-0.597882955951257,
120.970894211169));
#51250=CARTESIAN_POINT('Ctrl Pts',(17.4713230749973,-0.824292723162997,
120.988054644643));
#51251=CARTESIAN_POINT('Ctrl Pts',(17.5930295495418,-0.963403094471689,
120.999506127854));
#51252=CARTESIAN_POINT('Ctrl Pts',(17.8429222056168,-1.17180944522949,121.019575839724));
#51253=CARTESIAN_POINT('Ctrl Pts',(18.2831358555107,-1.3472696457857,121.048331046648));
#51254=CARTESIAN_POINT('Ctrl Pts',(18.8536622082132,-1.32345121615729,121.082971735828));
#51255=CARTESIAN_POINT('Ctrl Pts',(19.3666123501032,-1.06776818445665,121.11774633767));
#51256=CARTESIAN_POINT('Ctrl Pts',(19.7318189194698,-0.623135744515387,
121.152654299799));
#51257=CARTESIAN_POINT('Ctrl Pts',(19.8841229814082,-0.0660261383455702,
121.187694946127));
#51258=CARTESIAN_POINT('Ctrl Pts',(19.7952691811095,0.506861240356869,121.22286752838));
#51259=CARTESIAN_POINT('Ctrl Pts',(19.4789909654556,0.995298037449156,121.258171199464));
#51260=CARTESIAN_POINT('Ctrl Pts',(18.9889997447394,1.31312136899922,121.293605027892));
#51261=CARTESIAN_POINT('Ctrl Pts',(18.4098258930854,1.40341469896206,121.329167991327));
#51262=CARTESIAN_POINT('Ctrl Pts',(17.8422514541543,1.2487159173822,121.364858980876));
#51263=CARTESIAN_POINT('Ctrl Pts',(17.3857498366357,0.874358654879244,121.400676801254));
#51264=CARTESIAN_POINT('Ctrl Pts',(17.1210452069084,0.344343613450397,121.436620170121));
#51265=CARTESIAN_POINT('Ctrl Pts',(17.0958251015548,-0.249607404749667,
121.472687721701));
#51266=CARTESIAN_POINT('Ctrl Pts',(17.3161507636215,-0.803935931388206,
121.508878001574));
#51267=CARTESIAN_POINT('Ctrl Pts',(17.7451068582081,-1.22131693446959,121.545189480257));
#51268=CARTESIAN_POINT('Ctrl Pts',(18.3089795239874,-1.42776624833079,121.581620531396));
#51269=CARTESIAN_POINT('Ctrl Pts',(18.9099344796403,-1.38575758159487,121.618169476059));
#51270=CARTESIAN_POINT('Ctrl Pts',(19.443003408243,-1.10105588624391,121.654834501032));
#51271=CARTESIAN_POINT('Ctrl Pts',(19.814447080578,-0.621956720707161,121.691613814933));
#51272=CARTESIAN_POINT('Ctrl Pts',(19.9582412943487,-0.0311460741792062,
121.728505359742));
#51273=CARTESIAN_POINT('Ctrl Pts',(19.8478423707596,0.568675584892993,121.765507307081));
#51274=CARTESIAN_POINT('Ctrl Pts',(19.5010738542693,1.07254435780881,121.802617407826));
#51275=CARTESIAN_POINT('Ctrl Pts',(18.9772465487843,1.39174398963045,121.839833580231));
#51276=CARTESIAN_POINT('Ctrl Pts',(18.3670349923433,1.46935809393124,121.877153590267));
#51277=CARTESIAN_POINT('Ctrl Pts',(17.7767415245785,1.29047771303663,121.91457510912));
#51278=CARTESIAN_POINT('Ctrl Pts',(17.3097639110163,0.88502066898406,121.952095792454));
#51279=CARTESIAN_POINT('Ctrl Pts',(17.0484530789278,0.322744770605088,121.98971320241));
#51280=CARTESIAN_POINT('Ctrl Pts',(17.0395741793232,-0.29877511550778,122.027424807101));
#51281=CARTESIAN_POINT('Ctrl Pts',(17.2859276060077,-0.871100232399064,
122.065228088574));
#51282=CARTESIAN_POINT('Ctrl Pts',(17.7456411246251,-1.29387701195727,122.103120366714));
#51283=CARTESIAN_POINT('Ctrl Pts',(18.3392916665445,-1.49245955151488,122.141098983942));
#51284=CARTESIAN_POINT('Ctrl Pts',(18.9636467540723,-1.43110986029732,122.179161195417));
#51285=CARTESIAN_POINT('Ctrl Pts',(19.5096427527803,-1.11943132446743,122.217304158637));
#51286=CARTESIAN_POINT('Ctrl Pts',(19.8814701962045,-0.610888906864692,
122.255525076564));
#51287=CARTESIAN_POINT('Ctrl Pts',(20.0134084028596,0.00638374819795061,
122.293820960483));
#51288=CARTESIAN_POINT('Ctrl Pts',(19.8814680357448,0.624863883396621,122.332188933733));
#51289=CARTESIAN_POINT('Ctrl Pts',(19.5077372244298,1.13643840843378,122.370625859871));
#51290=CARTESIAN_POINT('Ctrl Pts',(18.9567207702999,1.45127557085421,122.409128868261));
#51291=CARTESIAN_POINT('Ctrl Pts',(18.3241217337611,1.51368240153528,122.447694658652));
#51292=CARTESIAN_POINT('Ctrl Pts',(17.7202826349282,1.31196813537611,122.486320211507));
#51293=CARTESIAN_POINT('Ctrl Pts',(17.2508103246174,0.880536550537675,122.525002285958));
#51294=CARTESIAN_POINT('Ctrl Pts',(16.9981604164449,0.294249197224712,122.563737660687));
#51295=CARTESIAN_POINT('Ctrl Pts',(17.0060423714049,-0.274042958784632,
122.598213625129));
#51296=CARTESIAN_POINT('Ctrl Pts',(17.1818706810392,-0.73303144472968,122.628410343682));
#51297=CARTESIAN_POINT('Ctrl Pts',(17.5191721715142,-1.18310393837461,122.662947355674));
#51298=CARTESIAN_POINT('Ctrl Pts',(18.1531350042187,-1.53390972067408,122.706165522702));
#51299=CARTESIAN_POINT('Ctrl Pts',(19.0227874461394,-1.48519217492529,122.758094642985));
#51300=CARTESIAN_POINT('Ctrl Pts',(19.7338192740336,-0.980774656373063,
122.810082875595));
#51301=CARTESIAN_POINT('Ctrl Pts',(20.067922277282,-0.174626022127283,122.862122158172));
#51302=CARTESIAN_POINT('Ctrl Pts',(19.921708544036,0.68662933685667,122.914204231648));
#51303=CARTESIAN_POINT('Ctrl Pts',(19.4364076102001,1.22943043838242,122.957634782588));
#51304=CARTESIAN_POINT('Ctrl Pts',(18.9192757117743,1.45961435937841,122.992392354061));
#51305=CARTESIAN_POINT('Ctrl Pts',(18.5146998498917,1.51727349960696,123.017500336371));
#51306=CARTESIAN_POINT('Ctrl Pts',(18.1254479581993,1.46800683442712,123.041646590114));
#51307=CARTESIAN_POINT('Ctrl Pts',(17.65765089863,1.28524666288511,123.072557499479));
#51308=CARTESIAN_POINT('Ctrl Pts',(17.1864413110902,0.84817385210292,123.111201426539));
#51309=CARTESIAN_POINT('Ctrl Pts',(16.9818560590682,0.238917012125818,123.149847159061));
#51310=CARTESIAN_POINT('Ctrl Pts',(17.0077477842283,-0.262729802221198,
123.180762273051));
#51311=CARTESIAN_POINT('Ctrl Pts',(17.1549558342261,-0.742832495303323,
123.211674984775));
#51312=CARTESIAN_POINT('Ctrl Pts',(17.5555345576308,-1.24539323375308,123.250310351106));
#51313=CARTESIAN_POINT('Ctrl Pts',(18.2066766855254,-1.51951236558385,123.292795159863));
#51314=CARTESIAN_POINT('Ctrl Pts',(18.8397001520098,-1.49532848220801,123.331402485356));
#51315=CARTESIAN_POINT('Ctrl Pts',(19.361933038917,-1.2676766648096,123.36613474992));
#51316=CARTESIAN_POINT('Ctrl Pts',(19.7646594303858,-0.864798752237798,
123.400850262946));
#51317=CARTESIAN_POINT('Ctrl Pts',(19.992247479715,-0.343129638214644,123.435546682762));
#51318=CARTESIAN_POINT('Ctrl Pts',(20.0134975784261,0.225403110709894,123.470221342828));
#51319=CARTESIAN_POINT('Ctrl Pts',(19.8256820027275,0.761912608646907,123.504872214536));
#51320=CARTESIAN_POINT('Ctrl Pts',(19.516918297423,1.12076930887003,123.533725575818));
#51321=CARTESIAN_POINT('Ctrl Pts',(19.2041810039955,1.32499554631978,123.556794181975));
#51322=CARTESIAN_POINT('Ctrl Pts',(18.8020588760868,1.49233095074489,123.583695662073));
#51323=CARTESIAN_POINT('Ctrl Pts',(18.1960164011262,1.52254678614699,123.620174599657));
#51324=CARTESIAN_POINT('Ctrl Pts',(17.6216673694243,1.24564088295246,123.658522649907));
#51325=CARTESIAN_POINT('Ctrl Pts',(17.2833151529131,0.880111521286915,123.689167672577));
#51326=CARTESIAN_POINT('Ctrl Pts',(17.1050831264071,0.552606139546885,123.712134313292));
#51327=CARTESIAN_POINT('Ctrl Pts',(16.9816547923198,0.0706959663075114,
123.742732173804));
#51328=CARTESIAN_POINT('Ctrl Pts',(17.0529092044043,-0.496279877167484,
123.777112906262));
#51329=CARTESIAN_POINT('Ctrl Pts',(17.3864957981709,-1.02604026133052,123.815255128178));
#51330=CARTESIAN_POINT('Ctrl Pts',(17.857593613417,-1.37397111071324,123.850964243175));
#51331=CARTESIAN_POINT('Ctrl Pts',(18.4515962038669,-1.51829287387834,123.888044644597));
#51332=CARTESIAN_POINT('Ctrl Pts',(19.0746522170704,-1.40326627781162,123.926485479005));
#51333=CARTESIAN_POINT('Ctrl Pts',(19.5520449521414,-1.07433327180886,123.961659739466));
#51334=CARTESIAN_POINT('Ctrl Pts',(19.7870135179904,-0.729922634281818,
123.987199138138));
#51335=CARTESIAN_POINT('Ctrl Pts',(19.9172825726675,-0.412389600249223,
124.008461419526));
#51336=CARTESIAN_POINT('Ctrl Pts',(19.9813821346012,-0.0901260863987032,
124.028642265937));
#51337=CARTESIAN_POINT('Ctrl Pts',(19.9464919895927,0.322871316840072,124.054100150558));
#51338=CARTESIAN_POINT('Ctrl Pts',(19.7988560610193,0.709540527634926,124.079522689038));
#51339=CARTESIAN_POINT('Ctrl Pts',(19.5502809158787,1.03976970882056,124.104909666808));
#51340=CARTESIAN_POINT('Ctrl Pts',(19.2205019215012,1.28789198571529,124.130259814538));
#51341=CARTESIAN_POINT('Ctrl Pts',(18.8675304954949,1.42261786918923,124.153463104108));
#51342=CARTESIAN_POINT('Ctrl Pts',(18.5284830739033,1.46304402439271,124.174529127565));
#51343=CARTESIAN_POINT('Ctrl Pts',(18.1207874834896,1.4260614944801,124.199779233887));
#51344=CARTESIAN_POINT('Ctrl Pts',(17.6438940253866,1.2206283929953,124.231286143554));
#51345=CARTESIAN_POINT('Ctrl Pts',(17.2233006573008,0.762755887841534,124.269003086711));
#51346=CARTESIAN_POINT('Ctrl Pts',(17.0268753162689,0.174604680404742,124.306625880741));
#51347=CARTESIAN_POINT('Ctrl Pts',(17.0876702801681,-0.440949978759675,
124.344152137287));
#51348=CARTESIAN_POINT('Ctrl Pts',(17.3937696919832,-0.976537539345891,
124.381579352596));
#51349=CARTESIAN_POINT('Ctrl Pts',(17.8905867113653,-1.33941486357803,124.41890518565));
#51350=CARTESIAN_POINT('Ctrl Pts',(18.4906153716989,-1.46735186134762,124.456127313473));
#51351=CARTESIAN_POINT('Ctrl Pts',(19.0888593629504,-1.33941777641846,124.493243511411));
#51352=CARTESIAN_POINT('Ctrl Pts',(19.5812312587733,-0.97933823951139,124.530251612046));
#51353=CARTESIAN_POINT('Ctrl Pts',(19.8826841702414,-0.45113379238791,124.567149528264));
#51354=CARTESIAN_POINT('Ctrl Pts',(19.9419184246875,0.15228968271957,124.603935243626));
#51355=CARTESIAN_POINT('Ctrl Pts',(19.7501149544944,0.72549274055214,124.640606820178));
#51356=CARTESIAN_POINT('Ctrl Pts',(19.3422099788232,1.16895227798287,124.677162396834));
#51357=CARTESIAN_POINT('Ctrl Pts',(18.7905344628525,1.4063573661534,124.713600191806));
#51358=CARTESIAN_POINT('Ctrl Pts',(18.1919768114847,1.39775285517752,124.749918502117));
#51359=CARTESIAN_POINT('Ctrl Pts',(17.650949463827,1.14625964667207,124.786115706138));
#51360=CARTESIAN_POINT('Ctrl Pts',(17.2611574231578,0.697245715919318,124.822190264427));
#51361=CARTESIAN_POINT('Ctrl Pts',(17.0893550841156,0.130141700592976,124.858140721292));
#51362=CARTESIAN_POINT('Ctrl Pts',(17.1639091103876,-0.45562104348777,124.893965705161));
#51363=CARTESIAN_POINT('Ctrl Pts',(17.4701273616986,-0.958058662722596,
124.929663929076));
#51364=CARTESIAN_POINT('Ctrl Pts',(17.9531200725725,-1.29040433417455,124.965234192037));
#51365=CARTESIAN_POINT('Ctrl Pts',(18.5276405431088,-1.39610073357796,125.000675380104));
#51366=CARTESIAN_POINT('Ctrl Pts',(19.0931401580165,-1.25842381920182,125.035986467183));
#51367=CARTESIAN_POINT('Ctrl Pts',(19.5513770476802,-0.903101174061878,
125.071166515444));
#51368=CARTESIAN_POINT('Ctrl Pts',(19.8234925261704,-0.393520928653388,
125.106214675531));
#51369=CARTESIAN_POINT('Ctrl Pts',(19.863585446952,0.18057846519377,125.141130187601));
#51370=CARTESIAN_POINT('Ctrl Pts',(19.6664477552688,0.718918428921209,125.175912381995));
#51371=CARTESIAN_POINT('Ctrl Pts',(19.2681597354425,1.12820343239091,125.210560679702));
#51372=CARTESIAN_POINT('Ctrl Pts',(18.7394968083553,1.33829386724977,125.245074592494));
#51373=CARTESIAN_POINT('Ctrl Pts',(18.1733515600056,1.31422440666254,125.279453723019));
#51374=CARTESIAN_POINT('Ctrl Pts',(17.6684072336029,1.06200918227394,125.313697765461));
#51375=CARTESIAN_POINT('Ctrl Pts',(17.3119333434095,0.62727345561428,125.347806505814));
#51376=CARTESIAN_POINT('Ctrl Pts',(17.164703194465,0.0870075502303987,125.381779821996));
#51377=CARTESIAN_POINT('Ctrl Pts',(17.2506394082675,-0.464067284867245,
125.415617683646));
#51378=CARTESIAN_POINT('Ctrl Pts',(17.5529500312885,-0.93010635281992,125.449320152153));
#51379=CARTESIAN_POINT('Ctrl Pts',(18.0173742562096,-1.23080998259887,125.482887380882));
#51380=CARTESIAN_POINT('Ctrl Pts',(18.5619148970354,-1.31525442806852,125.516319615136));
#51381=CARTESIAN_POINT('Ctrl Pts',(19.0913123481237,-1.17050448618906,125.54961719185));
#51382=CARTESIAN_POINT('Ctrl Pts',(19.5137054329361,-0.823554001177106,
125.582780539051));
#51383=CARTESIAN_POINT('Ctrl Pts',(19.7565657136191,-0.336311890299757,
125.615810175785));
#51384=CARTESIAN_POINT('Ctrl Pts',(19.7791421686803,0.205437475860851,125.64870671201));
#51385=CARTESIAN_POINT('Ctrl Pts',(19.5792831503527,0.707131271594729,125.681470848156));
#51386=CARTESIAN_POINT('Ctrl Pts',(19.1934974783569,1.08192650056308,125.714103374504));
#51387=CARTESIAN_POINT('Ctrl Pts',(18.6903000531182,1.26572269937722,125.74660517022));
#51388=CARTESIAN_POINT('Ctrl Pts',(18.1580528586921,1.22811231780654,125.778977203127));
#51389=CARTESIAN_POINT('Ctrl Pts',(17.6894582924859,0.977390643756032,125.811220529498));
#51390=CARTESIAN_POINT('Ctrl Pts',(17.3654249182296,0.55880467658169,125.843336292948));
#51391=CARTESIAN_POINT('Ctrl Pts',(17.2411113552341,0.0464007134562138,
125.875325723779));
#51392=CARTESIAN_POINT('Ctrl Pts',(17.3365525714722,-0.470062155704644,
125.907190137343));
#51393=CARTESIAN_POINT('Ctrl Pts',(17.6334582774054,-0.900821679431447,
125.938930933878));
#51394=CARTESIAN_POINT('Ctrl Pts',(18.078689306533,-1.17169762162142,125.970549597961));
#51395=CARTESIAN_POINT('Ctrl Pts',(18.593754716555,-1.23684923441498,126.002047697117));
#51396=CARTESIAN_POINT('Ctrl Pts',(19.0886338471913,-1.0865147767173,126.033426880753));
#51397=CARTESIAN_POINT('Ctrl Pts',(19.4774918201155,-0.748430497103195,
126.064688878174));
#51398=CARTESIAN_POINT('Ctrl Pts',(19.6935481589647,-0.282732209663939,
126.095835498253));
#51399=CARTESIAN_POINT('Ctrl Pts',(19.7005261381603,0.228725868558277,126.126868628752));
#51400=CARTESIAN_POINT('Ctrl Pts',(19.4987238371462,0.696739517761545,126.157790234506));
#51401=CARTESIAN_POINT('Ctrl Pts',(19.1246955649095,1.04029099805458,126.188602356125));
#51402=CARTESIAN_POINT('Ctrl Pts',(18.6446468213007,1.20055180571536,126.219307107577));
#51403=CARTESIAN_POINT('Ctrl Pts',(18.1427337757278,1.15093580581614,126.24990667576));
#51404=CARTESIAN_POINT('Ctrl Pts',(17.7063324713574,0.901488522300449,126.280403319565));
#51405=CARTESIAN_POINT('Ctrl Pts',(17.4108529526162,0.496892712939118,126.310799367952));
#51406=CARTESIAN_POINT('Ctrl Pts',(17.3067328954843,0.0084812245335301,
126.34109721811));
#51407=CARTESIAN_POINT('Ctrl Pts',(17.4108490145204,-0.47831756693869,126.371299332964));
#51408=CARTESIAN_POINT('Ctrl Pts',(17.7038045321021,-0.878895943230857,
126.401408240409));
#51409=CARTESIAN_POINT('Ctrl Pts',(18.1335240920449,-1.12414442958507,126.431426532286));
#51410=CARTESIAN_POINT('Ctrl Pts',(18.6244919535479,-1.17234924842773,126.461356862258));
#51411=CARTESIAN_POINT('Ctrl Pts',(19.0909970917821,-1.01626672882518,126.491201943604));
#51412=CARTESIAN_POINT('Ctrl Pts',(19.4520665620905,-0.684179402726174,
126.520964546554));
#51413=CARTESIAN_POINT('Ctrl Pts',(19.6454906893739,-0.234786668051046,
126.550647497157));
#51414=CARTESIAN_POINT('Ctrl Pts',(19.6385159835268,0.253149219888882,126.580253676135));
#51415=CARTESIAN_POINT('Ctrl Pts',(19.4333722711128,0.694578566817253,126.609786017081));
#51416=CARTESIAN_POINT('Ctrl Pts',(19.0667063558325,1.01295613554844,126.639247502871));
#51417=CARTESIAN_POINT('Ctrl Pts',(18.6030514946211,1.1534838541102,126.668641164986));
#51418=CARTESIAN_POINT('Ctrl Pts',(18.1234957510667,1.09251755167767,126.697970077986));
#51419=CARTESIAN_POINT('Ctrl Pts',(17.7115308462464,0.841530068193854,126.727237365886));
#51420=CARTESIAN_POINT('Ctrl Pts',(17.4385535098235,0.444964463531077,126.756446186453));
#51421=CARTESIAN_POINT('Ctrl Pts',(17.3515170588706,-0.0276122872710075,
126.785599752877));
#51422=CARTESIAN_POINT('Ctrl Pts',(17.4648884689082,-0.493692017961726,
126.814701285522));
#51423=CARTESIAN_POINT('Ctrl Pts',(17.7582364067503,-0.872180645238306,
126.843754094616));
#51424=CARTESIAN_POINT('Ctrl Pts',(18.1799399597792,-1.09750112430032,126.872761421116));
#51425=CARTESIAN_POINT('Ctrl Pts',(18.6561791423461,-1.13087232076486,126.901726730967));
#51426=CARTESIAN_POINT('Ctrl Pts',(19.1039589342991,-0.967064360638307,
126.930653153623));
#51427=CARTESIAN_POINT('Ctrl Pts',(19.3883902256841,-0.690354148280827,
126.954729317772));
#51428=CARTESIAN_POINT('Ctrl Pts',(19.5332457227074,-0.414056911611768,
126.973973920849));
#51429=CARTESIAN_POINT('Ctrl Pts',(19.6177437769726,-0.113905111418309,
126.993208932229));
#51430=CARTESIAN_POINT('Ctrl Pts',(19.6011038359952,0.281732384417546,127.017234385341));
#51431=CARTESIAN_POINT('Ctrl Pts',(19.3890514321733,0.706565085330299,127.04604027079));
#51432=CARTESIAN_POINT('Ctrl Pts',(19.0223011451343,1.00751421476368,127.074824428941));
#51433=CARTESIAN_POINT('Ctrl Pts',(18.5648792017946,1.13234542273552,127.103590628698));
#51434=CARTESIAN_POINT('Ctrl Pts',(18.0966155583551,1.05950100369092,127.13234222422));
#51435=CARTESIAN_POINT('Ctrl Pts',(17.6990872091144,0.801854248777839,127.161082806753));
#51436=CARTESIAN_POINT('Ctrl Pts',(17.4415305074347,0.404417889894389,127.18981585486));
#51437=CARTESIAN_POINT('Ctrl Pts',(17.3687695530042,-0.0634870235218906,
127.218544916761));
#51438=CARTESIAN_POINT('Ctrl Pts',(17.4934609062107,-0.520295799873725,
127.247273508358));
#51439=CARTESIAN_POINT('Ctrl Pts',(17.7938846953223,-0.886376575644098,
127.276005163098));
#51440=CARTESIAN_POINT('Ctrl Pts',(18.2177247634987,-1.0978765550393,127.304743403475));
#51441=CARTESIAN_POINT('Ctrl Pts',(18.6911508939668,-1.11782834790528,127.333491753923));
#51442=CARTESIAN_POINT('Ctrl Pts',(19.1316465689169,-0.942594483611371,
127.362253727978));
#51443=CARTESIAN_POINT('Ctrl Pts',(19.4623516371648,-0.602527764442204,
127.391032833955));
#51444=CARTESIAN_POINT('Ctrl Pts',(19.6254375334004,-0.156728820867022,
127.419832557726));
#51445=CARTESIAN_POINT('Ctrl Pts',(19.5921943171502,0.317197263638082,127.448656399276));
#51446=CARTESIAN_POINT('Ctrl Pts',(19.368068361135,0.736614311055538,127.477507771776));
#51447=CARTESIAN_POINT('Ctrl Pts',(18.9917822982762,1.02822677014049,127.506390229474));
#51448=CARTESIAN_POINT('Ctrl Pts',(18.5286553795516,1.1408523543525,127.535306988223));
#51449=CARTESIAN_POINT('Ctrl Pts',(18.0593071007243,1.05438854513454,127.564261845145));
#51450=CARTESIAN_POINT('Ctrl Pts',(17.665645179454,0.78337931240486,127.593257348673));
#51451=CARTESIAN_POINT('Ctrl Pts',(17.4166255106301,0.374596672588247,127.622298651964));
#51452=CARTESIAN_POINT('Ctrl Pts',(17.356168808789,-0.10102697056375,127.651385319048));
#51453=CARTESIAN_POINT('Ctrl Pts',(17.4955452283241,-0.560666528004949,
127.680527574784));
#51454=CARTESIAN_POINT('Ctrl Pts',(17.8109503297906,-0.923997881438208,
127.709717292561));
#51455=CARTESIAN_POINT('Ctrl Pts',(18.2483725221223,-1.12713601481138,127.738975362331));
#51456=CARTESIAN_POINT('Ctrl Pts',(18.7311725427411,-1.13411043401417,127.768275574607));
#51457=CARTESIAN_POINT('Ctrl Pts',(19.1762783013378,-0.942422457862223,
127.797675015527));
#51458=CARTESIAN_POINT('Ctrl Pts',(19.5046484170361,-0.585761601815651,
127.827081897376));
#51459=CARTESIAN_POINT('Ctrl Pts',(19.6582495271737,-0.123680562238502,
127.85662756148));
#51460=CARTESIAN_POINT('Ctrl Pts',(19.6201095104048,0.280620801278878,127.881304584504));
#51461=CARTESIAN_POINT('Ctrl Pts',(19.4907597078714,0.572725205601487,127.900977353949));
#51462=CARTESIAN_POINT('Ctrl Pts',(19.3483928135265,0.768967247407983,127.915853796736));
#51463=CARTESIAN_POINT('Ctrl Pts',(19.1686762334047,0.931517072832566,127.930784609013));
#51464=CARTESIAN_POINT('Ctrl Pts',(18.9634686971736,1.051701521621,127.945656286825));
#51465=CARTESIAN_POINT('Ctrl Pts',(18.7395400780403,1.12529086281877,127.960455609962));
#51466=CARTESIAN_POINT('Ctrl Pts',(18.5767277357217,1.14299969027711,127.970442080495));
#51467=CARTESIAN_POINT('Ctrl Pts',(18.491314532458,1.14371857755274,127.975498274504));
#51468=CARTESIAN_POINT('Ctrl Pts',(18.4886857815326,1.24006279342174,112.700349483895));
#51469=CARTESIAN_POINT('Ctrl Pts',(18.350700487512,1.23890142880501,112.7085177809));
#51470=CARTESIAN_POINT('Ctrl Pts',(18.1772861379161,1.21099225659712,112.719338882009));
#51471=CARTESIAN_POINT('Ctrl Pts',(17.9371470941586,1.11768692836503,112.735559070081));
#51472=CARTESIAN_POINT('Ctrl Pts',(17.7502869740318,1.0082123691728,112.749104651932));
#51473=CARTESIAN_POINT('Ctrl Pts',(17.5538963727147,0.830572680386769,112.765421885891));
#51474=CARTESIAN_POINT('Ctrl Pts',(17.3972550616849,0.615007769038441,112.781770658263));
#51475=CARTESIAN_POINT('Ctrl Pts',(17.253907652199,0.291146232712233,112.803582570228));
#51476=CARTESIAN_POINT('Ctrl Pts',(17.2113131548919,-0.157408290328995,
112.830961830784));
#51477=CARTESIAN_POINT('Ctrl Pts',(17.3824904082006,-0.673584584172649,
112.863958155807));
#51478=CARTESIAN_POINT('Ctrl Pts',(17.7519425650394,-1.07558463392321,112.897078373792));
#51479=CARTESIAN_POINT('Ctrl Pts',(18.255676840556,-1.29276968930806,112.930352237627));
#51480=CARTESIAN_POINT('Ctrl Pts',(18.8060692042725,-1.28530683832539,112.963758718116));
#51481=CARTESIAN_POINT('Ctrl Pts',(19.3078619919564,-1.05259089330479,112.997309949318));
#51482=CARTESIAN_POINT('Ctrl Pts',(19.672166717931,-0.633541265410673,113.031000596886));
#51483=CARTESIAN_POINT('Ctrl Pts',(19.8343041249495,-0.0999775951895171,
113.064833380886));
#51484=CARTESIAN_POINT('Ctrl Pts',(19.7640474039292,0.455577886151346,113.09880714741));
#51485=CARTESIAN_POINT('Ctrl Pts',(19.4717972044179,0.935971626992234,113.13292248262));
#51486=CARTESIAN_POINT('Ctrl Pts',(19.0069067899873,1.25642301617407,113.167178934682));
#51487=CARTESIAN_POINT('Ctrl Pts',(18.4493883394344,1.3594620991575,113.201576453895));
#51488=CARTESIAN_POINT('Ctrl Pts',(17.896156579089,1.22525216584098,113.236114632791));
#51489=CARTESIAN_POINT('Ctrl Pts',(17.44416598478,0.875366234347725,113.270793101865));
#51490=CARTESIAN_POINT('Ctrl Pts',(17.1734203958771,0.369351019247229,113.305611329641));
#51491=CARTESIAN_POINT('Ctrl Pts',(17.1328069524393,-0.205403746546834,
113.340568728524));
#51492=CARTESIAN_POINT('Ctrl Pts',(17.3312781873272,-0.748761750970205,
113.375664582924));
#51493=CARTESIAN_POINT('Ctrl Pts',(17.7359495942994,-1.16529115160682,113.410898124736));
#51494=CARTESIAN_POINT('Ctrl Pts',(18.2775596178026,-1.38103864357808,113.44626843028));
#51495=CARTESIAN_POINT('Ctrl Pts',(18.8622737221434,-1.35665630399749,113.48177458993));
#51496=CARTESIAN_POINT('Ctrl Pts',(19.3880357926552,-1.09457855934319,113.517415429957));
#51497=CARTESIAN_POINT('Ctrl Pts',(19.762282781053,-0.63891289156151,113.553189894316));
#51498=CARTESIAN_POINT('Ctrl Pts',(19.9183542097906,-0.0680386023566974,
113.589096658421));
#51499=CARTESIAN_POINT('Ctrl Pts',(19.8273068616531,0.518948612910108,113.62513440713));
#51500=CARTESIAN_POINT('Ctrl Pts',(19.5032854374879,1.01931705204083,113.661301729037));
#51501=CARTESIAN_POINT('Ctrl Pts',(19.0013754975563,1.34488795255941,113.69759704498));
#51502=CARTESIAN_POINT('Ctrl Pts',(18.5070667715635,1.42188430560478,113.727948563529));
#51503=CARTESIAN_POINT('Ctrl Pts',(18.1176199059488,1.35815507053335,113.752292070503));
#51504=CARTESIAN_POINT('Ctrl Pts',(17.7491627514288,1.21499957788935,113.776676870709));
#51505=CARTESIAN_POINT('Ctrl Pts',(17.3596817931078,0.895664735229003,113.807234801998));
#51506=CARTESIAN_POINT('Ctrl Pts',(17.088766042796,0.353119873219169,113.844025336828));
#51507=CARTESIAN_POINT('Ctrl Pts',(17.0629633807845,-0.254681689259876,
113.880935056018));
#51508=CARTESIAN_POINT('Ctrl Pts',(17.2883999286117,-0.821825992495695,
113.917961912365));
#51509=CARTESIAN_POINT('Ctrl Pts',(17.727173455224,-1.24873485756755,113.955103786105));
#51510=CARTESIAN_POINT('Ctrl Pts',(18.303800663237,-1.45983756465867,113.99235852218));
#51511=CARTESIAN_POINT('Ctrl Pts',(18.9181754346717,-1.41687241297771,114.029723858283));
#51512=CARTESIAN_POINT('Ctrl Pts',(19.4629905317816,-1.1258760124666,114.06719743653));
#51513=CARTESIAN_POINT('Ctrl Pts',(19.8424979033294,-0.636345183090518,
114.10477690674));
#51514=CARTESIAN_POINT('Ctrl Pts',(19.9893577348222,-0.0328548365392322,
114.142459719485));
#51515=CARTESIAN_POINT('Ctrl Pts',(19.8766107184348,0.579636771896997,114.180243394414));
#51516=CARTESIAN_POINT('Ctrl Pts',(19.5226143125954,1.09396896256936,114.218125277347));
#51517=CARTESIAN_POINT('Ctrl Pts',(18.9880576434996,1.4196814246808,114.256102695897));
#51518=CARTESIAN_POINT('Ctrl Pts',(18.3655758455969,1.49883229295896,114.294172904322));
#51519=CARTESIAN_POINT('Ctrl Pts',(17.7636357733795,1.31639721669226,114.332333090623));
#51520=CARTESIAN_POINT('Ctrl Pts',(17.2876293894219,0.903070126436221,114.370580382322));
#51521=CARTESIAN_POINT('Ctrl Pts',(17.021381596707,0.330105442854477,114.408911856729));
#51522=CARTESIAN_POINT('Ctrl Pts',(17.0123615413044,-0.302963995370305,
114.447324511126));
#51523=CARTESIAN_POINT('Ctrl Pts',(17.2632246426998,-0.885701130781865,
114.485815331495));
#51524=CARTESIAN_POINT('Ctrl Pts',(17.7311221924098,-1.31595137471215,114.524381167031));
#51525=CARTESIAN_POINT('Ctrl Pts',(18.3351011606019,-1.51799826919431,114.563018976257));
#51526=CARTESIAN_POINT('Ctrl Pts',(18.8641772955744,-1.46590872316032,114.595274296623));
#51527=CARTESIAN_POINT('Ctrl Pts',(19.2475290597062,-1.29717065284742,114.621111390481));
#51528=CARTESIAN_POINT('Ctrl Pts',(19.587930934106,-1.05255012654514,114.646969774733));
#51529=CARTESIAN_POINT('Ctrl Pts',(19.9027887485453,-0.622010716970455,
114.679331455281));
#51530=CARTESIAN_POINT('Ctrl Pts',(20.0367268988523,0.00492783437249169,
114.718224488104));
#51531=CARTESIAN_POINT('Ctrl Pts',(19.902771949599,0.632745745648799,114.757172921015));
#51532=CARTESIAN_POINT('Ctrl Pts',(19.5235337266645,1.1518069086034,114.796173482906));
#51533=CARTESIAN_POINT('Ctrl Pts',(18.9646746735623,1.47107637085436,114.835222648074));
#51534=CARTESIAN_POINT('Ctrl Pts',(18.3234147425032,1.53431878643646,114.874317010436));
#51535=CARTESIAN_POINT('Ctrl Pts',(17.7115872791309,1.32988381647799,114.913452982608));
#51536=CARTESIAN_POINT('Ctrl Pts',(17.236199074676,0.892983590472233,114.95262716011));
#51537=CARTESIAN_POINT('Ctrl Pts',(16.9804303870928,0.299434632784239,114.991835755524));
#51538=CARTESIAN_POINT('Ctrl Pts',(16.9885500629826,-0.275357498986949,
115.026715644867));
#51539=CARTESIAN_POINT('Ctrl Pts',(17.1661753238746,-0.739792594872671,
115.057252816654));
#51540=CARTESIAN_POINT('Ctrl Pts',(17.3582591195826,-0.995315857598361,
115.076892896405));
#51541=CARTESIAN_POINT('Ctrl Pts',(17.5129117285239,-1.1393035260029,115.089988598705));
#51542=CARTESIAN_POINT('Ctrl Pts',(17.5949882602575,-1.20577477857244,115.096537396983));
#51543=CARTESIAN_POINT('Ctrl Pts',(17.6816102396563,-1.2662793811424,115.103086599594));
#51544=CARTESIAN_POINT('Ctrl Pts',(17.8628170287837,-1.37497559618221,115.116186841398));
#51545=CARTESIAN_POINT('Ctrl Pts',(18.1617769542351,-1.48907715427518,115.135839934973));
#51546=CARTESIAN_POINT('Ctrl Pts',(18.5869931130475,-1.52497006090699,115.162053457002));
#51547=CARTESIAN_POINT('Ctrl Pts',(19.0057443231637,-1.44168146613633,115.188272628449));
#51548=CARTESIAN_POINT('Ctrl Pts',(19.3849508796851,-1.2457392947455,115.214498469562));
#51549=CARTESIAN_POINT('Ctrl Pts',(19.6955043477239,-0.952325970828538,
115.240728071787));
#51550=CARTESIAN_POINT('Ctrl Pts',(19.9120727588161,-0.58453124815665,115.266961861401));
#51551=CARTESIAN_POINT('Ctrl Pts',(20.0554335071329,-0.0328780904536275,
115.30194294116));
#51552=CARTESIAN_POINT('Ctrl Pts',(19.9573549390358,0.544872472127717,115.336926751788));
#51553=CARTESIAN_POINT('Ctrl Pts',(19.6792725553991,0.959018990798004,115.367536446853));
#51554=CARTESIAN_POINT('Ctrl Pts',(19.4770068532755,1.15607677108951,115.385026263675));
#51555=CARTESIAN_POINT('Ctrl Pts',(19.2485905147621,1.32287773637073,115.402515663463));
#51556=CARTESIAN_POINT('Ctrl Pts',(19.0214001924108,1.42466933279182,115.417817762452));
#51557=CARTESIAN_POINT('Ctrl Pts',(18.8160770510847,1.47600201291175,115.430931956767));
#51558=CARTESIAN_POINT('Ctrl Pts',(18.7119660101375,1.49445958327978,115.437488986517));
#51559=CARTESIAN_POINT('Ctrl Pts',(18.6243012018012,1.50374532227516,115.442952840385));
#51560=CARTESIAN_POINT('Ctrl Pts',(18.5539105066717,1.50738308247896,115.44732397057));
#51561=CARTESIAN_POINT('Ctrl Pts',(18.2682087517811,1.51284780011209,115.465050305463));
#51562=CARTESIAN_POINT('Ctrl Pts',(17.7497170731845,1.38044204374156,115.497218908285));
#51563=CARTESIAN_POINT('Ctrl Pts',(17.30801070384,0.970768685607363,115.53345638968));
#51564=CARTESIAN_POINT('Ctrl Pts',(17.1114916776926,0.601056660964444,115.559330092168));
#51565=CARTESIAN_POINT('Ctrl Pts',(17.0446027454294,0.402885159945071,115.572263924207));
#51566=CARTESIAN_POINT('Ctrl Pts',(17.0117248103742,0.239205340866807,115.582609001927));
#51567=CARTESIAN_POINT('Ctrl Pts',(16.9724616627671,-0.0923162242471636,
115.60329739301));
#51568=CARTESIAN_POINT('Ctrl Pts',(17.0696480425108,-0.642532402723225,
115.636900798108));
#51569=CARTESIAN_POINT('Ctrl Pts',(17.5517663934372,-1.24713786909881,115.683388146918));
#51570=CARTESIAN_POINT('Ctrl Pts',(18.2042007282122,-1.5217813743094,115.725958665169));
#51571=CARTESIAN_POINT('Ctrl Pts',(18.8381530262514,-1.49751551729433,115.764620805466));
#51572=CARTESIAN_POINT('Ctrl Pts',(19.3608147157338,-1.26964475423224,115.799384658136));
#51573=CARTESIAN_POINT('Ctrl Pts',(19.7637360954163,-0.866573811032385,
115.834113791312));
#51574=CARTESIAN_POINT('Ctrl Pts',(19.9532575329137,-0.431912285220216,
115.863024225621));
#51575=CARTESIAN_POINT('Ctrl Pts',(20.0019084566828,-0.0608512365984601,
115.886132317853));
#51576=CARTESIAN_POINT('Ctrl Pts',(19.9862463403857,0.219126166715986,115.903454009194));
#51577=CARTESIAN_POINT('Ctrl Pts',(19.9299939358539,0.44586883885173,115.917879168524));
#51578=CARTESIAN_POINT('Ctrl Pts',(19.8603226080054,0.618480030546314,115.929414262885));
#51579=CARTESIAN_POINT('Ctrl Pts',(19.732335428513,0.866591475554719,115.946711763469));
#51580=CARTESIAN_POINT('Ctrl Pts',(19.4548716729342,1.1889197996581,115.972636463467));
#51581=CARTESIAN_POINT('Ctrl Pts',(18.9541280189803,1.45349838246967,116.007156800886));
#51582=CARTESIAN_POINT('Ctrl Pts',(18.3921287206258,1.51673596305252,116.041627931309));
#51583=CARTESIAN_POINT('Ctrl Pts',(17.98308129254,1.40706783893502,116.06744280953));
#51584=CARTESIAN_POINT('Ctrl Pts',(17.7390445958302,1.2749731316633,116.084636072118));
#51585=CARTESIAN_POINT('Ctrl Pts',(17.5852912916948,1.1722752978984,116.096093986087));
#51586=CARTESIAN_POINT('Ctrl Pts',(17.3432828327208,0.956086398655082,116.116132394891));
#51587=CARTESIAN_POINT('Ctrl Pts',(17.1809589926931,0.698076633103147,116.134717679963));
#51588=CARTESIAN_POINT('Ctrl Pts',(17.1020431840008,0.481651667190302,116.149000182525));
#51589=CARTESIAN_POINT('Ctrl Pts',(17.0813292455805,0.415767578672489,116.153283932293));
#51590=CARTESIAN_POINT('Ctrl Pts',(17.0637859639785,0.348956125741941,116.157566823568));
#51591=CARTESIAN_POINT('Ctrl Pts',(17.0493670996022,0.281437463958633,116.16184876527));
#51592=CARTESIAN_POINT('Ctrl Pts',(17.038100686667,0.213320935068083,116.166129828349));
#51593=CARTESIAN_POINT('Ctrl Pts',(17.027418537701,0.121921946398209,116.171836683298));
#51594=CARTESIAN_POINT('Ctrl Pts',(17.0154022607627,-0.131006355748056,
116.187525750009));
#51595=CARTESIAN_POINT('Ctrl Pts',(17.0937079736478,-0.544356912453348,
116.213169665427));
#51596=CARTESIAN_POINT('Ctrl Pts',(17.3916931786148,-1.01842990090603,116.247299944086));
#51597=CARTESIAN_POINT('Ctrl Pts',(17.8414160362638,-1.35021757910078,116.281365294444));
#51598=CARTESIAN_POINT('Ctrl Pts',(18.38024698509,-1.49448019673828,116.315364296159));
#51599=CARTESIAN_POINT('Ctrl Pts',(18.9333558500912,-1.43205814835875,116.349294475226));
#51600=CARTESIAN_POINT('Ctrl Pts',(19.4244998765879,-1.17237925887462,116.383154182635));
#51601=CARTESIAN_POINT('Ctrl Pts',(19.7055325005771,-0.845552308419617,
116.409432645791));
#51602=CARTESIAN_POINT('Ctrl Pts',(19.8402281106805,-0.574341496855494,
116.428175851723));
#51603=CARTESIAN_POINT('Ctrl Pts',(19.9200054022093,-0.345954669915418,
116.443158705062));
#51604=CARTESIAN_POINT('Ctrl Pts',(19.9840539280259,0.0748890717238647,
116.469349942729));
#51605=CARTESIAN_POINT('Ctrl Pts',(19.8458498456958,0.679996931929124,116.506679814718));
#51606=CARTESIAN_POINT('Ctrl Pts',(19.3540620896253,1.23670047743049,116.55133441875));
#51607=CARTESIAN_POINT('Ctrl Pts',(18.6584618742995,1.48956129229607,116.595843150702));
#51608=CARTESIAN_POINT('Ctrl Pts',(17.9289213122935,1.37932213376007,116.640202113418));
#51609=CARTESIAN_POINT('Ctrl Pts',(17.4285805916008,0.999858721838042,116.677960635258));
#51610=CARTESIAN_POINT('Ctrl Pts',(17.1711328116473,0.561567611548129,116.709185478337));
#51611=CARTESIAN_POINT('Ctrl Pts',(17.0359126623898,0.0415724183980224,
116.74217956973));
#51612=CARTESIAN_POINT('Ctrl Pts',(17.1515940470276,-0.637998239122351,
116.783294411513));
#51613=CARTESIAN_POINT('Ctrl Pts',(17.7010550860578,-1.25205133614912,116.832422554598));
#51614=CARTESIAN_POINT('Ctrl Pts',(18.4894062498268,-1.47858967259486,116.881336428698));
#51615=CARTESIAN_POINT('Ctrl Pts',(19.2738940695048,-1.25207829303643,116.9300315906));
#51616=CARTESIAN_POINT('Ctrl Pts',(19.8153307145306,-0.645520014193124,
116.978503807804));
#51617=CARTESIAN_POINT('Ctrl Pts',(19.9274909343049,0.0191068948937147,
117.018708427583));
#51618=CARTESIAN_POINT('Ctrl Pts',(19.7960939552228,0.52415495559139,117.050756767602));
#51619=CARTESIAN_POINT('Ctrl Pts',(19.5981826748897,0.860577176378632,117.074735160752));
#51620=CARTESIAN_POINT('Ctrl Pts',(19.314819314541,1.1276909269993,117.09865491716));
#51621=CARTESIAN_POINT('Ctrl Pts',(18.8549396626615,1.36629811978027,117.130469699018));
#51622=CARTESIAN_POINT('Ctrl Pts',(18.1917040784683,1.40331982158644,117.170090005227));
#51623=CARTESIAN_POINT('Ctrl Pts',(17.4975691912014,1.01895490957414,117.217394838748));
#51624=CARTESIAN_POINT('Ctrl Pts',(17.1163543952753,0.327987168551171,117.264457516944));
#51625=CARTESIAN_POINT('Ctrl Pts',(17.160929761522,-0.455921789738659,117.311275902367));
#51626=CARTESIAN_POINT('Ctrl Pts',(17.6133690361685,-1.0925258757231,117.357848055034));
#51627=CARTESIAN_POINT('Ctrl Pts',(18.3313062938161,-1.38928284881341,117.404172384602));
#51628=CARTESIAN_POINT('Ctrl Pts',(19.0929708141868,-1.25926708655467,117.450247571127));
#51629=CARTESIAN_POINT('Ctrl Pts',(19.6655860734287,-0.746753373827336,
117.496072609338));
#51630=CARTESIAN_POINT('Ctrl Pts',(19.8765949471167,-0.0121828500468043,
117.54164678921));
#51631=CARTESIAN_POINT('Ctrl Pts',(19.6656116013329,0.718007452175992,117.586969706763));
#51632=CARTESIAN_POINT('Ctrl Pts',(19.1016254377219,1.22121959599358,117.632041258556));
#51633=CARTESIAN_POINT('Ctrl Pts',(18.3605130926681,1.34653801701873,117.676861646409));
#51634=CARTESIAN_POINT('Ctrl Pts',(17.6702033501949,1.05996166417369,117.721431373627));
#51635=CARTESIAN_POINT('Ctrl Pts',(17.2405952007114,0.453464700753241,117.765751245736));
#51636=CARTESIAN_POINT('Ctrl Pts',(17.1997363628675,-0.284476148782968,
117.809822372049));
#51637=CARTESIAN_POINT('Ctrl Pts',(17.5557499811275,-0.927408650891648,
117.853646158814));
#51638=CARTESIAN_POINT('Ctrl Pts',(18.1956275936224,-1.28041361919324,117.897224312267));
#51639=CARTESIAN_POINT('Ctrl Pts',(18.921197736518,-1.23907672512662,117.940558832347));
#51640=CARTESIAN_POINT('Ctrl Pts',(19.5101916907598,-0.820458777550031,
117.983652023246));
#51641=CARTESIAN_POINT('Ctrl Pts',(19.7848036770107,-0.156223199417709,
118.026506456872));
#51642=CARTESIAN_POINT('Ctrl Pts',(19.6843949739844,0.430767380595849,118.062021937999));
#51643=CARTESIAN_POINT('Ctrl Pts',(19.4275325513615,0.813160885753741,118.09031793704));
#51644=CARTESIAN_POINT('Ctrl Pts',(19.0770973083296,1.11031666639859,118.11853700952));
#51645=CARTESIAN_POINT('Ctrl Pts',(18.5109814174046,1.27316147481377,118.153667438987));
#51646=CARTESIAN_POINT('Ctrl Pts',(17.8353641889859,1.07788215725043,118.195598493365));
#51647=CARTESIAN_POINT('Ctrl Pts',(17.3697015237894,0.556044035321663,118.237307932148));
#51648=CARTESIAN_POINT('Ctrl Pts',(17.2536309754749,-0.13005972066861,118.278800089396));
#51649=CARTESIAN_POINT('Ctrl Pts',(17.519011887563,-0.76940485670393,118.320079435902));
#51650=CARTESIAN_POINT('Ctrl Pts',(18.0810167923109,-1.16759070881662,118.361150774145));
#51651=CARTESIAN_POINT('Ctrl Pts',(18.7653205420581,-1.20552740953108,118.402019112245));
#51652=CARTESIAN_POINT('Ctrl Pts',(19.3620426768933,-0.875236261419451,
118.44268974516));
#51653=CARTESIAN_POINT('Ctrl Pts',(19.6899929427312,-0.280852314250413,
118.483168136373));
#51654=CARTESIAN_POINT('Ctrl Pts',(19.6517027034045,0.393658905744708,118.523460105995));
#51655=CARTESIAN_POINT('Ctrl Pts',(19.262049671239,0.94218480231557,118.563571483349));
#51656=CARTESIAN_POINT('Ctrl Pts',(18.7464141286224,1.15520066927372,118.596852495218));
#51657=CARTESIAN_POINT('Ctrl Pts',(18.3143388197521,1.14217861007577,118.623393153417));
#51658=CARTESIAN_POINT('Ctrl Pts',(18.0062641848802,1.04426592123211,118.643257711825));
#51659=CARTESIAN_POINT('Ctrl Pts',(17.737911282933,0.864729841538294,118.663081671285));
#51660=CARTESIAN_POINT('Ctrl Pts',(17.5301393468996,0.618703669685291,118.682866420824));
#51661=CARTESIAN_POINT('Ctrl Pts',(17.39886715547,0.325178671794981,118.702612273734));
#51662=CARTESIAN_POINT('Ctrl Pts',(17.3540635143272,0.00751232992213948,
118.722320588503));
#51663=CARTESIAN_POINT('Ctrl Pts',(17.3988571968852,-0.309665669008213,
118.741991793837));
#51664=CARTESIAN_POINT('Ctrl Pts',(17.5077328986331,-0.552719890765469,
118.758354742027));
#51665=CARTESIAN_POINT('Ctrl Pts',(17.6323989098259,-0.723375778033712,
118.77142712254));
#51666=CARTESIAN_POINT('Ctrl Pts',(17.7796050666785,-0.874496856491821,
118.784488585854));
#51667=CARTESIAN_POINT('Ctrl Pts',(18.0883757023863,-1.0816829350278,118.807315342415));
#51668=CARTESIAN_POINT('Ctrl Pts',(18.6258850389041,-1.17297338013441,118.839842374316));
#51669=CARTESIAN_POINT('Ctrl Pts',(19.2288585553104,-0.922879583318754,
118.878749049984));
#51670=CARTESIAN_POINT('Ctrl Pts',(19.542020048084,-0.480800009490288,118.911072799632));
#51671=CARTESIAN_POINT('Ctrl Pts',(19.6130019723937,-0.11988951021874,118.933651657005));
#51672=CARTESIAN_POINT('Ctrl Pts',(19.6102239348255,0.0882078318904775,
118.946540021196));
#51673=CARTESIAN_POINT('Ctrl Pts',(19.5782633862719,0.294095923696726,118.959420392155));
#51674=CARTESIAN_POINT('Ctrl Pts',(19.4847100541208,0.538407016934738,118.975504309447));
#51675=CARTESIAN_POINT('Ctrl Pts',(19.2335825206301,0.873421396581657,119.001206235821));
#51676=CARTESIAN_POINT('Ctrl Pts',(18.7630625129791,1.133423759209,119.033274471397));
#51677=CARTESIAN_POINT('Ctrl Pts',(18.1200833960856,1.09710962449598,119.071670495069));
#51678=CARTESIAN_POINT('Ctrl Pts',(17.5960924873024,0.725093259873059,119.109988487022));
#51679=CARTESIAN_POINT('Ctrl Pts',(17.3918121525979,0.231296298510037,119.14186251893));
#51680=CARTESIAN_POINT('Ctrl Pts',(17.4043290798831,-0.183311036107097,
119.167330765526));
#51681=CARTESIAN_POINT('Ctrl Pts',(17.4825892496997,-0.4299892222351,119.183237212406));
#51682=CARTESIAN_POINT('Ctrl Pts',(17.572039140911,-0.586160414573573,119.194365338264));
#51683=CARTESIAN_POINT('Ctrl Pts',(17.6318745222132,-0.669372754950965,
119.200722868091));
#51684=CARTESIAN_POINT('Ctrl Pts',(17.6975224916197,-0.748188779439941,
119.207079373284));
#51685=CARTESIAN_POINT('Ctrl Pts',(17.7895488799981,-0.837670708203213,
119.215023530388));
#51686=CARTESIAN_POINT('Ctrl Pts',(17.9553267231429,-0.958868977804718,
119.227729237297));
#51687=CARTESIAN_POINT('Ctrl Pts',(18.1912383187694,-1.06444361121362,119.243605397494));
#51688=CARTESIAN_POINT('Ctrl Pts',(18.4982090921703,-1.10776721271402,119.262646233441));
#51689=CARTESIAN_POINT('Ctrl Pts',(18.80502032819,-1.06443802417128,119.281678727518));
#51690=CARTESIAN_POINT('Ctrl Pts',(19.0877383109047,-0.937929437452661,
119.300703044015));
#51691=CARTESIAN_POINT('Ctrl Pts',(19.3242981547535,-0.738152546180218,
119.319721102764));
#51692=CARTESIAN_POINT('Ctrl Pts',(19.4962591468119,-0.480795071701003,
119.338732993694));
#51693=CARTESIAN_POINT('Ctrl Pts',(19.5902349861746,-0.185930364314395,
119.357741177416));
#51694=CARTESIAN_POINT('Ctrl Pts',(19.5988995449809,0.12332837974993,119.376744922794));
#51695=CARTESIAN_POINT('Ctrl Pts',(19.5345226003805,0.372995262793573,119.392580513945));
#51696=CARTESIAN_POINT('Ctrl Pts',(19.4430256832353,0.556105224782065,119.405247530558));
#51697=CARTESIAN_POINT('Ctrl Pts',(19.2980649158877,0.766998982846697,119.421081592547));
#51698=CARTESIAN_POINT('Ctrl Pts',(19.0156700351553,0.998794457158363,119.44324895863));
#51699=CARTESIAN_POINT('Ctrl Pts',(18.5624053105446,1.12252034366067,119.47175321809));
#51700=CARTESIAN_POINT('Ctrl Pts',(18.0980570899233,1.05032299384497,119.500264531386));
#51701=CARTESIAN_POINT('Ctrl Pts',(17.7035292914276,0.79466914998275,119.528786584334));
#51702=CARTESIAN_POINT('Ctrl Pts',(17.447699261081,0.399967002624156,119.557322986304));
#51703=CARTESIAN_POINT('Ctrl Pts',(17.3753531548392,-0.0650758120843595,
119.585877532102));
#51704=CARTESIAN_POINT('Ctrl Pts',(17.4993233063343,-0.519496847790021,
119.614453598271));
#51705=CARTESIAN_POINT('Ctrl Pts',(17.7485568416745,-0.82315833221159,119.638288394535));
#51706=CARTESIAN_POINT('Ctrl Pts',(18.0094705396139,-0.989327736740765,
119.657370307388));
#51707=CARTESIAN_POINT('Ctrl Pts',(18.2992856072175,-1.09795570141558,119.676462853576));
#51708=CARTESIAN_POINT('Ctrl Pts',(18.6926161209824,-1.11462209520415,119.700348615935));
#51709=CARTESIAN_POINT('Ctrl Pts',(19.132174381934,-0.939774985844624,119.729047762112));
#51710=CARTESIAN_POINT('Ctrl Pts',(19.4624379375494,-0.600228903798103,
119.757786510277));
#51711=CARTESIAN_POINT('Ctrl Pts',(19.6254642184456,-0.154710493808823,
119.786568470845));
#51712=CARTESIAN_POINT('Ctrl Pts',(19.5922506981539,0.319294076080361,119.815397085605));
#51713=CARTESIAN_POINT('Ctrl Pts',(19.3679519164038,0.739126592198824,119.844275847045));
#51714=CARTESIAN_POINT('Ctrl Pts',(18.9910313338467,1.03127863586338,119.873208155992));
#51715=CARTESIAN_POINT('Ctrl Pts',(18.526768166279,1.1442132821202,119.902197433971));
#51716=CARTESIAN_POINT('Ctrl Pts',(18.0558482748031,1.05752607607186,119.931246981343));
#51717=CARTESIAN_POINT('Ctrl Pts',(17.726496041802,0.830759475988353,119.955507997517));
#51718=CARTESIAN_POINT('Ctrl Pts',(17.5354344117903,0.580091248025318,119.974950233318));
#51719=CARTESIAN_POINT('Ctrl Pts',(17.4002338592083,0.29498975660088,119.994415199709));
#51720=CARTESIAN_POINT('Ctrl Pts',(17.3495085645331,-0.103555383199835,
120.018790389193));
#51721=CARTESIAN_POINT('Ctrl Pts',(17.4897005229253,-0.566111876871723,
120.048113816961));
#51722=CARTESIAN_POINT('Ctrl Pts',(17.8073958110046,-0.932013831621567,
120.077513669291));
#51723=CARTESIAN_POINT('Ctrl Pts',(18.2480282367772,-1.13680697021833,120.106992966317));
#51724=CARTESIAN_POINT('Ctrl Pts',(18.7352313285216,-1.14378430035558,120.136554771527));
#51725=CARTESIAN_POINT('Ctrl Pts',(19.1840902814294,-0.950608003668691,
120.1662020226));
#51726=CARTESIAN_POINT('Ctrl Pts',(19.5158873892962,-0.589875672534864,
120.195937638644));
#51727=CARTESIAN_POINT('Ctrl Pts',(19.671889057115,-0.123661189251937,120.22576445635));
#51728=CARTESIAN_POINT('Ctrl Pts',(19.623714661444,0.367152098317012,120.255685262371));
#51729=CARTESIAN_POINT('Ctrl Pts',(19.3784858113755,0.796867932693748,120.285702774258));
#51730=CARTESIAN_POINT('Ctrl Pts',(18.9778103881022,1.08991323854088,120.315819647296));
#51731=CARTESIAN_POINT('Ctrl Pts',(18.490745518226,1.19410168075579,120.346038467292));
#51732=CARTESIAN_POINT('Ctrl Pts',(18.0019208947732,1.0899089270007,120.376361751047));
#51733=CARTESIAN_POINT('Ctrl Pts',(17.5968617879682,0.794109542044404,120.406791944027));
#51734=CARTESIAN_POINT('Ctrl Pts',(17.347051270975,0.357102672662465,120.437331420421));
#51735=CARTESIAN_POINT('Ctrl Pts',(17.2973371287444,-0.145653526217233,
120.467982479992));
#51736=CARTESIAN_POINT('Ctrl Pts',(17.4578978561675,-0.626646770663367,
120.498747346768));
#51737=CARTESIAN_POINT('Ctrl Pts',(17.8022046733259,-1.00151876106162,120.529628166802));
#51738=CARTESIAN_POINT('Ctrl Pts',(18.2713816533395,-1.2038382914039,120.56062700755));
#51739=CARTESIAN_POINT('Ctrl Pts',(18.7842526924098,-1.19685517031873,120.591745857205));
#51740=CARTESIAN_POINT('Ctrl Pts',(19.2513645194326,-0.980158514937333,
120.622986622443));
#51741=CARTESIAN_POINT('Ctrl Pts',(19.5905678372684,-0.590034427104998,
120.654351127325));
#51742=CARTESIAN_POINT('Ctrl Pts',(19.7414461342557,-0.0934120172357776,
120.685841110659));
#51743=CARTESIAN_POINT('Ctrl Pts',(19.6760617503497,0.423601688996781,120.71745822783));
#51744=CARTESIAN_POINT('Ctrl Pts',(19.404107616491,0.870629407224791,120.749204045237));
#51745=CARTESIAN_POINT('Ctrl Pts',(18.9715208516985,1.16881187603194,120.781080048323));
#51746=CARTESIAN_POINT('Ctrl Pts',(18.4527393308266,1.26469201462238,120.813087622212));
#51747=CARTESIAN_POINT('Ctrl Pts',(17.9379142663286,1.13980835377827,120.845228084342));
#51748=CARTESIAN_POINT('Ctrl Pts',(17.5172493454425,0.814174010463595,120.877502620948));
#51749=CARTESIAN_POINT('Ctrl Pts',(17.2652262451152,0.343182535559932,120.909912404771));
#51750=CARTESIAN_POINT('Ctrl Pts',(17.2273959740802,-0.191955731854894,
120.942458370174));
#51751=CARTESIAN_POINT('Ctrl Pts',(17.3660099011979,-0.571412507180306,
120.966970834626));
#51752=CARTESIAN_POINT('Ctrl Pts',(17.5184864903043,-0.787587395398978,
120.983355475166));
#51753=CARTESIAN_POINT('Ctrl Pts',(17.6347010321129,-0.920420644721155,
120.994290222211));
#51754=CARTESIAN_POINT('Ctrl Pts',(17.8733381436317,-1.11944341903204,121.013456130434));
#51755=CARTESIAN_POINT('Ctrl Pts',(18.2938200015906,-1.28705511872534,121.040922810645));
#51756=CARTESIAN_POINT('Ctrl Pts',(18.838962756471,-1.26431650933352,121.074022238662));
#51757=CARTESIAN_POINT('Ctrl Pts',(19.3292777630611,-1.01994040665058,121.107261676011));
#51758=CARTESIAN_POINT('Ctrl Pts',(19.6785157529131,-0.594786234672817,
121.140641575335));
#51759=CARTESIAN_POINT('Ctrl Pts',(19.8242377305752,-0.061848242086873,
121.174162316278));
#51760=CARTESIAN_POINT('Ctrl Pts',(19.7392267053303,0.486436575583768,121.20782417147));
#51761=CARTESIAN_POINT('Ctrl Pts',(19.4364151393894,0.954128542250682,121.241627324197));
#51762=CARTESIAN_POINT('Ctrl Pts',(18.9670347240106,1.25861868234264,121.275571858454));
#51763=CARTESIAN_POINT('Ctrl Pts',(18.4119209874691,1.3451928655867,121.309657764006));
#51764=CARTESIAN_POINT('Ctrl Pts',(17.8676162900118,1.19687069039815,121.34388493345));
#51765=CARTESIAN_POINT('Ctrl Pts',(17.4295680364872,0.837690818648143,121.378253164648));
#51766=CARTESIAN_POINT('Ctrl Pts',(17.1753947118292,0.328842988621187,121.412762158879));
#51767=CARTESIAN_POINT('Ctrl Pts',(17.1511288723051,-0.241752018640547,
121.447411523291));
#51768=CARTESIAN_POINT('Ctrl Pts',(17.3628888947757,-0.77463506048684,121.482200766943));
#51769=CARTESIAN_POINT('Ctrl Pts',(17.7754799049959,-1.17614877543075,121.517129308824));
#51770=CARTESIAN_POINT('Ctrl Pts',(18.3182280438042,-1.37490813354109,121.552196464719));
#51771=CARTESIAN_POINT('Ctrl Pts',(18.897088341648,-1.33448709779315,121.587401473303));
#51772=CARTESIAN_POINT('Ctrl Pts',(19.410942275329,-1.06009788899736,121.622743447905));
#51773=CARTESIAN_POINT('Ctrl Pts',(19.7692799982594,-0.597977854521384,
121.658221467788));
#51774=CARTESIAN_POINT('Ctrl Pts',(19.9081358825043,-0.0276549104963941,
121.693834408962));
#51775=CARTESIAN_POINT('Ctrl Pts',(19.8015290711147,0.551829178738792,121.729581235412));
#51776=CARTESIAN_POINT('Ctrl Pts',(19.4663014352217,1.03901557989597,121.765460617446));
#51777=CARTESIAN_POINT('Ctrl Pts',(18.9594683704855,1.34791861935948,121.801471275704));
#51778=CARTESIAN_POINT('Ctrl Pts',(18.3685489456073,1.4231309693145,121.837611797694));
#51779=CARTESIAN_POINT('Ctrl Pts',(17.7964224040695,1.2498108864466,121.873880663349));
#51780=CARTESIAN_POINT('Ctrl Pts',(17.343411761646,0.856551976471352,121.910276301795));
#51781=CARTESIAN_POINT('Ctrl Pts',(17.0896693094759,0.310691435299757,121.946797039564));
#51782=CARTESIAN_POINT('Ctrl Pts',(17.0809859345148,-0.293233463282239,
121.983441096799));
#51783=CARTESIAN_POINT('Ctrl Pts',(17.3205246799805,-0.849870499306589,
122.020206666278));
#51784=CARTESIAN_POINT('Ctrl Pts',(17.7679800867644,-1.26145256297933,122.057091786186));
#51785=CARTESIAN_POINT('Ctrl Pts',(18.3463570362798,-1.45498776189057,122.09409447297));
#51786=CARTESIAN_POINT('Ctrl Pts',(18.9552323067948,-1.39521898177386,122.131212644739));
#51787=CARTESIAN_POINT('Ctrl Pts',(19.4882105420212,-1.09104109063806,122.16844410693));
#51788=CARTESIAN_POINT('Ctrl Pts',(19.8515424108103,-0.594221675970028,
122.205786668318));
#51789=CARTESIAN_POINT('Ctrl Pts',(19.9806313833143,0.00942427040184544,
122.24323795134));
#51790=CARTESIAN_POINT('Ctrl Pts',(19.8515388043119,0.614855844550354,122.280795635654));
#51791=CARTESIAN_POINT('Ctrl Pts',(19.4853987313484,1.11614759069681,122.318457157599));
#51792=CARTESIAN_POINT('Ctrl Pts',(18.945004615623,1.42498917337475,122.356220138897));
#51793=CARTESIAN_POINT('Ctrl Pts',(18.3239615977549,1.48632115394554,122.394081816335));
#51794=CARTESIAN_POINT('Ctrl Pts',(17.730540856481,1.28815607788699,122.43203962541));
#51795=CARTESIAN_POINT('Ctrl Pts',(17.2686808444291,0.863809782588366,122.470090788431));
#51796=CARTESIAN_POINT('Ctrl Pts',(17.0198424256365,0.286534217812077,122.508232510253));
#51797=CARTESIAN_POINT('Ctrl Pts',(17.0275509599641,-0.273612269369176,
122.542214254841));
#51798=CARTESIAN_POINT('Ctrl Pts',(17.200985856733,-0.726414318936751,122.572003192732));
#51799=CARTESIAN_POINT('Ctrl Pts',(17.533930302551,-1.17071941096088,122.60609683765));
#51800=CARTESIAN_POINT('Ctrl Pts',(18.1603244553639,-1.51749147705401,122.648803589497));
#51801=CARTESIAN_POINT('Ctrl Pts',(19.0208668383675,-1.4694521284666,122.700188190209));
#51802=CARTESIAN_POINT('Ctrl Pts',(19.7255038627886,-0.969775365785065,
122.751701753606));
#51803=CARTESIAN_POINT('Ctrl Pts',(20.057165664497,-0.169954192248215,122.803336782717));
#51804=CARTESIAN_POINT('Ctrl Pts',(19.9120558026029,0.685817564794368,122.855085508656));
#51805=CARTESIAN_POINT('Ctrl Pts',(19.4292974339625,1.22598318348634,122.898297694433));
#51806=CARTESIAN_POINT('Ctrl Pts',(18.9142363313226,1.45527724361131,122.932916381728));
#51807=CARTESIAN_POINT('Ctrl Pts',(18.5110045428195,1.51276370728313,122.957941335571));
#51808=CARTESIAN_POINT('Ctrl Pts',(18.1227813242447,1.46364271968411,122.982023454891));
#51809=CARTESIAN_POINT('Ctrl Pts',(17.6559380408361,1.28127618901461,123.01287122073));
#51810=CARTESIAN_POINT('Ctrl Pts',(17.1851908013954,0.844766685164182,123.05147176177));
#51811=CARTESIAN_POINT('Ctrl Pts',(16.9804906029009,0.235476790658082,123.090121547379));
#51812=CARTESIAN_POINT('Ctrl Pts',(17.0063897534652,-0.266692007359343,
123.121068363773));
#51813=CARTESIAN_POINT('Ctrl Pts',(17.1538193871115,-0.747580694334549,
123.152031740723));
#51814=CARTESIAN_POINT('Ctrl Pts',(17.5553447104498,-1.25148896205411,123.190765979047));
#51815=CARTESIAN_POINT('Ctrl Pts',(18.2089111413414,-1.52674514579364,123.233411566373));
#51816=CARTESIAN_POINT('Ctrl Pts',(18.845013323169,-1.50249908902663,123.272206310198));
#51817=CARTESIAN_POINT('Ctrl Pts',(19.3702773407149,-1.27357787369309,123.307138988368));
#51818=CARTESIAN_POINT('Ctrl Pts',(19.7757310421874,-0.868041960323205,
123.342086539292));
#51819=CARTESIAN_POINT('Ctrl Pts',(20.0050916775235,-0.342429526733087,
123.377046507916));
#51820=CARTESIAN_POINT('Ctrl Pts',(20.0265714206272,0.230936564025209,123.412016066948));
#51821=CARTESIAN_POINT('Ctrl Pts',(19.8370330508419,0.772511505541999,123.446993063256));
#51822=CARTESIAN_POINT('Ctrl Pts',(19.5251158650213,1.13509549584705,123.476144022344));
#51823=CARTESIAN_POINT('Ctrl Pts',(19.2089427812759,1.34157439541724,123.499466157668));
#51824=CARTESIAN_POINT('Ctrl Pts',(18.8022297310169,1.51083005679838,123.526675351318));
#51825=CARTESIAN_POINT('Ctrl Pts',(18.1887610066183,1.54150746802044,123.563601539563));
#51826=CARTESIAN_POINT('Ctrl Pts',(17.6066469876977,1.26096106460104,123.602465316226));
#51827=CARTESIAN_POINT('Ctrl Pts',(17.2634272748862,0.890203007238264,123.633549572047));
#51828=CARTESIAN_POINT('Ctrl Pts',(17.082525889251,0.557815732951941,123.656858912516));
#51829=CARTESIAN_POINT('Ctrl Pts',(16.9571642283976,0.0684428947444481,
123.687931234929));
#51830=CARTESIAN_POINT('Ctrl Pts',(17.0295068117547,-0.507832033319457,
123.722875203782));
#51831=CARTESIAN_POINT('Ctrl Pts',(17.3688526160543,-1.04683816221682,123.76168087717));
#51832=CARTESIAN_POINT('Ctrl Pts',(17.8485226943806,-1.40115675162508,123.798041904308));
#51833=CARTESIAN_POINT('Ctrl Pts',(18.4538939392114,-1.54830506570096,123.835832958897));
#51834=CARTESIAN_POINT('Ctrl Pts',(19.0894977356217,-1.43102650733447,123.875047216809));
#51835=CARTESIAN_POINT('Ctrl Pts',(19.5769795248757,-1.09521158649819,123.910962428104));
#51836=CARTESIAN_POINT('Ctrl Pts',(19.8171106927969,-0.743274952053088,
123.937060754552));
#51837=CARTESIAN_POINT('Ctrl Pts',(19.9502929533394,-0.41864633746552,123.958798228661));
#51838=CARTESIAN_POINT('Ctrl Pts',(20.0158658834292,-0.0890469932101259,
123.979438649622));
#51839=CARTESIAN_POINT('Ctrl Pts',(19.9801779106362,0.333611522888986,124.00549195359));
#51840=CARTESIAN_POINT('Ctrl Pts',(19.8290153175581,0.729564899250391,124.031524512427));
#51841=CARTESIAN_POINT('Ctrl Pts',(19.5743395932742,1.06792890083028,124.057536023747));
#51842=CARTESIAN_POINT('Ctrl Pts',(19.2362602337412,1.32231677379998,124.083524975047));
#51843=CARTESIAN_POINT('Ctrl Pts',(18.8741909391828,1.46053309200947,124.107326736802));
#51844=CARTESIAN_POINT('Ctrl Pts',(18.5262231917483,1.50202994660038,124.128946988843));
#51845=CARTESIAN_POINT('Ctrl Pts',(18.1076238579464,1.4640685601785,124.154872476773));
#51846=CARTESIAN_POINT('Ctrl Pts',(17.6176451983895,1.2530494858779,124.187242696241));
#51847=CARTESIAN_POINT('Ctrl Pts',(17.1851241144578,0.782275600676782,124.226025525988));
#51848=CARTESIAN_POINT('Ctrl Pts',(16.9829299045482,0.1770230330116,124.264743351255));
#51849=CARTESIAN_POINT('Ctrl Pts',(17.0454911865098,-0.456965239846467,
124.30339306494));
#51850=CARTESIAN_POINT('Ctrl Pts',(17.3609592723271,-1.00905161410177,124.341971388204));
#51851=CARTESIAN_POINT('Ctrl Pts',(17.8734251128938,-1.38342287409913,124.380475205641));
#51852=CARTESIAN_POINT('Ctrl Pts',(18.4928529976412,-1.51554782034155,124.418901391255));
#51853=CARTESIAN_POINT('Ctrl Pts',(19.1109216504511,-1.38342471232708,124.457246905499));
#51854=CARTESIAN_POINT('Ctrl Pts',(19.6200023544194,-1.01118544846169,124.49550874605));
#51855=CARTESIAN_POINT('Ctrl Pts',(19.9319316125004,-0.464719077268282,
124.533683975605));
#51856=CARTESIAN_POINT('Ctrl Pts',(19.9933046864079,0.160025206387855,124.571769710634));
#51857=CARTESIAN_POINT('Ctrl Pts',(19.7946296329937,0.753903791122387,124.609763131141));
#51858=CARTESIAN_POINT('Ctrl Pts',(19.3717730079164,1.21368184599254,124.64766147922));
#51859=CARTESIAN_POINT('Ctrl Pts',(18.7994810228966,1.46000434721644,124.685462062322));
#51860=CARTESIAN_POINT('Ctrl Pts',(18.1781480997808,1.45111278538542,124.723162252709));
#51861=CARTESIAN_POINT('Ctrl Pts',(17.6161784166517,1.1899275989982,124.760759491016));
#51862=CARTESIAN_POINT('Ctrl Pts',(17.2110444840083,0.723298061997832,124.798251287713));
#51863=CARTESIAN_POINT('Ctrl Pts',(17.0323572001242,0.13359183205746,124.835635225636));
#51864=CARTESIAN_POINT('Ctrl Pts',(17.1098918761081,-0.475863436901096,
124.872908960883));
#51865=CARTESIAN_POINT('Ctrl Pts',(17.4286318467171,-0.998910009243678,
124.910070223437));
#51866=CARTESIAN_POINT('Ctrl Pts',(17.9316532413484,-1.34507560956785,124.94711681947));
#51867=CARTESIAN_POINT('Ctrl Pts',(18.5302997942462,-1.4552410218869,124.984046633175));
#51868=CARTESIAN_POINT('Ctrl Pts',(19.1198269249153,-1.31174356609111,125.020857628516));
#51869=CARTESIAN_POINT('Ctrl Pts',(19.5977510346322,-0.941189098052047,
125.057547850278));
#51870=CARTESIAN_POINT('Ctrl Pts',(19.8816855461754,-0.409529192802567,
125.094115424384));
#51871=CARTESIAN_POINT('Ctrl Pts',(19.9235560493417,0.18968666604768,125.130558559894));
#51872=CARTESIAN_POINT('Ctrl Pts',(19.7177399243904,0.751788965015347,125.166875550473));
#51873=CARTESIAN_POINT('Ctrl Pts',(19.3017530441372,1.17929037033942,125.203064775802));
#51874=CARTESIAN_POINT('Ctrl Pts',(18.7494159379068,1.39880874462414,125.239124702444));
#51875=CARTESIAN_POINT('Ctrl Pts',(18.1577440922458,1.37367073694802,125.275053884033));
#51876=CARTESIAN_POINT('Ctrl Pts',(17.6298927509336,1.11003035193486,125.310850962849));
#51877=CARTESIAN_POINT('Ctrl Pts',(17.2571574920252,0.655483923670628,125.346514670974));
#51878=CARTESIAN_POINT('Ctrl Pts',(17.1031737632591,0.090478868078499,125.382043831286));
#51879=CARTESIAN_POINT('Ctrl Pts',(17.1930513384486,-0.485932720696993,
125.417437358099));
#51880=CARTESIAN_POINT('Ctrl Pts',(17.5092987036455,-0.97347085777756,125.452694257279));
#51881=CARTESIAN_POINT('Ctrl Pts',(17.9951946615233,-1.28808402644339,125.487813627298));
#51882=CARTESIAN_POINT('Ctrl Pts',(18.5649614447451,-1.37644458054661,125.522794660169));
#51883=CARTESIAN_POINT('Ctrl Pts',(19.1189140641177,-1.22498304396499,125.557636641932));
#51884=CARTESIAN_POINT('Ctrl Pts',(19.5609089134785,-0.861932403090798,
125.592338953059));
#51885=CARTESIAN_POINT('Ctrl Pts',(19.8150359936985,-0.3520829415954,125.626901068439));
#51886=CARTESIAN_POINT('Ctrl Pts',(19.8386557221893,0.214780046773663,125.661322558033));
#51887=CARTESIAN_POINT('Ctrl Pts',(19.6295419625641,0.739691486449853,125.695603087442));
#51888=CARTESIAN_POINT('Ctrl Pts',(19.2259376869629,1.13178788840374,125.729742418013));
#51889=CARTESIAN_POINT('Ctrl Pts',(18.699572821645,1.32403667491472,125.763740406868));
#51890=CARTESIAN_POINT('Ctrl Pts',(18.1429176388844,1.28469073562223,125.79759700673));
#51891=CARTESIAN_POINT('Ctrl Pts',(17.6529372209239,1.02251218425985,125.83131226639));
#51892=CARTESIAN_POINT('Ctrl Pts',(17.314201690391,0.584910210351183,125.864886330625));
#51893=CARTESIAN_POINT('Ctrl Pts',(17.1842938014887,0.0493775379142845,
125.8983194402));
#51894=CARTESIAN_POINT('Ctrl Pts',(17.2840304301682,-0.490228611078988,
125.931611931248));
#51895=CARTESIAN_POINT('Ctrl Pts',(17.5941561350494,-0.940132612138631,
125.964764235148));
#51896=CARTESIAN_POINT('Ctrl Pts',(18.0590277207118,-1.2229319970556,125.997776878586));
#51897=CARTESIAN_POINT('Ctrl Pts',(18.5965888870425,-1.29090509505102,126.030650483148));
#51898=CARTESIAN_POINT('Ctrl Pts',(19.1128476053057,-1.13404910216438,126.063385764873));
#51899=CARTESIAN_POINT('Ctrl Pts',(19.5183028611001,-0.781498242508856,
126.095983533252));
#51900=CARTESIAN_POINT('Ctrl Pts',(19.7434513004666,-0.296132794314435,
126.128444690937));
#51901=CARTESIAN_POINT('Ctrl Pts',(19.7506887966976,0.236626129343923,126.160770233622));
#51902=CARTESIAN_POINT('Ctrl Pts',(19.5405717683373,0.723840014487345,126.192961249111));
#51903=CARTESIAN_POINT('Ctrl Pts',(19.1514003155747,1.08125376520771,126.225018916639));
#51904=CARTESIAN_POINT('Ctrl Pts',(18.6522529654985,1.24785219893955,126.256944505325));
#51905=CARTESIAN_POINT('Ctrl Pts',(18.1307374876082,1.19626020002051,126.288739373834));
#51906=CARTESIAN_POINT('Ctrl Pts',(17.6776283044279,0.937216920035472,126.320404969913));
#51907=CARTESIAN_POINT('Ctrl Pts',(17.3710826183557,0.517398188580757,126.351942829254));
#51908=CARTESIAN_POINT('Ctrl Pts',(17.2631766509069,0.0110212755183283,
126.383354574252));
#51909=CARTESIAN_POINT('Ctrl Pts',(17.3710775008581,-0.493259952344315,
126.414641912253));
#51910=CARTESIAN_POINT('Ctrl Pts',(17.674343269895,-0.907858065298181,126.445806634917));
#51911=CARTESIAN_POINT('Ctrl Pts',(18.1187695860277,-1.16144504596442,126.476850617591));
#51912=CARTESIAN_POINT('Ctrl Pts',(18.6260618945864,-1.21120322734561,126.507775817858));
#51913=CARTESIAN_POINT('Ctrl Pts',(19.1076094508818,-1.05003444205409,126.538584273908));
#51914=CARTESIAN_POINT('Ctrl Pts',(19.479941054855,-0.707518256395985,126.569278102458));
#51915=CARTESIAN_POINT('Ctrl Pts',(19.6791707230463,-0.24450208536029,126.599859497819));
#51916=CARTESIAN_POINT('Ctrl Pts',(19.6719374762803,0.257689964881801,126.630330731029));
#51917=CARTESIAN_POINT('Ctrl Pts',(19.4609699048984,0.711518134755177,126.660694148595));
#51918=CARTESIAN_POINT('Ctrl Pts',(19.0843530164292,1.03846031023916,126.690952169495));
#51919=CARTESIAN_POINT('Ctrl Pts',(18.6086699841862,1.18257251108356,126.721107284798));
#51920=CARTESIAN_POINT('Ctrl Pts',(18.1172532654699,1.12003822633395,126.751162052644));
#51921=CARTESIAN_POINT('Ctrl Pts',(17.6956108030026,0.863083641583314,126.781119104258));
#51922=CARTESIAN_POINT('Ctrl Pts',(17.416579633507,0.457614474125132,126.810981129717));
#51923=CARTESIAN_POINT('Ctrl Pts',(17.3277652379225,-0.0249623152391279,
126.840750898208));
#51924=CARTESIAN_POINT('Ctrl Pts',(17.4434533079629,-0.500296570460753,
126.870431213523));
#51925=CARTESIAN_POINT('Ctrl Pts',(17.7423144868672,-0.88579332001242,126.90002499059));
#51926=CARTESIAN_POINT('Ctrl Pts',(18.1713583899084,-1.11496153501696,126.929535108301));
#51927=CARTESIAN_POINT('Ctrl Pts',(18.6552355318737,-1.14880190241397,126.958964681934));
#51928=CARTESIAN_POINT('Ctrl Pts',(19.1095782364948,-0.982521504293672,
126.988316543786));
#51929=CARTESIAN_POINT('Ctrl Pts',(19.3977730939009,-0.702071800600608,
127.012714617116));
#51930=CARTESIAN_POINT('Ctrl Pts',(19.544407755015,-0.422356879638505,127.032197081111));
#51931=CARTESIAN_POINT('Ctrl Pts',(19.6298827620869,-0.118693626635683,
127.051656751625));
#51932=CARTESIAN_POINT('Ctrl Pts',(19.6130086123708,0.281159288420498,127.075938299492));
#51933=CARTESIAN_POINT('Ctrl Pts',(19.398925270687,0.709905348928385,127.105011643396));
#51934=CARTESIAN_POINT('Ctrl Pts',(19.0292329604127,1.01317916174629,127.13402325986));
#51935=CARTESIAN_POINT('Ctrl Pts',(18.5688144179712,1.13875566987803,127.162976744829));
#51936=CARTESIAN_POINT('Ctrl Pts',(18.0981675564226,1.06546968077371,127.191875335313));
#51937=CARTESIAN_POINT('Ctrl Pts',(17.6992029213682,0.806808307174844,127.220722517499));
#51938=CARTESIAN_POINT('Ctrl Pts',(17.4411124901692,0.408418905232783,127.2495217004));
#51939=CARTESIAN_POINT('Ctrl Pts',(17.3683562548528,-0.059914175730859,
127.278276385889));
#51940=CARTESIAN_POINT('Ctrl Pts',(17.4930509072919,-0.516467398722105,
127.306990073295));
#51941=CARTESIAN_POINT('Ctrl Pts',(17.7929496172605,-0.881797347761693,
127.335666305827));
#51942=CARTESIAN_POINT('Ctrl Pts',(18.2154066647599,-1.09252862496411,127.364308643604));
#51943=CARTESIAN_POINT('Ctrl Pts',(18.6865908567962,-1.11231576412509,127.392920676274));
#51944=CARTESIAN_POINT('Ctrl Pts',(19.1243553998719,-0.938093194560736,
127.421506009437));
#51945=CARTESIAN_POINT('Ctrl Pts',(19.45251882398,-0.600540327235931,127.45006827227));
#51946=CARTESIAN_POINT('Ctrl Pts',(19.6140849830491,-0.158694271514664,
127.478611095749));
#51947=CARTESIAN_POINT('Ctrl Pts',(19.5811155297149,0.310347270840708,127.507138158241));
#51948=CARTESIAN_POINT('Ctrl Pts',(19.3595430994241,0.724840908398939,127.535653065854));
#51949=CARTESIAN_POINT('Ctrl Pts',(18.9881132079945,1.01260452927925,127.564159617603));
#51950=CARTESIAN_POINT('Ctrl Pts',(18.531618625509,1.1235480699415,127.592661253259));
#51951=CARTESIAN_POINT('Ctrl Pts',(18.0696423587533,1.03837509085643,127.621162112442));
#51952=CARTESIAN_POINT('Ctrl Pts',(17.6827054043867,0.771915824816395,127.649664924942));
#51953=CARTESIAN_POINT('Ctrl Pts',(17.4382943211488,0.370573227075538,127.678175448639));
#51954=CARTESIAN_POINT('Ctrl Pts',(17.3790816129046,-0.0957583806675449,
127.706693056054));
#51955=CARTESIAN_POINT('Ctrl Pts',(17.5156217028773,-0.54581326651222,127.735229383328));
#51956=CARTESIAN_POINT('Ctrl Pts',(17.8241150899294,-0.901101660216496,
127.763774970624));
#51957=CARTESIAN_POINT('Ctrl Pts',(18.2514042557898,-1.09944789271686,127.792354060315));
#51958=CARTESIAN_POINT('Ctrl Pts',(18.7223811907647,-1.10621903008227,127.820935645081));
#51959=CARTESIAN_POINT('Ctrl Pts',(19.1561166875056,-0.919327144483553,
127.849587422587));
#51960=CARTESIAN_POINT('Ctrl Pts',(19.4756002029098,-0.572270806023172,
127.878200076059));
#51961=CARTESIAN_POINT('Ctrl Pts',(19.6249067912141,-0.122932666865693,
127.906929915726));
#51962=CARTESIAN_POINT('Ctrl Pts',(19.5878100755787,0.269735776585891,127.930897472309));
#51963=CARTESIAN_POINT('Ctrl Pts',(19.4623935348208,0.552856736689258,127.94996601605));
#51964=CARTESIAN_POINT('Ctrl Pts',(19.3242851294489,0.74328918256335,127.964401021732));
#51965=CARTESIAN_POINT('Ctrl Pts',(19.1499004928383,0.900980613118008,127.978886757729));
#51966=CARTESIAN_POINT('Ctrl Pts',(18.951180564553,1.01733117928007,127.99328776375));
#51967=CARTESIAN_POINT('Ctrl Pts',(18.7347414903714,1.08846509195581,128.007592012474));
#51968=CARTESIAN_POINT('Ctrl Pts',(18.5768458460658,1.10568133857386,128.01727789117));
#51969=CARTESIAN_POINT('Ctrl Pts',(18.4937646355866,1.10638059843974,128.022196038513));
#51970=CARTESIAN_POINT('Ctrl Pts',(18.4930824954759,1.12090089948759,112.757679850141));
#51971=CARTESIAN_POINT('Ctrl Pts',(18.3665883682682,1.11983625122485,112.765167906081));
#51972=CARTESIAN_POINT('Ctrl Pts',(18.2101165898736,1.09441509929884,112.774937242857));
#51973=CARTESIAN_POINT('Ctrl Pts',(17.9940242321427,1.01053960936053,112.789530556343));
#51974=CARTESIAN_POINT('Ctrl Pts',(17.8253522939624,0.911714328966616,112.801759037985));
#51975=CARTESIAN_POINT('Ctrl Pts',(17.6473020816238,0.750791187869453,112.816545585475));
#51976=CARTESIAN_POINT('Ctrl Pts',(17.5057913426302,0.555764932259308,112.831330741684));
#51977=CARTESIAN_POINT('Ctrl Pts',(17.3767761116466,0.264559939346119,112.850945111638));
#51978=CARTESIAN_POINT('Ctrl Pts',(17.3383331924762,-0.140265095337886,
112.875655684827));
#51979=CARTESIAN_POINT('Ctrl Pts',(17.4927882555132,-0.605925596627459,
112.905423832316));
#51980=CARTESIAN_POINT('Ctrl Pts',(17.8254561829886,-0.967734043234468,
112.935237085143));
#51981=CARTESIAN_POINT('Ctrl Pts',(18.2793089423996,-1.16352235132462,112.965222037507));
#51982=CARTESIAN_POINT('Ctrl Pts',(18.7747576544017,-1.15669178044294,112.995289912586));
#51983=CARTESIAN_POINT('Ctrl Pts',(19.2264713360212,-0.947257459845427,
113.02549484845));
#51984=CARTESIAN_POINT('Ctrl Pts',(19.5543003375184,-0.570103883609804,
113.055812262305));
#51985=CARTESIAN_POINT('Ctrl Pts',(19.7002188514683,-0.0899595846873296,
113.086259988855));
#51986=CARTESIAN_POINT('Ctrl Pts',(19.6369907959431,0.409971727794146,113.1168309809));
#51987=CARTESIAN_POINT('Ctrl Pts',(19.3739931350828,0.842295715905271,113.147533111348));
#51988=CARTESIAN_POINT('Ctrl Pts',(18.955569154602,1.13072856629342,113.178365554388));
#51989=CARTESIAN_POINT('Ctrl Pts',(18.4536699456387,1.22350120172658,113.209331880026));
#51990=CARTESIAN_POINT('Ctrl Pts',(17.955480573998,1.10266249250285,113.240433415561));
#51991=CARTESIAN_POINT('Ctrl Pts',(17.5483074543974,0.787495789961384,113.271672405762));
#51992=CARTESIAN_POINT('Ctrl Pts',(17.3042899501749,0.331487994701509,113.303050509289));
#51993=CARTESIAN_POINT('Ctrl Pts',(17.2676425549497,-0.186732323798034,
113.334569540469));
#51994=CARTESIAN_POINT('Ctrl Pts',(17.4466617531715,-0.676931075321784,
113.366231100277));
#51995=CARTESIAN_POINT('Ctrl Pts',(17.8119359198239,-1.05296122692266,113.39803672783));
#51996=CARTESIAN_POINT('Ctrl Pts',(18.3011750647179,-1.24788995601349,113.429987890354));
#51997=CARTESIAN_POINT('Ctrl Pts',(18.8297649694566,-1.22589192727795,113.462085865074));
#51998=CARTESIAN_POINT('Ctrl Pts',(19.3054703951861,-0.988819290874638,
113.494331996892));
#51999=CARTESIAN_POINT('Ctrl Pts',(19.6444065316308,-0.576226626359959,
113.526727323068));
#52000=CARTESIAN_POINT('Ctrl Pts',(19.7859212202161,-0.0588050517471134,
113.559272952392));
#52001=CARTESIAN_POINT('Ctrl Pts',(19.7033719576413,0.47377367502414,113.591969792592));
#52002=CARTESIAN_POINT('Ctrl Pts',(19.4091319363877,0.928265721457266,113.624818684065));
#52003=CARTESIAN_POINT('Ctrl Pts',(18.9528039781542,1.22434665049485,113.657820367104));
#52004=CARTESIAN_POINT('Ctrl Pts',(18.5028388600387,1.29449412400773,113.68544960784));
#52005=CARTESIAN_POINT('Ctrl Pts',(18.1479930389594,1.23643849564634,113.707629976648));
#52006=CARTESIAN_POINT('Ctrl Pts',(17.8120670406829,1.10593529978113,113.729861743692));
#52007=CARTESIAN_POINT('Ctrl Pts',(17.4566011291118,0.814568801733298,113.75774788851));
#52008=CARTESIAN_POINT('Ctrl Pts',(17.2089757557268,0.318843304737269,113.791365973));
#52009=CARTESIAN_POINT('Ctrl Pts',(17.1852851292711,-0.237300982291561,
113.82513892758));
#52010=CARTESIAN_POINT('Ctrl Pts',(17.3917751493225,-0.757010035973108,
113.859066883272));
#52011=CARTESIAN_POINT('Ctrl Pts',(17.7943511543741,-1.14882229284447,113.893149827088));
#52012=CARTESIAN_POINT('Ctrl Pts',(18.3242514269155,-1.34291473661002,113.927387660746));
#52013=CARTESIAN_POINT('Ctrl Pts',(18.8897524203654,-1.30346129922779,113.96178017383));
#52014=CARTESIAN_POINT('Ctrl Pts',(19.3920622637203,-1.0352770156871,113.996327045818));
#52015=CARTESIAN_POINT('Ctrl Pts',(19.7425772839418,-0.583305907411899,
114.031027870034));
#52016=CARTESIAN_POINT('Ctrl Pts',(19.8785122908702,-0.0251396062433737,
114.065882103309));
#52017=CARTESIAN_POINT('Ctrl Pts',(19.7741540483073,0.542360198983367,114.100889139007));
#52018=CARTESIAN_POINT('Ctrl Pts',(19.4456896959022,1.01978490940607,114.136048227714));
#52019=CARTESIAN_POINT('Ctrl Pts',(18.9487316956458,1.32271689126222,114.171358545353));
#52020=CARTESIAN_POINT('Ctrl Pts',(18.3689335050377,1.3965536931616,114.206819149106));
#52021=CARTESIAN_POINT('Ctrl Pts',(17.8071893150124,1.22642114794512,114.242429002406));
#52022=CARTESIAN_POINT('Ctrl Pts',(17.3620871476616,0.840084178305824,114.278186961052));
#52023=CARTESIAN_POINT('Ctrl Pts',(17.1125862773131,0.303442518713258,114.314091790017));
#52024=CARTESIAN_POINT('Ctrl Pts',(17.1039992313928,-0.29069230440087,114.350142137921));
#52025=CARTESIAN_POINT('Ctrl Pts',(17.339781679565,-0.838712338207705,114.386336584108));
#52026=CARTESIAN_POINT('Ctrl Pts',(17.7805525009889,-1.24418911264205,114.422673554901));
#52027=CARTESIAN_POINT('Ctrl Pts',(18.3507274190001,-1.43506356953502,114.459151484535));
#52028=CARTESIAN_POINT('Ctrl Pts',(18.8512555693308,-1.38589286433566,114.489665673091));
#52029=CARTESIAN_POINT('Ctrl Pts',(19.2144873415626,-1.22603513103535,114.514145775214));
#52030=CARTESIAN_POINT('Ctrl Pts',(19.5373516406566,-0.994043405793173,
114.538671340607));
#52031=CARTESIAN_POINT('Ctrl Pts',(19.8365357359841,-0.585125520559961,
114.569412866718));
#52032=CARTESIAN_POINT('Ctrl Pts',(19.9641680455432,0.0116468285138929,
114.606436218208));
#52033=CARTESIAN_POINT('Ctrl Pts',(19.8365166045373,0.610578458805209,114.643590857788));
#52034=CARTESIAN_POINT('Ctrl Pts',(19.4740841771901,1.10687327644485,114.680874670396));
#52035=CARTESIAN_POINT('Ctrl Pts',(18.9387445540885,1.41286803486826,114.718285330484));
#52036=CARTESIAN_POINT('Ctrl Pts',(18.3230736607037,1.47372940305447,114.755820519772));
#52037=CARTESIAN_POINT('Ctrl Pts',(17.7343186963893,1.27715511909712,114.793477731825));
#52038=CARTESIAN_POINT('Ctrl Pts',(17.2757904414825,0.855945729927207,114.831254534063));
#52039=CARTESIAN_POINT('Ctrl Pts',(17.0284653198638,0.282361907137467,114.869148139596));
#52040=CARTESIAN_POINT('Ctrl Pts',(17.0362003735306,-0.274389704184093,
114.902933084858));
#52041=CARTESIAN_POINT('Ctrl Pts',(17.2085237252143,-0.725107334144531,
114.932566782391));
#52042=CARTESIAN_POINT('Ctrl Pts',(17.3951754462632,-0.973455623444401,
114.951654102959));
#52043=CARTESIAN_POINT('Ctrl Pts',(17.5456173829533,-1.11352655242482,114.964393287536));
#52044=CARTESIAN_POINT('Ctrl Pts',(17.6254879200035,-1.17821151495492,114.970766127917));
#52045=CARTESIAN_POINT('Ctrl Pts',(17.7098144577346,-1.23711376226772,114.977141778623));
#52046=CARTESIAN_POINT('Ctrl Pts',(17.8862821458639,-1.34296898272677,114.989899536136));
#52047=CARTESIAN_POINT('Ctrl Pts',(18.1776912562802,-1.45422368744665,115.00905699236));
#52048=CARTESIAN_POINT('Ctrl Pts',(18.5927994037828,-1.48930722877114,115.034647641612));
#52049=CARTESIAN_POINT('Ctrl Pts',(19.0022284342603,-1.40791898797909,115.060282536743));
#52050=CARTESIAN_POINT('Ctrl Pts',(19.3735618999477,-1.21609226917294,115.085962555239));
#52051=CARTESIAN_POINT('Ctrl Pts',(19.678145682308,-0.928385692937971,115.111685215156));
#52052=CARTESIAN_POINT('Ctrl Pts',(19.8908852298623,-0.567169870467851,
115.137450886196));
#52053=CARTESIAN_POINT('Ctrl Pts',(20.0319650959912,-0.0245695829546816,
115.171859957911));
#52054=CARTESIAN_POINT('Ctrl Pts',(19.9355006689882,0.545066308576247,115.206350112054));
#52055=CARTESIAN_POINT('Ctrl Pts',(19.6607594620582,0.954350677105631,115.236596811922));
#52056=CARTESIAN_POINT('Ctrl Pts',(19.4606676325734,1.14929313186806,115.253898981719));
#52057=CARTESIAN_POINT('Ctrl Pts',(19.2345360594306,1.31443977360675,115.271213897795));
#52058=CARTESIAN_POINT('Ctrl Pts',(19.0093660410988,1.4153511981227,115.286380615372));
#52059=CARTESIAN_POINT('Ctrl Pts',(18.8056648791855,1.46628172584519,115.299391205841));
#52060=CARTESIAN_POINT('Ctrl Pts',(18.70233708238,1.48460038389795,115.305898900516));
#52061=CARTESIAN_POINT('Ctrl Pts',(18.6152995235572,1.49382058101683,115.31132371314));
#52062=CARTESIAN_POINT('Ctrl Pts',(18.5453906128826,1.49743368689553,115.315664843346));
#52063=CARTESIAN_POINT('Ctrl Pts',(18.2616037566892,1.50286105643157,115.333272874718));
#52064=CARTESIAN_POINT('Ctrl Pts',(17.7457736243556,1.37132382404071,115.365273134799));
#52065=CARTESIAN_POINT('Ctrl Pts',(17.3050555028768,0.962837299905914,115.401418669274));
#52066=CARTESIAN_POINT('Ctrl Pts',(17.1086587613839,0.593395661306247,115.427273326137));
#52067=CARTESIAN_POINT('Ctrl Pts',(17.041754656606,0.395197980803883,115.440209277673));
#52068=CARTESIAN_POINT('Ctrl Pts',(17.0088461550716,0.231377891853717,115.45056305284));
#52069=CARTESIAN_POINT('Ctrl Pts',(16.9695299982344,-0.100563471670666,
115.471278156146));
#52070=CARTESIAN_POINT('Ctrl Pts',(17.0668112497359,-0.652391726720423,
115.504977987031));
#52071=CARTESIAN_POINT('Ctrl Pts',(17.5514104118804,-1.26053326074223,115.551724578996));
#52072=CARTESIAN_POINT('Ctrl Pts',(18.2091610061576,-1.53767209463446,115.594647763884));
#52073=CARTESIAN_POINT('Ctrl Pts',(18.8498791049214,-1.51327085728669,115.633721735647));
#52074=CARTESIAN_POINT('Ctrl Pts',(19.3792076114729,-1.28260786692149,115.668926420135));
#52075=CARTESIAN_POINT('Ctrl Pts',(19.7881337259166,-0.873687487640924,
115.704166304091));
#52076=CARTESIAN_POINT('Ctrl Pts',(19.9809069947669,-0.431787129828086,
115.733560457919));
#52077=CARTESIAN_POINT('Ctrl Pts',(20.0304646093459,-0.0539560084034985,
115.757090137144));
#52078=CARTESIAN_POINT('Ctrl Pts',(20.014513183359,0.231413092827471,115.774745421663));
#52079=CARTESIAN_POINT('Ctrl Pts',(19.9571325086356,0.462752236719258,115.789462821084));
#52080=CARTESIAN_POINT('Ctrl Pts',(19.8859980822438,0.638993028576267,115.801240368326));
#52081=CARTESIAN_POINT('Ctrl Pts',(19.7552607146953,0.892444019511638,115.818910181336));
#52082=CARTESIAN_POINT('Ctrl Pts',(19.4715368254779,1.22216613224498,115.84542538746));
#52083=CARTESIAN_POINT('Ctrl Pts',(18.9584318064315,1.49339724075382,115.880801368486));
#52084=CARTESIAN_POINT('Ctrl Pts',(18.3813899373706,1.55843356026758,115.916195855039));
#52085=CARTESIAN_POINT('Ctrl Pts',(17.9605504546436,1.44568553379809,115.942753651494));
#52086=CARTESIAN_POINT('Ctrl Pts',(17.7091835003908,1.30962683993775,115.96046307762));
#52087=CARTESIAN_POINT('Ctrl Pts',(17.5507370910921,1.20379635308115,115.972270697712));
#52088=CARTESIAN_POINT('Ctrl Pts',(17.3011550655096,0.98086341180248,115.992935385917));
#52089=CARTESIAN_POINT('Ctrl Pts',(17.1334706598133,0.714436140504968,116.012129312691));
#52090=CARTESIAN_POINT('Ctrl Pts',(17.0518809246904,0.490682531218659,116.026895286345));
#52091=CARTESIAN_POINT('Ctrl Pts',(17.0304611374528,0.422553018506051,116.031325075242));
#52092=CARTESIAN_POINT('Ctrl Pts',(17.0123149108823,0.353447043175113,116.035755043463));
#52093=CARTESIAN_POINT('Ctrl Pts',(16.9973973546347,0.283593260328368,116.04018507481));
#52094=CARTESIAN_POINT('Ctrl Pts',(16.9857382118008,0.213104433320238,116.044615258831));
#52095=CARTESIAN_POINT('Ctrl Pts',(16.9746811349069,0.118498464452188,116.050522304053));
#52096=CARTESIAN_POINT('Ctrl Pts',(16.9622358386438,-0.143393353812591,
116.066767577372));
#52097=CARTESIAN_POINT('Ctrl Pts',(17.0433378618505,-0.57191585117926,116.093351814281));
#52098=CARTESIAN_POINT('Ctrl Pts',(17.3527452079877,-1.06435322127642,116.128800325967));
#52099=CARTESIAN_POINT('Ctrl Pts',(17.8206484218217,-1.40967908128267,116.164247300363));
#52100=CARTESIAN_POINT('Ctrl Pts',(18.3823463748326,-1.56016792906666,116.199690802844));
#52101=CARTESIAN_POINT('Ctrl Pts',(18.960023412883,-1.49507323389592,116.235127425045));
#52102=CARTESIAN_POINT('Ctrl Pts',(19.473954356025,-1.22345837930286,116.270554878086));
#52103=CARTESIAN_POINT('Ctrl Pts',(19.7685848901886,-0.880932463929016,
116.298099485735));
#52104=CARTESIAN_POINT('Ctrl Pts',(19.9099467736206,-0.596314691693052,
116.317769354208));
#52105=CARTESIAN_POINT('Ctrl Pts',(19.9937199319316,-0.356497524231079,
116.333502033051));
#52106=CARTESIAN_POINT('Ctrl Pts',(20.0610683033509,0.0857899363499977,
116.361028744888));
#52107=CARTESIAN_POINT('Ctrl Pts',(19.915745394596,0.722908696208606,116.400330942654));
#52108=CARTESIAN_POINT('Ctrl Pts',(19.3969443143545,1.31053562959535,116.447453844904));
#52109=CARTESIAN_POINT('Ctrl Pts',(18.6612967313308,1.57818772307471,116.494529797347));
#52110=CARTESIAN_POINT('Ctrl Pts',(17.8879145752841,1.46154465113853,116.541552584403));
#52111=CARTESIAN_POINT('Ctrl Pts',(17.3562475109639,1.05855180793689,116.581666715373));
#52112=CARTESIAN_POINT('Ctrl Pts',(17.0822320017472,0.592142557113021,116.614895645628));
#52113=CARTESIAN_POINT('Ctrl Pts',(16.9381151379149,0.0381362663569181,
116.650049508666));
#52114=CARTESIAN_POINT('Ctrl Pts',(17.06135129899,-0.687251812711299,116.693934033461));
#52115=CARTESIAN_POINT('Ctrl Pts',(17.6489755475387,-1.34438516219944,116.746493535922));
#52116=CARTESIAN_POINT('Ctrl Pts',(18.4942268949859,-1.58756196052271,116.798942419545));
#52117=CARTESIAN_POINT('Ctrl Pts',(19.337338674134,-1.34440174201639,116.851272002281));
#52118=CARTESIAN_POINT('Ctrl Pts',(19.92063012609,-0.691351138595169,116.90347356047));
#52119=CARTESIAN_POINT('Ctrl Pts',(20.0418737752447,0.025869309660071,116.946861524311));
#52120=CARTESIAN_POINT('Ctrl Pts',(19.8998969931766,0.571745128810662,116.981499280576));
#52121=CARTESIAN_POINT('Ctrl Pts',(19.6858090505737,0.935720760934458,117.007440856283));
#52122=CARTESIAN_POINT('Ctrl Pts',(19.3789673554751,1.22500437846248,117.033343801827));
#52123=CARTESIAN_POINT('Ctrl Pts',(18.8805090860516,1.48367338497174,117.067829408806));
#52124=CARTESIAN_POINT('Ctrl Pts',(18.1606038475644,1.52404123757986,117.110835756358));
#52125=CARTESIAN_POINT('Ctrl Pts',(17.4056904905111,1.10626788119792,117.162275443176));
#52126=CARTESIAN_POINT('Ctrl Pts',(16.9902676509324,0.353713203820808,117.213539395222));
#52127=CARTESIAN_POINT('Ctrl Pts',(17.0387094918925,-0.501579978728816,
117.264620504126));
#52128=CARTESIAN_POINT('Ctrl Pts',(17.5329599372551,-1.19732719183391,117.31551163559));
#52129=CARTESIAN_POINT('Ctrl Pts',(18.3185603384476,-1.5222362057658,117.366206019748));
#52130=CARTESIAN_POINT('Ctrl Pts',(19.1532504124722,-1.37991603886097,117.416697051433));
#52131=CARTESIAN_POINT('Ctrl Pts',(19.7816490558389,-0.817671078757634,
117.466978403285));
#52132=CARTESIAN_POINT('Ctrl Pts',(20.0135833048256,-0.0107439011157763,
117.51704398714));
#52133=CARTESIAN_POINT('Ctrl Pts',(19.7816717126225,0.792319952976642,117.56688798825));
#52134=CARTESIAN_POINT('Ctrl Pts',(19.1608825384109,1.34636250207202,117.616504844247));
#52135=CARTESIAN_POINT('Ctrl Pts',(18.3443183643152,1.48453909285033,117.665889273317));
#52136=CARTESIAN_POINT('Ctrl Pts',(17.583080543547,1.16861015724102,117.715036278499));
#52137=CARTESIAN_POINT('Ctrl Pts',(17.1089685240541,0.499410868515231,117.763941144654));
#52138=CARTESIAN_POINT('Ctrl Pts',(17.063797208761,-0.315336896122432,117.812599443987));
#52139=CARTESIAN_POINT('Ctrl Pts',(17.4570085476632,-1.02554149240549,117.861007055314));
#52140=CARTESIAN_POINT('Ctrl Pts',(18.1640470768909,-1.41563553676877,117.909160155275));
#52141=CARTESIAN_POINT('Ctrl Pts',(18.9659789153658,-1.36996787540684,117.957055229807));
#52142=CARTESIAN_POINT('Ctrl Pts',(19.6170386441137,-0.907245642934142,
118.004689063668));
#52143=CARTESIAN_POINT('Ctrl Pts',(19.9205783683424,-0.173019719646544,
118.052058788429));
#52144=CARTESIAN_POINT('Ctrl Pts',(19.8095868167875,0.475732877498027,118.091311294739));
#52145=CARTESIAN_POINT('Ctrl Pts',(19.5257452599602,0.898279490209589,118.122578859281));
#52146=CARTESIAN_POINT('Ctrl Pts',(19.1385654967184,1.22658636111508,118.153756402072));
#52147=CARTESIAN_POINT('Ctrl Pts',(18.5132602545178,1.40641663127513,118.192559112172));
#52148=CARTESIAN_POINT('Ctrl Pts',(17.7674133597538,1.19077223754927,118.23884983952));
#52149=CARTESIAN_POINT('Ctrl Pts',(17.2537148357509,0.614990335990114,118.284866859679));
#52150=CARTESIAN_POINT('Ctrl Pts',(17.1258431048699,-0.141409915617434,
118.330609188837));
#52151=CARTESIAN_POINT('Ctrl Pts',(17.418242037862,-0.845576547539981,118.376076242404));
#52152=CARTESIAN_POINT('Ctrl Pts',(18.0366942746291,-1.28361257902887,118.421267732646));
#52153=CARTESIAN_POINT('Ctrl Pts',(18.7887803634788,-1.32517662651085,118.466183719367));
#52154=CARTESIAN_POINT('Ctrl Pts',(19.4436861157114,-0.962516049661502,
118.510824594297));
#52155=CARTESIAN_POINT('Ctrl Pts',(19.8029993786324,-0.310963483597782,
118.555191066519));
#52156=CARTESIAN_POINT('Ctrl Pts',(19.7609285432409,0.427174297464442,118.599284210161));
#52157=CARTESIAN_POINT('Ctrl Pts',(19.3350856476775,1.02632487648794,118.643105363827));
#52158=CARTESIAN_POINT('Ctrl Pts',(18.7727329827513,1.25846786869882,118.679397823757));
#52159=CARTESIAN_POINT('Ctrl Pts',(18.3022615240602,1.24425151779425,118.708297621323));
#52160=CARTESIAN_POINT('Ctrl Pts',(17.9671502464406,1.13772165563029,118.729905777668));
#52161=CARTESIAN_POINT('Ctrl Pts',(17.6755615111956,0.942607394299044,118.751447393656));
#52162=CARTESIAN_POINT('Ctrl Pts',(17.4500539954179,0.675538200698231,118.772922954479));
#52163=CARTESIAN_POINT('Ctrl Pts',(17.3077447937584,0.357268879764495,118.79433265138));
#52164=CARTESIAN_POINT('Ctrl Pts',(17.2592510930774,0.0132284868385163,
118.815676981559));
#52165=CARTESIAN_POINT('Ctrl Pts',(17.3077344272548,-0.329873474156492,
118.83695621263));
#52166=CARTESIAN_POINT('Ctrl Pts',(17.4253889548699,-0.592464205208098,
118.854635131944));
#52167=CARTESIAN_POINT('Ctrl Pts',(17.5599631022999,-0.77667438666265,118.868745986558));
#52168=CARTESIAN_POINT('Ctrl Pts',(17.7187598102564,-0.939688687757648,
118.882835792676));
#52169=CARTESIAN_POINT('Ctrl Pts',(18.0515602644821,-1.16295343598271,118.907436743883));
#52170=CARTESIAN_POINT('Ctrl Pts',(18.6297474877978,-1.26093160039624,118.942422930714));
#52171=CARTESIAN_POINT('Ctrl Pts',(19.2764330124332,-0.992404814600162,
118.984156975342));
#52172=CARTESIAN_POINT('Ctrl Pts',(19.61120284939,-0.519416332488902,119.018730962761));
#52173=CARTESIAN_POINT('Ctrl Pts',(19.686909231104,-0.134245860237119,119.042827779968));
#52174=CARTESIAN_POINT('Ctrl Pts',(19.6839452453031,0.0875961253331513,
119.056567264143));
#52175=CARTESIAN_POINT('Ctrl Pts',(19.6498909294618,0.306908054978469,119.070287444309));
#52176=CARTESIAN_POINT('Ctrl Pts',(19.5503299373673,0.566837211628185,119.087400456966));
#52177=CARTESIAN_POINT('Ctrl Pts',(19.283502207417,0.922706019580419,119.114703819853));
#52178=CARTESIAN_POINT('Ctrl Pts',(18.7847361296941,1.19802461749581,119.148688660687));
#52179=CARTESIAN_POINT('Ctrl Pts',(18.105589661502,1.15934359728563,119.189245337803));
#52180=CARTESIAN_POINT('Ctrl Pts',(17.554184317493,0.767457727973741,119.229582217277));
#52181=CARTESIAN_POINT('Ctrl Pts',(17.3401465479837,0.249355250526175,119.263018378624));
#52182=CARTESIAN_POINT('Ctrl Pts',(17.3533022473312,-0.184386285466681,
119.289663181768));
#52183=CARTESIAN_POINT('Ctrl Pts',(17.435058145981,-0.441987019344221,119.306274088754));
#52184=CARTESIAN_POINT('Ctrl Pts',(17.5283491445481,-0.604844175741195,
119.317879227065));
#52185=CARTESIAN_POINT('Ctrl Pts',(17.5907056725042,-0.691564410421368,
119.324504643888));
#52186=CARTESIAN_POINT('Ctrl Pts',(17.6590894370632,-0.773661699956384,
119.331125917677));
#52187=CARTESIAN_POINT('Ctrl Pts',(17.7548833948339,-0.866802523811535,
119.339395111115));
#52188=CARTESIAN_POINT('Ctrl Pts',(17.9272916167502,-0.992838247175765,
119.35260859244));
#52189=CARTESIAN_POINT('Ctrl Pts',(18.1722977532925,-1.10244509398686,119.369095798182));
#52190=CARTESIAN_POINT('Ctrl Pts',(18.4904870561884,-1.14730747422361,119.388832136372));
#52191=CARTESIAN_POINT('Ctrl Pts',(18.8078898486568,-1.1024397351981,119.408522019047));
#52192=CARTESIAN_POINT('Ctrl Pts',(19.0997912866972,-0.971773191355699,
119.428165514072));
#52193=CARTESIAN_POINT('Ctrl Pts',(19.3435464737509,-0.765863353259586,
119.447764277111));
#52194=CARTESIAN_POINT('Ctrl Pts',(19.520374037332,-0.50114213177421,119.467318315598));
#52195=CARTESIAN_POINT('Ctrl Pts',(19.6167962999359,-0.198456868038709,
119.486829786065));
#52196=CARTESIAN_POINT('Ctrl Pts',(19.625628021481,0.118361475213261,119.506297999103));
#52197=CARTESIAN_POINT('Ctrl Pts',(19.5597739900227,0.373606936035918,119.522487978212));
#52198=CARTESIAN_POINT('Ctrl Pts',(19.4663649515948,0.560527496785607,119.535418986606));
#52199=CARTESIAN_POINT('Ctrl Pts',(19.3185225194951,0.775596785762759,119.551566637584));
#52200=CARTESIAN_POINT('Ctrl Pts',(19.0310431260634,1.0114115820414,119.574127159248));
#52201=CARTESIAN_POINT('Ctrl Pts',(18.5711112904984,1.13679629805337,119.603048118056));
#52202=CARTESIAN_POINT('Ctrl Pts',(18.1014514961469,1.06361619886642,119.631887037596));
#52203=CARTESIAN_POINT('Ctrl Pts',(17.7037118047289,0.805695586947934,119.660647396262));
#52204=CARTESIAN_POINT('Ctrl Pts',(17.4466785036886,0.408850110880016,119.689332630667));
#52205=CARTESIAN_POINT('Ctrl Pts',(17.3743358538123,-0.0571818016204902,
119.717946446007));
#52206=CARTESIAN_POINT('Ctrl Pts',(17.4983253082146,-0.511079568737379,
119.746492162257));
#52207=CARTESIAN_POINT('Ctrl Pts',(17.7466129424125,-0.813384860531917,
119.770227025735));
#52208=CARTESIAN_POINT('Ctrl Pts',(18.0058293990763,-0.978443247176416,
119.789184216853));
#52209=CARTESIAN_POINT('Ctrl Pts',(18.2933141133492,-1.08617062167036,119.808122253429));
#52210=CARTESIAN_POINT('Ctrl Pts',(18.6825508024836,-1.10253496953756,119.831759004564));
#52211=CARTESIAN_POINT('Ctrl Pts',(19.1161093341978,-0.929908145532468,
119.860070187335));
#52212=CARTESIAN_POINT('Ctrl Pts',(19.4407832828235,-0.59588973771539,119.888332066323));
#52213=CARTESIAN_POINT('Ctrl Pts',(19.6004637023044,-0.159071451104862,
119.916548585756));
#52214=CARTESIAN_POINT('Ctrl Pts',(19.5678525962247,0.304175161164362,119.94472356439));
#52215=CARTESIAN_POINT('Ctrl Pts',(19.3491799377188,0.713159074225391,119.972860943747));
#52216=CARTESIAN_POINT('Ctrl Pts',(18.9829635246229,0.996826194546356,120.000964621022));
#52217=CARTESIAN_POINT('Ctrl Pts',(18.5333246059365,1.10605246133314,120.029038590895));
#52218=CARTESIAN_POINT('Ctrl Pts',(18.0786639414332,1.02221007217602,120.057086755249));
#52219=CARTESIAN_POINT('Ctrl Pts',(17.7616747610674,0.803810507414772,120.08044215356));
#52220=CARTESIAN_POINT('Ctrl Pts',(17.5781706881473,0.563020021594781,120.099117557111));
#52221=CARTESIAN_POINT('Ctrl Pts',(17.4485102894162,0.289546062171738,120.117787596985));
#52222=CARTESIAN_POINT('Ctrl Pts',(17.4000766883178,-0.0919110956988218,
120.141116750007));
#52223=CARTESIAN_POINT('Ctrl Pts',(17.5340026995979,-0.533317467951709,
120.169101926724));
#52224=CARTESIAN_POINT('Ctrl Pts',(17.8364514864612,-0.881453389642329,
120.197081436934));
#52225=CARTESIAN_POINT('Ctrl Pts',(18.2546972918622,-1.07569505981494,120.225059261169));
#52226=CARTESIAN_POINT('Ctrl Pts',(18.7158361983992,-1.08216853743163,120.253039487099));
#52227=CARTESIAN_POINT('Ctrl Pts',(19.1395027643609,-0.899695026965587,
120.281026122395));
#52228=CARTESIAN_POINT('Ctrl Pts',(19.4518086127432,-0.559968571162895,
120.309023214945));
#52229=CARTESIAN_POINT('Ctrl Pts',(19.5981997788132,-0.122089063377897,
120.33703477985));
#52230=CARTESIAN_POINT('Ctrl Pts',(19.552950474692,0.337696943191307,120.36506483566));
#52231=CARTESIAN_POINT('Ctrl Pts',(19.3236731730684,0.739225257076302,120.393117382629));
#52232=CARTESIAN_POINT('Ctrl Pts',(18.9500423513974,1.01234988098468,120.421196409681));
#52233=CARTESIAN_POINT('Ctrl Pts',(18.4969528285068,1.10915757122897,120.449305885466));
#52234=CARTESIAN_POINT('Ctrl Pts',(18.0432838645376,1.0123484532541,120.477449757804));
#52235=CARTESIAN_POINT('Ctrl Pts',(17.6682096728875,0.738317035565853,120.505631950467));
#52236=CARTESIAN_POINT('Ctrl Pts',(17.437423751279,0.334387982344825,120.533856363023));
#52237=CARTESIAN_POINT('Ctrl Pts',(17.3916675325301,-0.129330292288387,
120.562126866275));
#52238=CARTESIAN_POINT('Ctrl Pts',(17.5395597076022,-0.572076137360996,
120.590447299692));
#52239=CARTESIAN_POINT('Ctrl Pts',(17.855984803406,-0.916457888564851,120.618821467709));
#52240=CARTESIAN_POINT('Ctrl Pts',(18.2863409307668,-1.10194268406267,120.647253137918));
#52241=CARTESIAN_POINT('Ctrl Pts',(18.7559322318109,-1.09546592268358,120.67574604072));
#52242=CARTESIAN_POINT('Ctrl Pts',(19.1828951657191,-0.897307355511358,
120.704303864294));
#52243=CARTESIAN_POINT('Ctrl Pts',(19.4924290395271,-0.541191746237481,
120.732930254292));
#52244=CARTESIAN_POINT('Ctrl Pts',(19.629864127016,-0.0885718616664442,
120.761628805457));
#52245=CARTESIAN_POINT('Ctrl Pts',(19.5702915902,0.38194575566233,120.790403069716));
#52246=CARTESIAN_POINT('Ctrl Pts',(19.3230606442279,0.788211584401149,120.81925653667));
#52247=CARTESIAN_POINT('Ctrl Pts',(18.9303370039179,1.05884354017487,120.848192665372));
#52248=CARTESIAN_POINT('Ctrl Pts',(18.4599333444905,1.14572580145235,120.877214815781));
#52249=CARTESIAN_POINT('Ctrl Pts',(17.9936381567603,1.03256046278807,120.906326368603));
#52250=CARTESIAN_POINT('Ctrl Pts',(17.6130217950625,0.737867413805891,120.935530493837));
#52251=CARTESIAN_POINT('Ctrl Pts',(17.3852199880608,0.312046699813544,120.964830580706));
#52252=CARTESIAN_POINT('Ctrl Pts',(17.3510866111027,-0.171347529488756,
120.994229417955));
#52253=CARTESIAN_POINT('Ctrl Pts',(17.4762315523886,-0.513852621030988,
121.016355467724));
#52254=CARTESIAN_POINT('Ctrl Pts',(17.6138033107167,-0.708894863435242,
121.031138486187));
#52255=CARTESIAN_POINT('Ctrl Pts',(17.7186460182362,-0.828728920899541,
121.041003185243));
#52256=CARTESIAN_POINT('Ctrl Pts',(17.9338771397665,-1.00822503331039,121.058288970429));
#52257=CARTESIAN_POINT('Ctrl Pts',(18.3129598588467,-1.15930959599405,121.083050806596));
#52258=CARTESIAN_POINT('Ctrl Pts',(18.8041703554433,-1.13879633990496,121.112875718073));
#52259=CARTESIAN_POINT('Ctrl Pts',(19.2457859888915,-0.918670752954191,
121.142814329296));
#52260=CARTESIAN_POINT('Ctrl Pts',(19.5602240335785,-0.535856279758148,
121.172869253422));
#52261=CARTESIAN_POINT('Ctrl Pts',(19.6913854815473,-0.0561259788657527,
121.203043167138));
#52262=CARTESIAN_POINT('Ctrl Pts',(19.6148686833085,0.437325039991343,121.233338591474));
#52263=CARTESIAN_POINT('Ctrl Pts',(19.3423661747877,0.858198271022791,121.263758005378));
#52264=CARTESIAN_POINT('Ctrl Pts',(18.9199837839974,1.13220110886314,121.294303783052));
#52265=CARTESIAN_POINT('Ctrl Pts',(18.42042918257,1.21011500633407,121.32497822383));
#52266=CARTESIAN_POINT('Ctrl Pts',(17.9305393050093,1.07662958513204,121.355783533596));
#52267=CARTESIAN_POINT('Ctrl Pts',(17.5362003747735,0.753305442664608,121.386721831682));
#52268=CARTESIAN_POINT('Ctrl Pts',(17.3073177623713,0.295125520361277,121.417795146862));
#52269=CARTESIAN_POINT('Ctrl Pts',(17.2854401515084,-0.218834434459951,
121.449005416441));
#52270=CARTESIAN_POINT('Ctrl Pts',(17.4762374736664,-0.699031393505859,
121.480354486252));
#52271=CARTESIAN_POINT('Ctrl Pts',(17.8481867637241,-1.06103365410968,121.511844103753));
#52272=CARTESIAN_POINT('Ctrl Pts',(18.3377536992966,-1.24035134890439,121.543475928373));
#52273=CARTESIAN_POINT('Ctrl Pts',(18.8602278069233,-1.20390349087577,121.575251508684));
#52274=CARTESIAN_POINT('Ctrl Pts',(19.3243579160287,-0.956110272282689,
121.607172324249));
#52275=CARTESIAN_POINT('Ctrl Pts',(19.6482814584831,-0.538442349648599,
121.63923970298));
#52276=CARTESIAN_POINT('Ctrl Pts',(19.7739347309703,-0.0225425683993542,
121.671454972332));
#52277=CARTESIAN_POINT('Ctrl Pts',(19.6774652298788,0.502115753058099,121.703819199622));
#52278=CARTESIAN_POINT('Ctrl Pts',(19.3737224989186,0.943640496909592,121.736333532426));
#52279=CARTESIAN_POINT('Ctrl Pts',(18.9140030444815,1.22389593147418,121.768998887406));
#52280=CARTESIAN_POINT('Ctrl Pts',(18.377429165599,1.29225269519424,121.801816130025));
#52281=CARTESIAN_POINT('Ctrl Pts',(17.8573241502507,1.13475923997334,121.834786019857));
#52282=CARTESIAN_POINT('Ctrl Pts',(17.4450010757071,0.776910878603483,121.867909199878));
#52283=CARTESIAN_POINT('Ctrl Pts',(17.2137312599202,0.279562992177936,121.901186219253));
#52284=CARTESIAN_POINT('Ctrl Pts',(17.2057348606295,-0.2714116808315,121.934617523114));
#52285=CARTESIAN_POINT('Ctrl Pts',(17.4244858838036,-0.779938810205246,
121.968203442992));
#52286=CARTESIAN_POINT('Ctrl Pts',(17.8337421937975,-1.15649409223492,122.001944217451));
#52287=CARTESIAN_POINT('Ctrl Pts',(18.3635288783225,-1.33385851932845,122.035839968655));
#52288=CARTESIAN_POINT('Ctrl Pts',(18.9220955048508,-1.27911558981949,122.069890723435));
#52289=CARTESIAN_POINT('Ctrl Pts',(19.4118031026727,-0.999736384496644,
122.104096394088));
#52290=CARTESIAN_POINT('Ctrl Pts',(19.7461944871727,-0.542647687182364,
122.138456799284));
#52291=CARTESIAN_POINT('Ctrl Pts',(19.8652556008789,0.013647933341159,122.172971637033));
#52292=CARTESIAN_POINT('Ctrl Pts',(19.7461888829058,0.572532365852113,122.207640521162));
#52293=CARTESIAN_POINT('Ctrl Pts',(19.4077323355963,1.03609396929577,122.242462929572));
#52294=CARTESIAN_POINT('Ctrl Pts',(18.9072812151109,1.322227313061,122.277438289026));
#52295=CARTESIAN_POINT('Ctrl Pts',(18.3310963479423,1.37923683565688,122.312565853708));
#52296=CARTESIAN_POINT('Ctrl Pts',(17.7795212835281,1.19516070447226,122.34784483257));
#52297=CARTESIAN_POINT('Ctrl Pts',(17.3494069677128,0.800134075483034,122.38327430115));
#52298=CARTESIAN_POINT('Ctrl Pts',(17.1171842054199,0.261691707489099,122.418853238197));
#52299=CARTESIAN_POINT('Ctrl Pts',(17.1242829390838,-0.261793907771907,
122.450610839665));
#52300=CARTESIAN_POINT('Ctrl Pts',(17.2865889445715,-0.685649920943017,
122.478494089534));
#52301=CARTESIAN_POINT('Ctrl Pts',(17.5985838897628,-1.10207969945623,122.510447354666));
#52302=CARTESIAN_POINT('Ctrl Pts',(18.18666838241,-1.42792122315664,122.550550404142));
#52303=CARTESIAN_POINT('Ctrl Pts',(18.9968853221201,-1.38299738205048,122.598929027424));
#52304=CARTESIAN_POINT('Ctrl Pts',(19.6622552549554,-0.911544492503412,
122.647558773599));
#52305=CARTESIAN_POINT('Ctrl Pts',(19.9764902272409,-0.154570377655717,
122.696435587038));
#52306=CARTESIAN_POINT('Ctrl Pts',(19.8390738237385,0.657775266502406,122.74555504686));
#52307=CARTESIAN_POINT('Ctrl Pts',(19.3797620617075,1.17210955074175,122.786686268123));
#52308=CARTESIAN_POINT('Ctrl Pts',(18.8884735110166,1.39088302497454,122.819707738936));
#52309=CARTESIAN_POINT('Ctrl Pts',(18.5033111211165,1.44583087334473,122.843612041481));
#52310=CARTESIAN_POINT('Ctrl Pts',(18.1319627148124,1.39887538222455,122.866646747491));
#52311=CARTESIAN_POINT('Ctrl Pts',(17.6848506292388,1.22425836285374,122.896190503993));
#52312=CARTESIAN_POINT('Ctrl Pts',(17.2330030000641,0.805544093152841,122.933230312885));
#52313=CARTESIAN_POINT('Ctrl Pts',(17.0358813147302,0.219439642783941,122.970413341592));
#52314=CARTESIAN_POINT('Ctrl Pts',(17.0608067523446,-0.264630775831841,
123.000243864343));
#52315=CARTESIAN_POINT('Ctrl Pts',(17.2030640210597,-0.72877788689057,123.030129409407));
#52316=CARTESIAN_POINT('Ctrl Pts',(17.5912103662842,-1.21622770551833,123.067588736755));
#52317=CARTESIAN_POINT('Ctrl Pts',(18.2248499897429,-1.48333671290741,123.108939586315));
#52318=CARTESIAN_POINT('Ctrl Pts',(18.8430841455309,-1.45988936207864,123.146643846141));
#52319=CARTESIAN_POINT('Ctrl Pts',(19.35464113493,-1.23705318214091,123.180662420129));
#52320=CARTESIAN_POINT('Ctrl Pts',(19.7503526751607,-0.841413044968066,
123.214763669378));
#52321=CARTESIAN_POINT('Ctrl Pts',(19.9747043163627,-0.327540003001533,
123.248945585414));
#52322=CARTESIAN_POINT('Ctrl Pts',(19.9958554010032,0.234190739582267,123.283205786453));
#52323=CARTESIAN_POINT('Ctrl Pts',(19.809886470046,0.765886840091164,123.31754245384));
#52324=CARTESIAN_POINT('Ctrl Pts',(19.503128994245,1.12261086723232,123.346217672991));
#52325=CARTESIAN_POINT('Ctrl Pts',(19.1916465195094,1.32604725655206,123.369194036914));
#52326=CARTESIAN_POINT('Ctrl Pts',(18.7905766269883,1.49297621000668,123.396027008284));
#52327=CARTESIAN_POINT('Ctrl Pts',(18.1844752698309,1.52349251558905,123.432510323781));
#52328=CARTESIAN_POINT('Ctrl Pts',(17.6076908763952,1.24575162694292,123.471012023267));
#52329=CARTESIAN_POINT('Ctrl Pts',(17.2669358073587,0.877725128070975,123.501869301326));
#52330=CARTESIAN_POINT('Ctrl Pts',(17.0870893744063,0.547329694514233,123.525039768527));
#52331=CARTESIAN_POINT('Ctrl Pts',(16.9622603091664,0.0602367962628432,
123.555968827903));
#52332=CARTESIAN_POINT('Ctrl Pts',(17.0342291378425,-0.514571727658781,
123.590822340935));
#52333=CARTESIAN_POINT('Ctrl Pts',(17.3733949645324,-1.05353060709449,123.629619294211));
#52334=CARTESIAN_POINT('Ctrl Pts',(17.8538625057619,-1.40857439093685,123.666045889573));
#52335=CARTESIAN_POINT('Ctrl Pts',(18.461592831455,-1.5564523426571,123.703986589641));
#52336=CARTESIAN_POINT('Ctrl Pts',(19.101195146309,-1.43859456950387,123.743445712838));
#52337=CARTESIAN_POINT('Ctrl Pts',(19.5929149609134,-1.10003231948515,123.77966722315));
#52338=CARTESIAN_POINT('Ctrl Pts',(19.8356254005539,-0.74441967000705,123.806040285316));
#52339=CARTESIAN_POINT('Ctrl Pts',(19.9703654530638,-0.416005980207952,
123.828031369899));
#52340=CARTESIAN_POINT('Ctrl Pts',(20.0368072594968,-0.0822239677629709,
123.848934198666));
#52341=CARTESIAN_POINT('Ctrl Pts',(20.0006566043124,0.346454692026937,123.875358332762));
#52342=CARTESIAN_POINT('Ctrl Pts',(19.8471547497178,0.748660819823204,123.901800955164));
#52343=CARTESIAN_POINT('Ctrl Pts',(19.5881175815438,1.09289552386003,123.928261650183));
#52344=CARTESIAN_POINT('Ctrl Pts',(19.2437140701204,1.35209703835508,123.954738785435));
#52345=CARTESIAN_POINT('Ctrl Pts',(18.8743120378708,1.49315805935625,123.97902361159));
#52346=CARTESIAN_POINT('Ctrl Pts',(18.5188213115279,1.53557171478921,124.001111261365));
#52347=CARTESIAN_POINT('Ctrl Pts',(18.0907023088825,1.49677336723877,124.027626520082));
#52348=CARTESIAN_POINT('Ctrl Pts',(17.5886989835531,1.28071224384361,124.060787965071));
#52349=CARTESIAN_POINT('Ctrl Pts',(17.1445191175465,0.797474344906156,124.10060608365));
#52350=CARTESIAN_POINT('Ctrl Pts',(16.9363317375956,0.174754912879289,124.140444286067));
#52351=CARTESIAN_POINT('Ctrl Pts',(17.000693693818,-0.479009409878407,124.180298719382));
#52352=CARTESIAN_POINT('Ctrl Pts',(17.3265672215966,-1.04960547491672,124.220165279827));
#52353=CARTESIAN_POINT('Ctrl Pts',(17.8571916910488,-1.43742494106541,124.260039981735));
#52354=CARTESIAN_POINT('Ctrl Pts',(18.5000049546241,-1.57468781447863,124.299918766618));
#52355=CARTESIAN_POINT('Ctrl Pts',(19.142818830386,-1.43742342812486,124.339797610578));
#52356=CARTESIAN_POINT('Ctrl Pts',(19.6734460569893,-1.04960765164736,124.379672470623));
#52357=CARTESIAN_POINT('Ctrl Pts',(19.9993212502782,-0.478996882985747,
124.419539315287));
#52358=CARTESIAN_POINT('Ctrl Pts',(20.063685387175,0.17475275129412,124.459394112919));
#52359=CARTESIAN_POINT('Ctrl Pts',(19.855493029657,0.79751985498053,124.499232843074));
#52360=CARTESIAN_POINT('Ctrl Pts',(19.4113116700434,1.28068814713101,124.539051495894));
#52361=CARTESIAN_POINT('Ctrl Pts',(18.8088847361186,1.54012930695157,124.57884607634));
#52362=CARTESIAN_POINT('Ctrl Pts',(18.1534946893475,1.53088466548527,124.618612603657));
#52363=CARTESIAN_POINT('Ctrl Pts',(17.5595230439077,1.25497200645252,124.658347116273));
#52364=CARTESIAN_POINT('Ctrl Pts',(17.1304444180403,0.760962163490976,124.698045674236));
#52365=CARTESIAN_POINT('Ctrl Pts',(16.940761355013,0.135410421294839,124.73770436324));
#52366=CARTESIAN_POINT('Ctrl Pts',(17.0230407297764,-0.51234136906881,124.77731929645));
#52367=CARTESIAN_POINT('Ctrl Pts',(17.3623119928872,-1.0693180342063,124.81688661527));
#52368=CARTESIAN_POINT('Ctrl Pts',(17.8987924872961,-1.43865725028846,124.856402493113));
#52369=CARTESIAN_POINT('Ctrl Pts',(18.5384432864047,-1.55649001223549,124.89586313845));
#52370=CARTESIAN_POINT('Ctrl Pts',(19.1694876783657,-1.40300740644741,124.935264798184));
#52371=CARTESIAN_POINT('Ctrl Pts',(19.6819844911938,-1.00579246197517,124.974603759877));
#52372=CARTESIAN_POINT('Ctrl Pts',(19.9870215554236,-0.434856710408076,
125.013876352219));
#52373=CARTESIAN_POINT('Ctrl Pts',(20.0321717618401,0.209724078121503,125.053078948617));
#52374=CARTESIAN_POINT('Ctrl Pts',(19.8105195361387,0.815386929581868,125.092207970087));
#52375=CARTESIAN_POINT('Ctrl Pts',(19.361701163962,1.27677787532468,125.131259888399));
#52376=CARTESIAN_POINT('Ctrl Pts',(18.7648066215825,1.5141139501787,125.170231228365));
#52377=CARTESIAN_POINT('Ctrl Pts',(18.1244162904329,1.48700453469375,125.209118568196));
#52378=CARTESIAN_POINT('Ctrl Pts',(17.5522425067462,1.20133350244083,125.247918542709));
#52379=CARTESIAN_POINT('Ctrl Pts',(17.1476050430654,0.708028317127927,125.286627846152));
#52380=CARTESIAN_POINT('Ctrl Pts',(16.9801594170711,0.0939676037639261,
125.325243234936));
#52381=CARTESIAN_POINT('Ctrl Pts',(17.0778869149266,-0.533346746909132,
125.363761529995));
#52382=CARTESIAN_POINT('Ctrl Pts',(17.4224200985157,-1.0646435628828,125.402179617076));
#52383=CARTESIAN_POINT('Ctrl Pts',(17.9524839925264,-1.40794981777256,125.440494449376));
#52384=CARTESIAN_POINT('Ctrl Pts',(18.5748095291292,-1.50453836038642,125.47870305043));
#52385=CARTESIAN_POINT('Ctrl Pts',(19.1805722495993,-1.33898635608767,125.516802516252));
#52386=CARTESIAN_POINT('Ctrl Pts',(19.6644539096247,-0.941619949238724,
125.554790017782));
#52387=CARTESIAN_POINT('Ctrl Pts',(19.9429825043806,-0.382961689893696,
125.592662801021));
#52388=CARTESIAN_POINT('Ctrl Pts',(19.9689520201468,0.2388025468179,125.630418189203));
#52389=CARTESIAN_POINT('Ctrl Pts',(19.7394275641386,0.815106336169562,125.668053585541));
#52390=CARTESIAN_POINT('Ctrl Pts',(19.2959782023475,1.24598811837169,125.705566474907));
#52391=CARTESIAN_POINT('Ctrl Pts',(18.7171464460761,1.45745420294917,125.742954426178));
#52392=CARTESIAN_POINT('Ctrl Pts',(18.1045195341734,1.41419939899926,125.780215092177));
#52393=CARTESIAN_POINT('Ctrl Pts',(17.5648760765932,1.12549636275945,125.817346211604));
#52394=CARTESIAN_POINT('Ctrl Pts',(17.1915502824867,0.643272766242982,125.854345611245));
#52395=CARTESIAN_POINT('Ctrl Pts',(17.0482705064466,0.0527665519465494,
125.891211207534));
#52396=CARTESIAN_POINT('Ctrl Pts',(17.1582735037444,-0.54255765424983,125.927941008396));
#52397=CARTESIAN_POINT('Ctrl Pts',(17.5005545415035,-1.03915845752618,125.964533113257));
#52398=CARTESIAN_POINT('Ctrl Pts',(18.0138543548987,-1.35144610286629,126.000985714488));
#52399=CARTESIAN_POINT('Ctrl Pts',(18.6076292011844,-1.42654679770189,126.037297099343));
#52400=CARTESIAN_POINT('Ctrl Pts',(19.1780377234228,-1.25325431972676,126.073465651058));
#52401=CARTESIAN_POINT('Ctrl Pts',(19.6261188945682,-0.863654225443849,
126.109489850372));
#52402=CARTESIAN_POINT('Ctrl Pts',(19.8749757363862,-0.327195816840043,
126.145368275421));
#52403=CARTESIAN_POINT('Ctrl Pts',(19.8829785376702,0.261694286094789,126.181099602915));
#52404=CARTESIAN_POINT('Ctrl Pts',(19.650719858024,0.800245939977902,126.216682609493));
#52405=CARTESIAN_POINT('Ctrl Pts',(19.220561895408,1.19529383673981,126.252116172656));
#52406=CARTESIAN_POINT('Ctrl Pts',(18.6689174524219,1.37940357614657,126.287399271635));
#52407=CARTESIAN_POINT('Ctrl Pts',(18.0926704275284,1.32238292183252,126.322530987377));
#52408=CARTESIAN_POINT('Ctrl Pts',(17.5921506137728,1.03621366175272,126.357510503253));
#52409=CARTESIAN_POINT('Ctrl Pts',(17.2536567723353,0.572602926071189,126.392337106094));
#52410=CARTESIAN_POINT('Ctrl Pts',(17.1345737699536,0.0136453744042972,
126.427010186614));
#52411=CARTESIAN_POINT('Ctrl Pts',(17.2536504364034,-0.542717522157398,
126.461529239891));
#52412=CARTESIAN_POINT('Ctrl Pts',(17.5880834324056,-0.999864641603807,
126.495893865198));
#52413=CARTESIAN_POINT('Ctrl Pts',(18.0778530411477,-1.27927849056268,126.530103766427));
#52414=CARTESIAN_POINT('Ctrl Pts',(18.6364904459868,-1.33402870614301,126.564158752655));
#52415=CARTESIAN_POINT('Ctrl Pts',(19.1663446909442,-1.15664138180575,126.598058738222));
#52416=CARTESIAN_POINT('Ctrl Pts',(19.5756533377215,-0.78003806942924,126.631803742641));
#52417=CARTESIAN_POINT('Ctrl Pts',(19.794432443157,-0.271445460467721,126.665393890358));
#52418=CARTESIAN_POINT('Ctrl Pts',(19.7864349006516,0.27959998319499,126.69882941077));
#52419=CARTESIAN_POINT('Ctrl Pts',(19.5551353092926,0.777012272782376,126.732110638587));
#52420=CARTESIAN_POINT('Ctrl Pts',(19.1427587398274,1.13490641725472,126.765238013014));
#52421=CARTESIAN_POINT('Ctrl Pts',(18.6225867432735,1.29242086659805,126.798212078173));
#52422=CARTESIAN_POINT('Ctrl Pts',(18.0859430362728,1.22405396241437,126.831033480681));
#52423=CARTESIAN_POINT('Ctrl Pts',(17.6261649865072,0.943764553716469,126.863702973114));
#52424=CARTESIAN_POINT('Ctrl Pts',(17.3223818224607,0.502178353438225,126.896221407178));
#52425=CARTESIAN_POINT('Ctrl Pts',(17.2259017352908,-0.0225383357424905,
126.92858974499));
#52426=CARTESIAN_POINT('Ctrl Pts',(17.3515757437269,-0.538512892512059,
126.960809035826));
#52427=CARTESIAN_POINT('Ctrl Pts',(17.6755338947518,-0.956225990676644,
126.992880456677));
#52428=CARTESIAN_POINT('Ctrl Pts',(18.1397311835696,-1.20405787590894,127.024805234591));
#52429=CARTESIAN_POINT('Ctrl Pts',(18.6622539843598,-1.24049861448516,127.056584791087));
#52430=CARTESIAN_POINT('Ctrl Pts',(19.1519117947061,-1.06117933724715,127.088220467932));
#52431=CARTESIAN_POINT('Ctrl Pts',(19.4618550662539,-0.759439290617938,
127.114465119351));
#52432=CARTESIAN_POINT('Ctrl Pts',(19.6193300865727,-0.459005379949352,
127.135390361088));
#52433=CARTESIAN_POINT('Ctrl Pts',(19.7110223729966,-0.133185783680743,
127.156269267074));
#52434=CARTESIAN_POINT('Ctrl Pts',(19.6928503715007,0.295153408660477,127.182280859505));
#52435=CARTESIAN_POINT('Ctrl Pts',(19.4639046032388,0.753395195664358,127.213357950153));
#52436=CARTESIAN_POINT('Ctrl Pts',(19.0695377246349,1.07675375085461,127.244299876378));
#52437=CARTESIAN_POINT('Ctrl Pts',(18.5795803461416,1.21025686910366,127.275108807355));
#52438=CARTESIAN_POINT('Ctrl Pts',(18.0799738634865,1.13233247683963,127.305786783584));
#52439=CARTESIAN_POINT('Ctrl Pts',(17.6575395077607,0.858299579569359,127.336336050748));
#52440=CARTESIAN_POINT('Ctrl Pts',(17.3850098668066,0.437377398955207,127.366758880445));
#52441=CARTESIAN_POINT('Ctrl Pts',(17.3084803074032,-0.0561256639258518,
127.39705766334));
#52442=CARTESIAN_POINT('Ctrl Pts',(17.439663243693,-0.535912780145553,127.427234856148));
#52443=CARTESIAN_POINT('Ctrl Pts',(17.7541222443087,-0.918759596678555,
127.45729300688));
#52444=CARTESIAN_POINT('Ctrl Pts',(18.1958079698188,-1.13892417265509,127.487234739106));
#52445=CARTESIAN_POINT('Ctrl Pts',(18.6870232674475,-1.15940871276915,127.517062760317));
#52446=CARTESIAN_POINT('Ctrl Pts',(19.1420662103094,-0.978153105648501,
127.546779850572));
#52447=CARTESIAN_POINT('Ctrl Pts',(19.4821508736072,-0.628126893328401,
127.576388872373));
#52448=CARTESIAN_POINT('Ctrl Pts',(19.6490175278053,-0.171352587712298,
127.605892744728));
#52449=CARTESIAN_POINT('Ctrl Pts',(19.6148875667895,0.312060165323532,127.635294496316));
#52450=CARTESIAN_POINT('Ctrl Pts',(19.387060763882,0.737933090385993,127.664597137408));
#52451=CARTESIAN_POINT('Ctrl Pts',(19.0064135995696,1.03264512775516,127.69380393404));
#52452=CARTESIAN_POINT('Ctrl Pts',(18.5400762875866,1.14582302109237,127.722917848391));
#52453=CARTESIAN_POINT('Ctrl Pts',(18.069635799574,1.05893307361866,127.751942612257));
#52454=CARTESIAN_POINT('Ctrl Pts',(17.6768791166838,0.788277917073556,127.780880584301));
#52455=CARTESIAN_POINT('Ctrl Pts',(17.4296332142809,0.381982697626676,127.809737248291));
#52456=CARTESIAN_POINT('Ctrl Pts',(17.3700415360265,-0.0885703605568786,
127.838511718406));
#52457=CARTESIAN_POINT('Ctrl Pts',(17.507531797481,-0.541218118675741,127.867215509699));
#52458=CARTESIAN_POINT('Ctrl Pts',(17.816984019384,-0.897377443387583,127.895838832972));
#52459=CARTESIAN_POINT('Ctrl Pts',(18.244166417509,-1.09549488656034,127.924406623306));
#52460=CARTESIAN_POINT('Ctrl Pts',(18.7134661788609,-1.10209796420226,127.952885817208));
#52461=CARTESIAN_POINT('Ctrl Pts',(19.1442712717119,-0.916283636031154,
127.981348904678));
#52462=CARTESIAN_POINT('Ctrl Pts',(19.460485405136,-0.572567145982761,128.009677920323));
#52463=CARTESIAN_POINT('Ctrl Pts',(19.6077409437319,-0.12891228120585,128.038041366258));
#52464=CARTESIAN_POINT('Ctrl Pts',(19.571105117469,0.257508093441198,128.061628433663));
#52465=CARTESIAN_POINT('Ctrl Pts',(19.4479991183959,0.535304279391785,128.080339688794));
#52466=CARTESIAN_POINT('Ctrl Pts',(19.3125791070956,0.722042855063143,128.094494421635));
#52467=CARTESIAN_POINT('Ctrl Pts',(19.141797922151,0.876422884225493,128.108678534636));
#52468=CARTESIAN_POINT('Ctrl Pts',(18.9477421547559,0.990014057708069,128.122740918746));
#52469=CARTESIAN_POINT('Ctrl Pts',(18.7367548382266,1.05934633488113,128.136684558088));
#52470=CARTESIAN_POINT('Ctrl Pts',(18.582539945268,1.07619894693391,128.146145491089));
#52471=CARTESIAN_POINT('Ctrl Pts',(18.5011390454481,1.07688406432642,128.150964169306));
#52472=CARTESIAN_POINT('Ctrl Pts',(18.5048905446611,1.0769826448063,112.950906422413));
#52473=CARTESIAN_POINT('Ctrl Pts',(18.3830098066567,1.07595682551458,112.958121380168));
#52474=CARTESIAN_POINT('Ctrl Pts',(18.2332489107013,1.05152251268125,112.967474141999));
#52475=CARTESIAN_POINT('Ctrl Pts',(18.0268596028074,0.971442179610211,112.981411102263));
#52476=CARTESIAN_POINT('Ctrl Pts',(17.8656334975826,0.876962742492602,112.993100991851));
#52477=CARTESIAN_POINT('Ctrl Pts',(17.6954686455205,0.723186909327924,113.007230605468));
#52478=CARTESIAN_POINT('Ctrl Pts',(17.5608075681054,0.537408101995845,113.021310819524));
#52479=CARTESIAN_POINT('Ctrl Pts',(17.4385635814574,0.261558152501724,113.039890602226));
#52480=CARTESIAN_POINT('Ctrl Pts',(17.4023331932359,-0.121639614718659,
113.063280373129));
#52481=CARTESIAN_POINT('Ctrl Pts',(17.5481112006283,-0.560471337755449,
113.091337893366));
#52482=CARTESIAN_POINT('Ctrl Pts',(17.8601965720909,-0.899510546216632,
113.119288341739));
#52483=CARTESIAN_POINT('Ctrl Pts',(18.2843287346396,-1.08233432237433,113.147308243339));
#52484=CARTESIAN_POINT('Ctrl Pts',(18.7451740809681,-1.0757227904068,113.175274045851));
#52485=CARTESIAN_POINT('Ctrl Pts',(19.1636363346921,-0.881531337437797,
113.203262131254));
#52486=CARTESIAN_POINT('Ctrl Pts',(19.4659983852052,-0.53335175821849,113.231237553952));
#52487=CARTESIAN_POINT('Ctrl Pts',(19.5999624515289,-0.0919352051397887,
113.259227393613));
#52488=CARTESIAN_POINT('Ctrl Pts',(19.5418755258235,0.36583827782248,113.28722106912));
#52489=CARTESIAN_POINT('Ctrl Pts',(19.3017885872034,0.760159580845085,113.315231457202));
#52490=CARTESIAN_POINT('Ctrl Pts',(18.9213424421171,1.02219956875272,113.343257793308));
#52491=CARTESIAN_POINT('Ctrl Pts',(18.4667053085281,1.10606223937008,113.371306390066));
#52492=CARTESIAN_POINT('Ctrl Pts',(18.0170529864695,0.996825804229037,113.399380178387));
#52493=CARTESIAN_POINT('Ctrl Pts',(17.6508486223648,0.71316562605935,113.427483635222));
#52494=CARTESIAN_POINT('Ctrl Pts',(17.432175698002,0.304188605160904,113.455620456518));
#52495=CARTESIAN_POINT('Ctrl Pts',(17.3995688929116,-0.159048710866342,
113.483794694377));
#52496=CARTESIAN_POINT('Ctrl Pts',(17.5592416108375,-0.595843498412212,
113.512010220208));
#52497=CARTESIAN_POINT('Ctrl Pts',(17.8839047765297,-0.929863593703113,
113.5402708761));
#52498=CARTESIAN_POINT('Ctrl Pts',(18.3174363420886,-1.10244895914806,113.568580611988));
#52499=CARTESIAN_POINT('Ctrl Pts',(18.7845032234939,-1.08288015874688,113.596943024728));
#52500=CARTESIAN_POINT('Ctrl Pts',(19.2036958810281,-0.873830234443041,
113.625362225695));
#52501=CARTESIAN_POINT('Ctrl Pts',(19.5015677804977,-0.511035220651307,
113.653841612173));
#52502=CARTESIAN_POINT('Ctrl Pts',(19.625569402385,-0.057210726531146,113.682385109334));
#52503=CARTESIAN_POINT('Ctrl Pts',(19.5532262978395,0.408801574029359,113.710996276871));
#52504=CARTESIAN_POINT('Ctrl Pts',(19.2962196078634,0.805590455062962,113.739678701328));
#52505=CARTESIAN_POINT('Ctrl Pts',(18.8985263284912,1.06350860478144,113.768436045941));
#52506=CARTESIAN_POINT('Ctrl Pts',(18.5071722498531,1.12444142266846,113.792465688214));
#52507=CARTESIAN_POINT('Ctrl Pts',(18.1989776345572,1.07400338365928,113.811730434757));
#52508=CARTESIAN_POINT('Ctrl Pts',(17.9074645018029,0.960739376980088,113.831023029996));
#52509=CARTESIAN_POINT('Ctrl Pts',(17.5994270430112,0.70815915760555,113.855191843742));
#52510=CARTESIAN_POINT('Ctrl Pts',(17.3852129809237,0.279151779569495,113.884283163333));
#52511=CARTESIAN_POINT('Ctrl Pts',(17.3648125841006,-0.201413575017571,
113.913466255147));
#52512=CARTESIAN_POINT('Ctrl Pts',(17.543062918984,-0.649872702566433,113.942744420078));
#52513=CARTESIAN_POINT('Ctrl Pts',(17.8900876353479,-0.987536991035994,
113.972120816461));
#52514=CARTESIAN_POINT('Ctrl Pts',(18.3463327148162,-1.15459443856777,114.001598506433));
#52515=CARTESIAN_POINT('Ctrl Pts',(18.8327332303177,-1.1206124571982,114.031180517165));
#52516=CARTESIAN_POINT('Ctrl Pts',(19.2643943014772,-0.890100751175115,
114.06086982685));
#52517=CARTESIAN_POINT('Ctrl Pts',(19.5653719416265,-0.501947847935971,
114.09066925157));
#52518=CARTESIAN_POINT('Ctrl Pts',(19.6820042768537,-0.0229147496842619,
114.120581667901));
#52519=CARTESIAN_POINT('Ctrl Pts',(19.5924653448508,0.463866328892549,114.150609737823));
#52520=CARTESIAN_POINT('Ctrl Pts',(19.3108158047468,0.873213114754433,114.180756134765));
#52521=CARTESIAN_POINT('Ctrl Pts',(18.884827463517,1.13286962417431,114.211023428844));
#52522=CARTESIAN_POINT('Ctrl Pts',(18.3879247470357,1.19614313007461,114.241414092977));
#52523=CARTESIAN_POINT('Ctrl Pts',(17.9065295194458,1.05034460153068,114.271930535497));
#52524=CARTESIAN_POINT('Ctrl Pts',(17.525074544366,0.719258169043549,114.302575067548));
#52525=CARTESIAN_POINT('Ctrl Pts',(17.311212189731,0.259295019260713,114.333349916817));
#52526=CARTESIAN_POINT('Ctrl Pts',(17.3038340324676,-0.250078136447899,
114.364257227859));
#52527=CARTESIAN_POINT('Ctrl Pts',(17.5060302198135,-0.720090902958034,
114.395299041011));
#52528=CARTESIAN_POINT('Ctrl Pts',(17.8842069801639,-1.0680223900666,114.42647733462));
#52529=CARTESIAN_POINT('Ctrl Pts',(18.3736961688967,-1.23192189085238,114.457793936704));
#52530=CARTESIAN_POINT('Ctrl Pts',(18.8036898078691,-1.1897113502064,114.484007900284));
#52531=CARTESIAN_POINT('Ctrl Pts',(19.1159133168913,-1.05231178322972,114.50504993148));
#52532=CARTESIAN_POINT('Ctrl Pts',(19.3935460299567,-0.852827854344241,
114.526139457072));
#52533=CARTESIAN_POINT('Ctrl Pts',(19.6510131217686,-0.500999526556579,
114.55259106752));
#52534=CARTESIAN_POINT('Ctrl Pts',(19.7609905689121,0.0129651070626104,
114.584477754316));
#52535=CARTESIAN_POINT('Ctrl Pts',(19.650994915611,0.529347254895316,114.616510721381));
#52536=CARTESIAN_POINT('Ctrl Pts',(19.3382243340085,0.957748579656661,114.648691181518));
#52537=CARTESIAN_POINT('Ctrl Pts',(18.8756353988208,1.22224115354423,114.681020361715));
#52538=CARTESIAN_POINT('Ctrl Pts',(18.3429067772104,1.27497971988073,114.713499322237));
#52539=CARTESIAN_POINT('Ctrl Pts',(17.8327292020459,1.10472610803286,114.746129066567));
#52540=CARTESIAN_POINT('Ctrl Pts',(17.4347759656649,0.739278786151279,114.778910452807));
#52541=CARTESIAN_POINT('Ctrl Pts',(17.2197395303671,0.240806168981795,114.811844294554));
#52542=CARTESIAN_POINT('Ctrl Pts',(17.2263876359587,-0.243861224283583,
114.84125487901));
#52543=CARTESIAN_POINT('Ctrl Pts',(17.3765832012891,-0.636801446696335,
114.86708881416));
#52544=CARTESIAN_POINT('Ctrl Pts',(17.5394691336362,-0.853562773319375,
114.883747582543));
#52545=CARTESIAN_POINT('Ctrl Pts',(17.6708754828836,-0.975913973213227,
114.894874948331));
#52546=CARTESIAN_POINT('Ctrl Pts',(17.7406579614793,-1.03242891223486,114.90044288571));
#52547=CARTESIAN_POINT('Ctrl Pts',(17.8143583148267,-1.08390903483199,114.906015127139));
#52548=CARTESIAN_POINT('Ctrl Pts',(17.9686273982593,-1.17645090895374,114.917168135458));
#52549=CARTESIAN_POINT('Ctrl Pts',(18.2235871886093,-1.27381361087282,114.933929931012));
#52550=CARTESIAN_POINT('Ctrl Pts',(18.5872244681008,-1.30458106909559,114.956347672507));
#52551=CARTESIAN_POINT('Ctrl Pts',(18.9463768488907,-1.23322152774062,114.978834252193));
#52552=CARTESIAN_POINT('Ctrl Pts',(19.2725435869032,-1.06476481773121,115.001389672404));
#52553=CARTESIAN_POINT('Ctrl Pts',(19.5404655740093,-0.811742344080699,
115.024013960787));
#52554=CARTESIAN_POINT('Ctrl Pts',(19.7278646675296,-0.49361337321824,115.046707123689));
#52555=CARTESIAN_POINT('Ctrl Pts',(19.8523533513939,-0.0150590219413064,
115.077056466642));
#52556=CARTESIAN_POINT('Ctrl Pts',(19.7672800481721,0.488492784476201,115.107543396053));
#52557=CARTESIAN_POINT('Ctrl Pts',(19.5239217355454,0.851131103462418,115.134339669597));
#52558=CARTESIAN_POINT('Ctrl Pts',(19.3464502043358,1.02403675952917,115.149686032856));
#52559=CARTESIAN_POINT('Ctrl Pts',(19.1457347753392,1.17063466428336,115.165055294933));
#52560=CARTESIAN_POINT('Ctrl Pts',(18.9456442449245,1.26032940329247,115.178533337362));
#52561=CARTESIAN_POINT('Ctrl Pts',(18.7644374565501,1.30563923878879,115.190107211783));
#52562=CARTESIAN_POINT('Ctrl Pts',(18.6724851125622,1.32194107295301,115.195898442959));
#52563=CARTESIAN_POINT('Ctrl Pts',(18.5949991174864,1.33015007590669,115.20072800507));
#52564=CARTESIAN_POINT('Ctrl Pts',(18.5327430757371,1.33336828052772,115.204593820968));
#52565=CARTESIAN_POINT('Ctrl Pts',(18.2799794944861,1.33819961620997,115.220277475459));
#52566=CARTESIAN_POINT('Ctrl Pts',(17.8197716587963,1.22103049658674,115.2488239801));
#52567=CARTESIAN_POINT('Ctrl Pts',(17.4253298552619,0.855698560316531,115.281163584306));
#52568=CARTESIAN_POINT('Ctrl Pts',(17.2492366094994,0.524494113764414,115.304342264289));
#52569=CARTESIAN_POINT('Ctrl Pts',(17.1891919203476,0.346634023056757,115.315951203043));
#52570=CARTESIAN_POINT('Ctrl Pts',(17.1596329463037,0.199501998041167,115.325250098553));
#52571=CARTESIAN_POINT('Ctrl Pts',(17.1243035124897,-0.0987566443949158,
115.343863735336));
#52572=CARTESIAN_POINT('Ctrl Pts',(17.2116820602607,-0.595538227281773,
115.374199781352));
#52573=CARTESIAN_POINT('Ctrl Pts',(17.6490664555784,-1.14488189393693,115.416413259229));
#52574=CARTESIAN_POINT('Ctrl Pts',(18.2448545926823,-1.39619727372569,115.455299363107));
#52575=CARTESIAN_POINT('Ctrl Pts',(18.8269985365369,-1.37416556805341,115.490800315133));
#52576=CARTESIAN_POINT('Ctrl Pts',(19.3091730618201,-1.16418222178215,115.522865895736));
#52577=CARTESIAN_POINT('Ctrl Pts',(19.6826743730051,-0.790869258048996,
115.555045084909));
#52578=CARTESIAN_POINT('Ctrl Pts',(19.8592522083324,-0.386354923335411,
115.581955060021));
#52579=CARTESIAN_POINT('Ctrl Pts',(19.9047342090055,-0.039775606573619,
115.603538521507));
#52580=CARTESIAN_POINT('Ctrl Pts',(19.8900978097642,0.222324863243005,115.619754213295));
#52581=CARTESIAN_POINT('Ctrl Pts',(19.8373395713028,0.435090922581195,115.633289817848));
#52582=CARTESIAN_POINT('Ctrl Pts',(19.7718546188064,0.597339740059701,115.644132193337));
#52583=CARTESIAN_POINT('Ctrl Pts',(19.651425322384,0.830816794202225,115.660409573376));
#52584=CARTESIAN_POINT('Ctrl Pts',(19.3896969715251,1.13513142859796,115.684876307424));
#52585=CARTESIAN_POINT('Ctrl Pts',(18.9150284789188,1.38619680296976,115.717606636203));
#52586=CARTESIAN_POINT('Ctrl Pts',(18.3797054104768,1.4466716138587,115.750443142464));
#52587=CARTESIAN_POINT('Ctrl Pts',(17.988183958309,1.34188408743399,115.775149099498));
#52588=CARTESIAN_POINT('Ctrl Pts',(17.7539350453868,1.21509730703865,115.791652121032));
#52589=CARTESIAN_POINT('Ctrl Pts',(17.6061813470909,1.11641122904621,115.802662864195));
#52590=CARTESIAN_POINT('Ctrl Pts',(17.3731821120973,0.908319548202519,115.821953447962));
#52591=CARTESIAN_POINT('Ctrl Pts',(17.2162644616103,0.659137577823519,115.839908099308));
#52592=CARTESIAN_POINT('Ctrl Pts',(17.1398169389646,0.449494569945197,115.85374265585));
#52593=CARTESIAN_POINT('Ctrl Pts',(17.1197416648792,0.385640496558971,115.85789451934));
#52594=CARTESIAN_POINT('Ctrl Pts',(17.1027272724371,0.320847543293446,115.862047984451));
#52595=CARTESIAN_POINT('Ctrl Pts',(17.0887358351757,0.255330496363598,115.866202984813));
#52596=CARTESIAN_POINT('Ctrl Pts',(17.0777963741667,0.189195464046852,115.870359570435));
#52597=CARTESIAN_POINT('Ctrl Pts',(17.067418125527,0.100399771748922,115.87590376183));
#52598=CARTESIAN_POINT('Ctrl Pts',(17.0557272856128,-0.145527942481447,
115.891159038571));
#52599=CARTESIAN_POINT('Ctrl Pts',(17.1319155326297,-0.548674192364992,
115.916167747218));
#52600=CARTESIAN_POINT('Ctrl Pts',(17.4236891361341,-1.01332159343547,115.949610144654));
#52601=CARTESIAN_POINT('Ctrl Pts',(17.8662933378701,-1.34016087503944,115.983147288212));
#52602=CARTESIAN_POINT('Ctrl Pts',(18.399223693082,-1.48309771040529,116.016777928577));
#52603=CARTESIAN_POINT('Ctrl Pts',(18.9489636278778,-1.42130150179873,116.050499822527));
#52604=CARTESIAN_POINT('Ctrl Pts',(19.439526569492,-1.16221164480534,116.084311444931));
#52605=CARTESIAN_POINT('Ctrl Pts',(19.7216356020653,-0.834420794277268,
116.110677095138));
#52606=CARTESIAN_POINT('Ctrl Pts',(19.8572233100093,-0.561455048962172,
116.129541929259));
#52607=CARTESIAN_POINT('Ctrl Pts',(19.9376530730783,-0.331222395435849,
116.144645751291));
#52608=CARTESIAN_POINT('Ctrl Pts',(20.0024589418389,0.0939862014720346,
116.171111021937));
#52609=CARTESIAN_POINT('Ctrl Pts',(19.8626252653565,0.708422611339051,116.20900999971));
#52610=CARTESIAN_POINT('Ctrl Pts',(19.3606426600479,1.27757833594637,116.254631289769));
#52611=CARTESIAN_POINT('Ctrl Pts',(18.6457170687546,1.53809320293154,116.300389436894));
#52612=CARTESIAN_POINT('Ctrl Pts',(17.890910575448,1.4246417143608,116.346279427979));
#52613=CARTESIAN_POINT('Ctrl Pts',(17.3697592183846,1.03003291245044,116.385584939065));
#52614=CARTESIAN_POINT('Ctrl Pts',(17.100337406561,0.571607302391164,116.418246772046));
#52615=CARTESIAN_POINT('Ctrl Pts',(16.9582745330856,0.0258686179393441,
116.452879275666));
#52616=CARTESIAN_POINT('Ctrl Pts',(17.079642569554,-0.691275011863127,116.4962606349));
#52617=CARTESIAN_POINT('Ctrl Pts',(17.6627581645516,-1.34421776223012,116.54845478634));
#52618=CARTESIAN_POINT('Ctrl Pts',(18.5058185302644,-1.58735022301968,116.600777176171));
#52619=CARTESIAN_POINT('Ctrl Pts',(19.3508960628413,-1.34420890496649,116.65321930077));
#52620=CARTESIAN_POINT('Ctrl Pts',(19.9385417998377,-0.687144258006306,
116.705772267722));
#52621=CARTESIAN_POINT('Ctrl Pts',(20.0616184527334,0.0381325630880677,
116.74965182232));
#52622=CARTESIAN_POINT('Ctrl Pts',(19.9176287834958,0.592128040193145,116.784801682567));
#52623=CARTESIAN_POINT('Ctrl Pts',(19.6999442414976,0.962347691535422,116.81118670354));
#52624=CARTESIAN_POINT('Ctrl Pts',(19.387187078997,1.25730153941532,116.83759221283));
#52625=CARTESIAN_POINT('Ctrl Pts',(18.8779720660596,1.52166037321083,116.872826686248));
#52626=CARTESIAN_POINT('Ctrl Pts',(18.1399667081786,1.56350792410162,116.9169162291));
#52627=CARTESIAN_POINT('Ctrl Pts',(17.3622686789024,1.13377519632968,116.969889685186));
#52628=CARTESIAN_POINT('Ctrl Pts',(16.9320466679883,0.355566704353337,117.022919441898));
#52629=CARTESIAN_POINT('Ctrl Pts',(16.9818233579469,-0.533172765301191,
117.075996285446));
#52630=CARTESIAN_POINT('Ctrl Pts',(17.4972137629198,-1.25963702599659,117.129110660468));
#52631=CARTESIAN_POINT('Ctrl Pts',(18.3205410600314,-1.60074493849521,117.18225312368));
#52632=CARTESIAN_POINT('Ctrl Pts',(19.199461586771,-1.45143815071003,117.23541411388));
#52633=CARTESIAN_POINT('Ctrl Pts',(19.8643227073833,-0.857296174050731,
117.288584083064));
#52634=CARTESIAN_POINT('Ctrl Pts',(20.1111513110505,-0.000491905914397789,
117.341753458203));
#52635=CARTESIAN_POINT('Ctrl Pts',(19.8643244718875,0.856132975128993,117.394912684707));
#52636=CARTESIAN_POINT('Ctrl Pts',(19.1998096494292,1.44990225773341,117.448052198099));
#52637=CARTESIAN_POINT('Ctrl Pts',(18.3217251143232,1.599013628145,117.501162465982));
#52638=CARTESIAN_POINT('Ctrl Pts',(17.499504374338,1.25832728231969,117.554234001358));
#52639=CARTESIAN_POINT('Ctrl Pts',(16.985055982408,0.533061319756643,117.60725735614));
#52640=CARTESIAN_POINT('Ctrl Pts',(16.9353935453568,-0.353785275682392,
117.660223128507));
#52641=CARTESIAN_POINT('Ctrl Pts',(17.3646646422282,-1.13011770093016,117.713122006794));
#52642=CARTESIAN_POINT('Ctrl Pts',(18.1400392517145,-1.55845623704423,117.76594474964));
#52643=CARTESIAN_POINT('Ctrl Pts',(19.0230777257463,-1.50863468531329,117.818682215354));
#52644=CARTESIAN_POINT('Ctrl Pts',(19.7428658914057,-0.997619269505286,
117.871325327931));
#52645=CARTESIAN_POINT('Ctrl Pts',(20.0799462528815,-0.183426406491474,
117.923865215528));
#52646=CARTESIAN_POINT('Ctrl Pts',(19.9567569394742,0.538729417132324,117.967555008894));
#52647=CARTESIAN_POINT('Ctrl Pts',(19.6400599565462,1.01030681822159,118.002446570801));
#52648=CARTESIAN_POINT('Ctrl Pts',(19.2073385738753,1.37731958827904,118.03729626475));
#52649=CARTESIAN_POINT('Ctrl Pts',(18.5067297996373,1.57915592164188,118.080777892618));
#52650=CARTESIAN_POINT('Ctrl Pts',(17.6681360568722,1.33710476368857,118.132817962888));
#52651=CARTESIAN_POINT('Ctrl Pts',(17.0885466977777,0.6880330974798,118.184712313374));
#52652=CARTESIAN_POINT('Ctrl Pts',(16.9435495706207,-0.167492528644316,
118.236452721141));
#52653=CARTESIAN_POINT('Ctrl Pts',(17.2749324092385,-0.966447647923809,
118.288031455808));
#52654=CARTESIAN_POINT('Ctrl Pts',(17.9782861905575,-1.46502430150085,118.33944080786));
#52655=CARTESIAN_POINT('Ctrl Pts',(18.8361224498172,-1.51274888582587,118.390673366568));
#52656=CARTESIAN_POINT('Ctrl Pts',(19.5851780705485,-1.09829472567512,118.441721870754));
#52657=CARTESIAN_POINT('Ctrl Pts',(19.9973084426146,-0.351551880340416,
118.492579360892));
#52658=CARTESIAN_POINT('Ctrl Pts',(19.9492369017591,0.496527279998027,118.543238980189));
#52659=CARTESIAN_POINT('Ctrl Pts',(19.4591265716024,1.1865303680748,118.59369432018));
#52660=CARTESIAN_POINT('Ctrl Pts',(18.8104123489689,1.45452734640773,118.635564768299));
#52661=CARTESIAN_POINT('Ctrl Pts',(18.2668600482904,1.43813882096128,118.66895295447));
#52662=CARTESIAN_POINT('Ctrl Pts',(17.8793606825511,1.3149779455841,118.69393898397));
#52663=CARTESIAN_POINT('Ctrl Pts',(17.5418800138726,1.08918872056738,118.718869663376));
#52664=CARTESIAN_POINT('Ctrl Pts',(17.2806722359481,0.779868090767067,118.743743756155));
#52665=CARTESIAN_POINT('Ctrl Pts',(17.115688834786,0.41095174070353,118.768561126351));
#52666=CARTESIAN_POINT('Ctrl Pts',(17.059420080157,0.0118658393363464,118.793320604163));
#52667=CARTESIAN_POINT('Ctrl Pts',(17.1156776902122,-0.386417116216434,
118.818022013955));
#52668=CARTESIAN_POINT('Ctrl Pts',(17.2523308733496,-0.691438028513019,
118.838557160723));
#52669=CARTESIAN_POINT('Ctrl Pts',(17.4087191006526,-0.905517574177908,
118.854955848303));
#52670=CARTESIAN_POINT('Ctrl Pts',(17.5933085235369,-1.09500930757365,118.871334137985));
#52671=CARTESIAN_POINT('Ctrl Pts',(17.9803266474948,-1.35467533102602,118.899944149037));
#52672=CARTESIAN_POINT('Ctrl Pts',(18.6532437648212,-1.46879524415219,118.940663432495));
#52673=CARTESIAN_POINT('Ctrl Pts',(19.4066095777413,-1.15607767482664,118.989279524881));
#52674=CARTESIAN_POINT('Ctrl Pts',(19.7969063670871,-0.604727996663488,
119.029583574239));
#52675=CARTESIAN_POINT('Ctrl Pts',(19.8852025512401,-0.15555160666413,119.05768465636));
#52676=CARTESIAN_POINT('Ctrl Pts',(19.88174482432,0.103206678710061,119.073710544167));
#52677=CARTESIAN_POINT('Ctrl Pts',(19.8420242547932,0.359028078531283,119.089714694668));
#52678=CARTESIAN_POINT('Ctrl Pts',(19.7258720066209,0.662275611606032,119.109679686885));
#52679=CARTESIAN_POINT('Ctrl Pts',(19.4145468469588,1.07750284183372,119.141536856276));
#52680=CARTESIAN_POINT('Ctrl Pts',(18.8325235269669,1.39878522268015,119.181194851707));
#52681=CARTESIAN_POINT('Ctrl Pts',(18.0400340075687,1.35363547075075,119.228519889168));
#52682=CARTESIAN_POINT('Ctrl Pts',(17.3967718435735,0.89641934013867,119.275577945121));
#52683=CARTESIAN_POINT('Ctrl Pts',(17.1472193984553,0.292229951924935,119.314568595929));
#52684=CARTESIAN_POINT('Ctrl Pts',(17.1625698892113,-0.213333516171699,
119.345625653156));
#52685=CARTESIAN_POINT('Ctrl Pts',(17.2578325055986,-0.513471977461749,
119.364979574332));
#52686=CARTESIAN_POINT('Ctrl Pts',(17.3665030300232,-0.703170857591556,
119.378497592737));
#52687=CARTESIAN_POINT('Ctrl Pts',(17.4391238043473,-0.804166878514464,
119.386213631278));
#52688=CARTESIAN_POINT('Ctrl Pts',(17.5187561772849,-0.899766250215976,
119.393923967814));
#52689=CARTESIAN_POINT('Ctrl Pts',(17.630281948166,-1.00820403810343,119.403551172218));
#52690=CARTESIAN_POINT('Ctrl Pts',(17.8309717833451,-1.15490872115532,119.418932014259));
#52691=CARTESIAN_POINT('Ctrl Pts',(18.1160464864079,-1.28243128828034,119.438115227001));
#52692=CARTESIAN_POINT('Ctrl Pts',(18.4860686310391,-1.33458226019453,119.461066507994));
#52693=CARTESIAN_POINT('Ctrl Pts',(18.8549377775812,-1.28242608286313,119.483949129966));
#52694=CARTESIAN_POINT('Ctrl Pts',(19.1939409847697,-1.13065085353412,119.506762964988));
#52695=CARTESIAN_POINT('Ctrl Pts',(19.4768178449134,-0.891673212986614,
119.52950802525));
#52696=CARTESIAN_POINT('Ctrl Pts',(19.6818581712436,-0.584671279112933,
119.552184188786));
#52697=CARTESIAN_POINT('Ctrl Pts',(19.7935622110083,-0.233953471223591,
119.574791531524));
#52698=CARTESIAN_POINT('Ctrl Pts',(19.8037606611236,0.132828699787753,119.597329945963));
#52699=CARTESIAN_POINT('Ctrl Pts',(19.7275779091676,0.428031572432683,119.616054659699));
#52700=CARTESIAN_POINT('Ctrl Pts',(19.619614446759,0.644065603823603,119.630999964254));
#52701=CARTESIAN_POINT('Ctrl Pts',(19.4488281681557,0.89250425474605,119.64965300798));
#52702=CARTESIAN_POINT('Ctrl Pts',(19.1170401588768,1.16456978521157,119.675687037975));
#52703=CARTESIAN_POINT('Ctrl Pts',(18.5871553030014,1.30892105032127,119.709005045111));
#52704=CARTESIAN_POINT('Ctrl Pts',(18.0470739154042,1.22466017262848,119.742169110698));
#52705=CARTESIAN_POINT('Ctrl Pts',(17.5906153353427,0.92852820021813,119.775179782028));
#52706=CARTESIAN_POINT('Ctrl Pts',(17.2962939028983,0.473891549786357,119.80803764787));
#52707=CARTESIAN_POINT('Ctrl Pts',(17.2137278862079,-0.0588069964784256,
119.840743488334));
#52708=CARTESIAN_POINT('Ctrl Pts',(17.3552583261151,-0.576413195052804,
119.873298037803));
#52709=CARTESIAN_POINT('Ctrl Pts',(17.6378267009486,-0.920280590517876,
119.900301683486));
#52710=CARTESIAN_POINT('Ctrl Pts',(17.9322059358076,-1.10769984563428,119.921829832672));
#52711=CARTESIAN_POINT('Ctrl Pts',(18.2582726230055,-1.22986089927834,119.943308554429));
#52712=CARTESIAN_POINT('Ctrl Pts',(18.6988777360301,-1.24826140338436,119.970064276947));
#52713=CARTESIAN_POINT('Ctrl Pts',(19.1882573017696,-1.05324218253824,120.002024304111));
#52714=CARTESIAN_POINT('Ctrl Pts',(19.5536298555227,-0.677126307322699,
120.033838749918));
#52715=CARTESIAN_POINT('Ctrl Pts',(19.7327011533039,-0.186782542043285,
120.065509088722));
#52716=CARTESIAN_POINT('Ctrl Pts',(19.6960404522687,0.331577532740455,120.0970368287));
#52717=CARTESIAN_POINT('Ctrl Pts',(19.4519605062165,0.787710743631352,120.128423616381));
#52718=CARTESIAN_POINT('Ctrl Pts',(19.0446667619321,1.10296875506974,120.159671158499));
#52719=CARTESIAN_POINT('Ctrl Pts',(18.5463561410001,1.22382983664122,120.19078130098));
#52720=CARTESIAN_POINT('Ctrl Pts',(18.0442916571447,1.13105334473252,120.221755909485));
#52721=CARTESIAN_POINT('Ctrl Pts',(17.6955585720856,0.890589398969558,120.247456881368));
#52722=CARTESIAN_POINT('Ctrl Pts',(17.494206304073,0.626324017549734,120.267951925713));
#52723=CARTESIAN_POINT('Ctrl Pts',(17.3521978134265,0.326733896928664,120.288403487671));
#52724=CARTESIAN_POINT('Ctrl Pts',(17.2994574052005,-0.089976635869453,
120.313887268105));
#52725=CARTESIAN_POINT('Ctrl Pts',(17.4453910079367,-0.570256699169521,
120.344340822402));
#52726=CARTESIAN_POINT('Ctrl Pts',(17.7733937212861,-0.947489949761874,
120.374669791192));
#52727=CARTESIAN_POINT('Ctrl Pts',(18.2250498759407,-1.15701559211397,120.404876598007));
#52728=CARTESIAN_POINT('Ctrl Pts',(18.7209167059739,-1.16376250471033,120.43496378867));
#52729=CARTESIAN_POINT('Ctrl Pts',(19.1745246697594,-0.968157083714777,
120.46493395781));
#52730=CARTESIAN_POINT('Ctrl Pts',(19.5074032171353,-0.605727211221481,
120.494789798378));
#52731=CARTESIAN_POINT('Ctrl Pts',(19.6626391866769,-0.140691381829317,
120.524534069588));
#52732=CARTESIAN_POINT('Ctrl Pts',(19.6145749646053,0.345408120183416,120.554169611841));
#52733=CARTESIAN_POINT('Ctrl Pts',(19.3730279409814,0.767967837218571,120.583699337212));
#52734=CARTESIAN_POINT('Ctrl Pts',(18.981327184557,1.05401910504784,120.613126231449));
#52735=CARTESIAN_POINT('Ctrl Pts',(18.5085627461879,1.15479574234016,120.64245334912));
#52736=CARTESIAN_POINT('Ctrl Pts',(18.037426479005,1.05402306854266,120.671683811955));
#52737=CARTESIAN_POINT('Ctrl Pts',(17.6497818027982,0.770520108026078,120.700820806668));
#52738=CARTESIAN_POINT('Ctrl Pts',(17.4124738708295,0.354706256959195,120.729867584727));
#52739=CARTESIAN_POINT('Ctrl Pts',(17.3658345014046,-0.120342674613531,
120.758827458907));
#52740=CARTESIAN_POINT('Ctrl Pts',(17.5168518221837,-0.571705086255479,
120.787703800973));
#52741=CARTESIAN_POINT('Ctrl Pts',(17.8381564074402,-0.921050935566984,
120.816500038417));
#52742=CARTESIAN_POINT('Ctrl Pts',(18.2729637820143,-1.10819891035518,120.845219652361));
#52743=CARTESIAN_POINT('Ctrl Pts',(18.7450836643294,-1.10145297227955,120.873866177775));
#52744=CARTESIAN_POINT('Ctrl Pts',(19.1722351044748,-0.902949084941853,
120.902443198341));
#52745=CARTESIAN_POINT('Ctrl Pts',(19.4803468036944,-0.54811414646913,120.930954347204));
#52746=CARTESIAN_POINT('Ctrl Pts',(19.6163641816792,-0.0993634013560132,
120.959403296642));
#52747=CARTESIAN_POINT('Ctrl Pts',(19.5573567106693,0.36484925508517,120.987793769242));
#52748=CARTESIAN_POINT('Ctrl Pts',(19.3143653934618,0.763705712028081,121.016129512177));
#52749=CARTESIAN_POINT('Ctrl Pts',(18.9303516375633,1.0280578161787,121.044414340805));
#52750=CARTESIAN_POINT('Ctrl Pts',(18.4726214819807,1.1123686635717,121.072652047794));
#52751=CARTESIAN_POINT('Ctrl Pts',(18.0210682203609,1.00254924865375,121.100846563677));
#52752=CARTESIAN_POINT('Ctrl Pts',(17.6542606193921,0.718265809992657,121.129001647677));
#52753=CARTESIAN_POINT('Ctrl Pts',(17.4358298475876,0.309493931538336,121.157121462298));
#52754=CARTESIAN_POINT('Ctrl Pts',(17.4034366817011,-0.152362004672267,
121.185209478558));
#52755=CARTESIAN_POINT('Ctrl Pts',(17.5226227411507,-0.478090876422412,
121.206255356037));
#52756=CARTESIAN_POINT('Ctrl Pts',(17.6531201906185,-0.663090893144466,
121.22027789221));
#52757=CARTESIAN_POINT('Ctrl Pts',(17.7524655785764,-0.776636580209785,
121.229625106739));
#52758=CARTESIAN_POINT('Ctrl Pts',(17.9560938470234,-0.94641425946181,121.245976987179));
#52759=CARTESIAN_POINT('Ctrl Pts',(18.3135998936201,-1.08871343434314,121.269325120801));
#52760=CARTESIAN_POINT('Ctrl Pts',(18.7747781066023,-1.06924543466266,121.297327130536));
#52761=CARTESIAN_POINT('Ctrl Pts',(19.1875682929109,-0.863261922321633,
121.325317720602));
#52762=CARTESIAN_POINT('Ctrl Pts',(19.480175414768,-0.506709737445342,121.353300778039));
#52763=CARTESIAN_POINT('Ctrl Pts',(19.6016091931846,-0.0618147900173241,
121.38128041041));
#52764=CARTESIAN_POINT('Ctrl Pts',(19.5307495553282,0.393896407522541,121.409260613888));
#52765=CARTESIAN_POINT('Ctrl Pts',(19.2798982106118,0.78098259809769,121.437245445173));
#52766=CARTESIAN_POINT('Ctrl Pts',(18.8927083288752,1.03193571113476,121.465238926932));
#52767=CARTESIAN_POINT('Ctrl Pts',(18.4365809280527,1.10289372174427,121.493245092408));
#52768=CARTESIAN_POINT('Ctrl Pts',(17.9909862406699,0.981295289662669,121.521267957359));
#52769=CARTESIAN_POINT('Ctrl Pts',(17.6336525893153,0.688090158880322,121.54931152847));
#52770=CARTESIAN_POINT('Ctrl Pts',(17.4270545585554,0.274145584653852,121.577379799094));
#52771=CARTESIAN_POINT('Ctrl Pts',(17.407521715122,-0.188551808914773,121.605476744048));
#52772=CARTESIAN_POINT('Ctrl Pts',(17.578871006045,-0.619374849770778,121.633606325448));
#52773=CARTESIAN_POINT('Ctrl Pts',(17.9116705005978,-0.943060979454274,
121.661772468717));
#52774=CARTESIAN_POINT('Ctrl Pts',(18.3482760990906,-1.10282238037483,121.689979100292));
#52775=CARTESIAN_POINT('Ctrl Pts',(18.8127861354656,-1.07027500003871,121.718230068639));
#52776=CARTESIAN_POINT('Ctrl Pts',(19.2241926323308,-0.850473759884222,
121.746529289687));
#52777=CARTESIAN_POINT('Ctrl Pts',(19.5104728423211,-0.481127471064448,
121.774880465549));
#52778=CARTESIAN_POINT('Ctrl Pts',(19.6211489336822,-0.0261818239526985,
121.803287602493));
#52779=CARTESIAN_POINT('Ctrl Pts',(19.5361773084952,0.435267939246471,121.831754120211));
#52780=CARTESIAN_POINT('Ctrl Pts',(19.2695609307072,0.822620385440146,121.860284019395));
#52781=CARTESIAN_POINT('Ctrl Pts',(18.8670431140771,1.06787405410294,121.888880821572));
#52782=CARTESIAN_POINT('Ctrl Pts',(18.3983088047807,1.12748222485771,121.917548158767));
#52783=CARTESIAN_POINT('Ctrl Pts',(17.9449368652974,0.990091865801272,121.946289639226));
#52784=CARTESIAN_POINT('Ctrl Pts',(17.5862538567715,0.678671854848107,121.975108743805));
#52785=CARTESIAN_POINT('Ctrl Pts',(17.3854827140722,0.24670147648264,122.004008943349));
#52786=CARTESIAN_POINT('Ctrl Pts',(17.3786328692577,-0.230991019697471,
122.032993686558));
#52787=CARTESIAN_POINT('Ctrl Pts',(17.5680585071982,-0.67115046067875,122.062066264703));
#52788=CARTESIAN_POINT('Ctrl Pts',(17.9218464717271,-0.996572482097319,
122.091230038573));
#52789=CARTESIAN_POINT('Ctrl Pts',(18.3791686838937,-1.14960748605158,122.120488198196));
#52790=CARTESIAN_POINT('Ctrl Pts',(18.8607119999246,-1.10235313954737,122.14984391457));
#52791=CARTESIAN_POINT('Ctrl Pts',(19.2823992466147,-0.861717252928226,
122.179300327631));
#52792=CARTESIAN_POINT('Ctrl Pts',(19.5700353909992,-0.468457924978318,
122.208860408707));
#52793=CARTESIAN_POINT('Ctrl Pts',(19.67233106885,0.0097073705472888,122.238527197898));
#52794=CARTESIAN_POINT('Ctrl Pts',(19.5700316977566,0.489712410185742,122.268303502345));
#52795=CARTESIAN_POINT('Ctrl Pts',(19.2795029754614,0.887577837959271,122.298192256778));
#52796=CARTESIAN_POINT('Ctrl Pts',(18.8501763787566,1.13301634843011,122.328196028424));
#52797=CARTESIAN_POINT('Ctrl Pts',(18.3561006293489,1.18188281079065,122.35831766051));
#52798=CARTESIAN_POINT('Ctrl Pts',(17.8832822795417,1.02407533627195,122.388559619116));
#52799=CARTESIAN_POINT('Ctrl Pts',(17.5146580665992,0.685512525443912,122.418924457051));
#52800=CARTESIAN_POINT('Ctrl Pts',(17.3156519974485,0.224081959662186,122.44941458419));
#52801=CARTESIAN_POINT('Ctrl Pts',(17.3217321515332,-0.224535868550723,
122.476630331878));
#52802=CARTESIAN_POINT('Ctrl Pts',(17.4608369291701,-0.587814069483905,
122.500528323594));
#52803=CARTESIAN_POINT('Ctrl Pts',(17.7282696593147,-0.944769846820399,
122.527918057151));
#52804=CARTESIAN_POINT('Ctrl Pts',(18.232480082639,-1.22418021862519,122.562302776727));
#52805=CARTESIAN_POINT('Ctrl Pts',(18.9275391443125,-1.18570268762942,122.603805135729));
#52806=CARTESIAN_POINT('Ctrl Pts',(19.4987907286606,-0.781035799526716,
122.645552786729));
#52807=CARTESIAN_POINT('Ctrl Pts',(19.7688835459748,-0.130648543500597,
122.687549892942));
#52808=CARTESIAN_POINT('Ctrl Pts',(19.6507983536421,0.568114068619408,122.72980038736));
#52809=CARTESIAN_POINT('Ctrl Pts',(19.2553118912251,1.01114100863068,122.76522328566));
#52810=CARTESIAN_POINT('Ctrl Pts',(18.8317674110158,1.19977536711199,122.79369172896));
#52811=CARTESIAN_POINT('Ctrl Pts',(18.4994714464154,1.24719930072615,122.814315320483));
#52812=CARTESIAN_POINT('Ctrl Pts',(18.1788486649134,1.20667156059022,122.83420320996));
#52813=CARTESIAN_POINT('Ctrl Pts',(17.7925371098079,1.05582037916025,122.859729393806));
#52814=CARTESIAN_POINT('Ctrl Pts',(17.4016249448576,0.693715854025999,122.89176826119));
#52815=CARTESIAN_POINT('Ctrl Pts',(17.2307330623022,0.185953345830622,122.92398349555));
#52816=CARTESIAN_POINT('Ctrl Pts',(17.2523323040732,-0.23399781816306,122.949862141601));
#52817=CARTESIAN_POINT('Ctrl Pts',(17.3758319956166,-0.63702041854291,122.975812083321));
#52818=CARTESIAN_POINT('Ctrl Pts',(17.7132270565981,-1.06094316132434,123.008383394391));
#52819=CARTESIAN_POINT('Ctrl Pts',(18.2652129563259,-1.29379566909652,123.044409330373));
#52820=CARTESIAN_POINT('Ctrl Pts',(18.8048202871323,-1.27341194899918,123.077317844062));
#52821=CARTESIAN_POINT('Ctrl Pts',(19.2520591589225,-1.0786731726488,123.107057458581));
#52822=CARTESIAN_POINT('Ctrl Pts',(19.5986320076058,-0.732275146337212,
123.136919222601));
#52823=CARTESIAN_POINT('Ctrl Pts',(19.7955049190142,-0.281541487902919,
123.166903310585));
#52824=CARTESIAN_POINT('Ctrl Pts',(19.814175494069,0.212080051862212,123.197009803247));
#52825=CARTESIAN_POINT('Ctrl Pts',(19.6505357555705,0.680199603450974,123.22723875367));
#52826=CARTESIAN_POINT('Ctrl Pts',(19.3800198693595,0.994891712538085,123.252531518524));
#52827=CARTESIAN_POINT('Ctrl Pts',(19.1048855509728,1.17460736001555,123.272826913899));
#52828=CARTESIAN_POINT('Ctrl Pts',(18.7502795847464,1.32221520931078,123.296552374618));
#52829=CARTESIAN_POINT('Ctrl Pts',(18.2134028163266,1.34942925716205,123.328869397769));
#52830=CARTESIAN_POINT('Ctrl Pts',(17.7009999455689,1.10290673401308,123.363067775711));
#52831=CARTESIAN_POINT('Ctrl Pts',(17.3976492612122,0.775343454126338,123.390534343115));
#52832=CARTESIAN_POINT('Ctrl Pts',(17.2373156796508,0.480844927046111,123.411188117109));
#52833=CARTESIAN_POINT('Ctrl Pts',(17.1258389632255,0.0460476148377275,
123.438798023514));
#52834=CARTESIAN_POINT('Ctrl Pts',(17.190043079014,-0.468229286583892,123.469979677869));
#52835=CARTESIAN_POINT('Ctrl Pts',(17.4941741697257,-0.951758531768305,
123.504781176556));
#52836=CARTESIAN_POINT('Ctrl Pts',(17.9260851237358,-1.27106107307662,123.537531680416));
#52837=CARTESIAN_POINT('Ctrl Pts',(18.4738055254567,-1.40450128521582,123.571728513849));
#52838=CARTESIAN_POINT('Ctrl Pts',(19.0518747398078,-1.29815338903981,123.607389463288));
#52839=CARTESIAN_POINT('Ctrl Pts',(19.4975667911712,-0.991471108595277,
123.64021397565));
#52840=CARTESIAN_POINT('Ctrl Pts',(19.718108765147,-0.668458656443225,123.664171779265));
#52841=CARTESIAN_POINT('Ctrl Pts',(19.840684276858,-0.369704589488725,123.684176966688));
#52842=CARTESIAN_POINT('Ctrl Pts',(19.9012468618966,-0.0656783463889097,
123.703216913146));
#52843=CARTESIAN_POINT('Ctrl Pts',(19.8683061355372,0.325537213186654,123.727331521864));
#52844=CARTESIAN_POINT('Ctrl Pts',(19.7280021633901,0.693317586446537,123.751509567709));
#52845=CARTESIAN_POINT('Ctrl Pts',(19.4907339764757,1.00870957723937,123.775750778072));
#52846=CARTESIAN_POINT('Ctrl Pts',(19.1746344843562,1.24667974067477,123.800054570196));
#52847=CARTESIAN_POINT('Ctrl Pts',(18.8349045453036,1.37646300010242,123.822389896322));
#52848=CARTESIAN_POINT('Ctrl Pts',(18.5073833848405,1.41556608351708,123.842739728062));
#52849=CARTESIAN_POINT('Ctrl Pts',(18.1123610183889,1.37979837018668,123.867205371628));
#52850=CARTESIAN_POINT('Ctrl Pts',(17.6480520706786,1.18013603372677,123.89787276461));
#52851=CARTESIAN_POINT('Ctrl Pts',(17.2358803945236,0.732012860791261,123.934808434271));
#52852=CARTESIAN_POINT('Ctrl Pts',(17.0419794776495,0.152653694038211,123.971876745333));
#52853=CARTESIAN_POINT('Ctrl Pts',(17.10185151608,-0.45756914112672,124.009075627682));
#52854=CARTESIAN_POINT('Ctrl Pts',(17.4067903543957,-0.991921667797129,
124.046402830605));
#52855=CARTESIAN_POINT('Ctrl Pts',(17.9050692573643,-1.35635713407927,124.08385606453));
#52856=CARTESIAN_POINT('Ctrl Pts',(18.5107335847068,-1.48590165559992,124.121432928518));
#52857=CARTESIAN_POINT('Ctrl Pts',(19.1184385180564,-1.3563507502972,124.159130952342));
#52858=CARTESIAN_POINT('Ctrl Pts',(19.6218022289785,-0.98872576919303,124.196947576568));
#52859=CARTESIAN_POINT('Ctrl Pts',(19.9320540444447,-0.445907038184834,
124.234880164305));
#52860=CARTESIAN_POINT('Ctrl Pts',(19.9937135700085,0.178148153659393,124.272925997681));
#52861=CARTESIAN_POINT('Ctrl Pts',(19.7945218608488,0.774684491212139,124.311082283028));
#52862=CARTESIAN_POINT('Ctrl Pts',(19.3678473665426,1.23913646259581,124.349346152036));
#52863=CARTESIAN_POINT('Ctrl Pts',(18.7870971810712,1.48948517765483,124.387714664201));
#52864=CARTESIAN_POINT('Ctrl Pts',(18.1530697283671,1.48076648367652,124.426184806719));
#52865=CARTESIAN_POINT('Ctrl Pts',(17.5764302450274,1.21315420572873,124.464753497712));
#52866=CARTESIAN_POINT('Ctrl Pts',(17.1583610032014,0.73216643659731,124.503417588286));
#52867=CARTESIAN_POINT('Ctrl Pts',(16.9727754031592,0.120915171124057,124.542173865763));
#52868=CARTESIAN_POINT('Ctrl Pts',(17.053228230474,-0.514279241981028,124.581019055523));
#52869=CARTESIAN_POINT('Ctrl Pts',(17.3868443511107,-1.06241526162645,124.619949821452));
#52870=CARTESIAN_POINT('Ctrl Pts',(17.9163655702989,-1.42724443394371,124.658962768982));
#52871=CARTESIAN_POINT('Ctrl Pts',(18.5499933474172,-1.54420384030286,124.698054447786));
#52872=CARTESIAN_POINT('Ctrl Pts',(19.177333010067,-1.39186200173388,124.737221354945));
#52873=CARTESIAN_POINT('Ctrl Pts',(19.6886650872882,-0.995845166220365,
124.776459937328));
#52874=CARTESIAN_POINT('Ctrl Pts',(19.9941729942927,-0.424524481016298,
124.815766591911));
#52875=CARTESIAN_POINT('Ctrl Pts',(20.0397508728227,0.222810121504123,124.855137669041));
#52876=CARTESIAN_POINT('Ctrl Pts',(19.816603606709,0.833240192938617,124.894569475321));
#52877=CARTESIAN_POINT('Ctrl Pts',(19.3629322894934,1.29995631129024,124.934058276943));
#52878=CARTESIAN_POINT('Ctrl Pts',(18.7573836344576,1.5409857282793,124.973600302423));
#52879=CARTESIAN_POINT('Ctrl Pts',(18.1053883878064,1.51361956558236,125.013191742918));
#52880=CARTESIAN_POINT('Ctrl Pts',(17.5207664641707,1.22199509521115,125.05282875548));
#52881=CARTESIAN_POINT('Ctrl Pts',(17.1058149097213,0.716484110643661,125.092507466257));
#52882=CARTESIAN_POINT('Ctrl Pts',(16.9333696386985,0.0849747734438613,
125.132223973764));
#52883=CARTESIAN_POINT('Ctrl Pts',(17.0339933882744,-0.562441260921414,
125.171974352057));
#52884=CARTESIAN_POINT('Ctrl Pts',(17.390548421764,-1.11270270209401,125.211754651068));
#52885=CARTESIAN_POINT('Ctrl Pts',(17.9411197173863,-1.46956608382521,125.251560899613));
#52886=CARTESIAN_POINT('Ctrl Pts',(18.5897895263485,-1.570476072409,125.291389109069));
#52887=CARTESIAN_POINT('Ctrl Pts',(19.2233842915933,-1.39755490178516,125.331235276345));
#52888=CARTESIAN_POINT('Ctrl Pts',(19.7312635698777,-0.980776005995196,
125.371095387577));
#52889=CARTESIAN_POINT('Ctrl Pts',(20.0246830575117,-0.392757399099882,
125.410965418396));
#52890=CARTESIAN_POINT('Ctrl Pts',(20.0523356967461,0.263918904922262,125.45084133669));
#52891=CARTESIAN_POINT('Ctrl Pts',(19.8093430859602,0.874642369917206,125.490719106622));
#52892=CARTESIAN_POINT('Ctrl Pts',(19.338117939541,1.33282146051242,125.530594691345));
#52893=CARTESIAN_POINT('Ctrl Pts',(18.7209447529552,1.55852867925055,125.570464057095));
#52894=CARTESIAN_POINT('Ctrl Pts',(18.0655795919603,1.51247445386863,125.610323173319));
#52895=CARTESIAN_POINT('Ctrl Pts',(17.4863946151243,1.20286152519264,125.650168015395));
#52896=CARTESIAN_POINT('Ctrl Pts',(17.08437402484,0.68392126836871,125.689994568545));
#52897=CARTESIAN_POINT('Ctrl Pts',(16.929468039317,0.0463936644794652,125.729798830645));
#52898=CARTESIAN_POINT('Ctrl Pts',(17.0483951994113,-0.598374148289317,
125.769576816299));
#52899=CARTESIAN_POINT('Ctrl Pts',(17.4200245578257,-1.13791782047621,125.809324557098));
#52900=CARTESIAN_POINT('Ctrl Pts',(17.9791373208165,-1.47831538930677,125.849038104005));
#52901=CARTESIAN_POINT('Ctrl Pts',(18.6278970714101,-1.56057234280656,125.888713531393));
#52902=CARTESIAN_POINT('Ctrl Pts',(19.2530067739201,-1.37086750720055,125.928346939608));
#52903=CARTESIAN_POINT('Ctrl Pts',(19.7455372169818,-0.942876630111474,
125.967934459145));
#52904=CARTESIAN_POINT('Ctrl Pts',(20.0199490743694,-0.351783080761525,
126.007472250877));
#52905=CARTESIAN_POINT('Ctrl Pts',(20.0289798900698,0.298956955377318,126.046956508333));
#52906=CARTESIAN_POINT('Ctrl Pts',(19.7717997014967,0.895760095633046,126.086383461411));
#52907=CARTESIAN_POINT('Ctrl Pts',(19.2940254107556,1.33478268233592,126.125749379074));
#52908=CARTESIAN_POINT('Ctrl Pts',(18.6796145554874,1.54002675564106,126.165050573152));
#52909=CARTESIAN_POINT('Ctrl Pts',(18.0360819363224,1.47652170954235,126.204283398858));
#52910=CARTESIAN_POINT('Ctrl Pts',(17.4756475553532,1.15629106504151,126.243444256678));
#52911=CARTESIAN_POINT('Ctrl Pts',(17.0956282178994,0.636085037276605,126.282529595954));
#52912=CARTESIAN_POINT('Ctrl Pts',(16.9615059717559,0.00730541265974819,
126.321535917403));
#52913=CARTESIAN_POINT('Ctrl Pts',(17.0956248257272,-0.62008509447962,126.360459776655));
#52914=CARTESIAN_POINT('Ctrl Pts',(17.4734700822054,-1.13683065414485,126.399297784896));
#52915=CARTESIAN_POINT('Ctrl Pts',(18.0281490556148,-1.45344460991142,126.43804661051));
#52916=CARTESIAN_POINT('Ctrl Pts',(18.6622538987967,-1.51573411677912,126.476702982318));
#52917=CARTESIAN_POINT('Ctrl Pts',(19.2649987922204,-1.31408906543418,126.515263692086));
#52918=CARTESIAN_POINT('Ctrl Pts',(19.731610851688,-0.884941277427619,126.553725597545));
#52919=CARTESIAN_POINT('Ctrl Pts',(19.9815743866459,-0.304177503036399,
126.592085623336));
#52920=CARTESIAN_POINT('Ctrl Pts',(19.9725463963688,0.326301385032026,126.630340762356));
#52921=CARTESIAN_POINT('Ctrl Pts',(19.7075342584873,0.896490569366356,126.668488078281));
#52922=CARTESIAN_POINT('Ctrl Pts',(19.2341192578344,1.30750680377586,126.70652470863));
#52923=CARTESIAN_POINT('Ctrl Pts',(18.635904943503,1.48876449058148,126.744447866081));
#52924=CARTESIAN_POINT('Ctrl Pts',(18.0177319941314,1.41011257811453,126.782254841743));
#52925=CARTESIAN_POINT('Ctrl Pts',(17.4872732878289,1.08684624833835,126.819943002246));
#52926=CARTESIAN_POINT('Ctrl Pts',(17.1362552397195,0.576755853808402,126.857509799078));
#52927=CARTESIAN_POINT('Ctrl Pts',(17.0245670874354,-0.0302098809080251,
126.894952757996));
#52928=CARTESIAN_POINT('Ctrl Pts',(17.1700489322066,-0.62783585744949,126.932269505093));
#52929=CARTESIAN_POINT('Ctrl Pts',(17.5456363009555,-1.11223706751881,126.969457722877));
#52930=CARTESIAN_POINT('Ctrl Pts',(18.0844346743395,-1.39997160299426,127.006515235409));
#52931=CARTESIAN_POINT('Ctrl Pts',(18.6915498483127,-1.44237197701727,127.043439851825));
#52932=CARTESIAN_POINT('Ctrl Pts',(19.2610012684699,-1.2338864451594,127.080229666573));
#52933=CARTESIAN_POINT('Ctrl Pts',(19.6217471892279,-0.882743718249303,
127.110773685143));
#52934=CARTESIAN_POINT('Ctrl Pts',(19.805122901504,-0.532909080357985,127.135139757539));
#52935=CARTESIAN_POINT('Ctrl Pts',(19.9119297871484,-0.153404834080003,
127.159459066494));
#52936=CARTESIAN_POINT('Ctrl Pts',(19.8907835817646,0.345745192049258,127.189770694683));
#52937=CARTESIAN_POINT('Ctrl Pts',(19.6238862093633,0.880005756149412,127.226002377005));
#52938=CARTESIAN_POINT('Ctrl Pts',(19.1639432332974,1.25716124729007,127.262090500425));
#52939=CARTESIAN_POINT('Ctrl Pts',(18.5923414539904,1.4129249048356,127.298033459251));
#52940=CARTESIAN_POINT('Ctrl Pts',(18.009376013041,1.32200688726968,127.333829961582));
#52941=CARTESIAN_POINT('Ctrl Pts',(17.5164251968782,1.00223104074899,127.369478700124));
#52942=CARTESIAN_POINT('Ctrl Pts',(17.1984201622755,0.511061484236086,127.404978528688));
#52943=CARTESIAN_POINT('Ctrl Pts',(17.1091447607243,-0.0647150657709647,
127.440328369783));
#52944=CARTESIAN_POINT('Ctrl Pts',(17.2621761209424,-0.624337498948366,
127.47552726517));
#52945=CARTESIAN_POINT('Ctrl Pts',(17.6288480874875,-1.07071164630888,127.510574350276));
#52946=CARTESIAN_POINT('Ctrl Pts',(18.1436098481768,-1.32726550817446,127.545468867205));
#52947=CARTESIAN_POINT('Ctrl Pts',(18.7157402346546,-1.35108485996325,127.580210160365));
#52948=CARTESIAN_POINT('Ctrl Pts',(19.245344894428,-1.14007961976173,127.614797677075));
#52949=CARTESIAN_POINT('Ctrl Pts',(19.640802728471,-0.732985556833016,127.649230973288));
#52950=CARTESIAN_POINT('Ctrl Pts',(19.8346190767915,-0.202266924232661,
127.68350970104));
#52951=CARTESIAN_POINT('Ctrl Pts',(19.794941200486,0.358782068939732,127.717633632851));
#52952=CARTESIAN_POINT('Ctrl Pts',(19.53076983591,0.852439588636981,127.751602617564));
#52953=CARTESIAN_POINT('Ctrl Pts',(19.090026891229,1.19357867870462,127.785416661368));
#52954=CARTESIAN_POINT('Ctrl Pts',(18.5508679670964,1.32434237931937,127.819075778772));
#52955=CARTESIAN_POINT('Ctrl Pts',(18.0078302825239,1.22394906443107,127.852580278532));
#52956=CARTESIAN_POINT('Ctrl Pts',(17.5552573816975,0.911952688854262,127.885930186338));
#52957=CARTESIAN_POINT('Ctrl Pts',(17.2709072300368,0.444489100297998,127.919126443317));
#52958=CARTESIAN_POINT('Ctrl Pts',(17.2026017157444,-0.0958390632178888,
127.95216844486));
#52959=CARTESIAN_POINT('Ctrl Pts',(17.3602499056931,-0.614522317041156,
127.98505884808));
#52960=CARTESIAN_POINT('Ctrl Pts',(17.7142513339655,-1.02169725457206,128.017794748452));
#52961=CARTESIAN_POINT('Ctrl Pts',(18.2016487037711,-1.24768921999965,128.050383328832));
#52962=CARTESIAN_POINT('Ctrl Pts',(18.7359726277051,-1.25494106694358,128.082813363425));
#52963=CARTESIAN_POINT('Ctrl Pts',(19.2248728288001,-1.04408787605343,128.115109897118));
#52964=CARTESIAN_POINT('Ctrl Pts',(19.5831890659344,-0.65421290817496,128.147230907527));
#52965=CARTESIAN_POINT('Ctrl Pts',(19.7492083587371,-0.153536892969666,
128.179236143029));
#52966=CARTESIAN_POINT('Ctrl Pts',(19.7078812619029,0.281365767131694,128.205782412348));
#52967=CARTESIAN_POINT('Ctrl Pts',(19.5690632182825,0.594917565556771,128.226900693016));
#52968=CARTESIAN_POINT('Ctrl Pts',(19.4172180661828,0.803935885721005,128.242751399009));
#52969=CARTESIAN_POINT('Ctrl Pts',(19.2267655611754,0.976197794016201,128.258576146578));
#52970=CARTESIAN_POINT('Ctrl Pts',(19.0095330421784,1.10340832807125,128.274317652345));
#52971=CARTESIAN_POINT('Ctrl Pts',(18.7723693852942,1.18134487520901,128.289992329285));
#52972=CARTESIAN_POINT('Ctrl Pts',(18.6008172746989,1.19991945929139,128.300512808918));
#52973=CARTESIAN_POINT('Ctrl Pts',(18.5113472588518,1.200672491065,128.305809153521));
#52974=CARTESIAN_POINT('Ctrl Pts',(18.5130339424071,1.20056362969837,113.106041784737));
#52975=CARTESIAN_POINT('Ctrl Pts',(18.3796380772671,1.19944089238864,113.113938401934));
#52976=CARTESIAN_POINT('Ctrl Pts',(18.212995110346,1.1725142972848,113.124339511499));
#52977=CARTESIAN_POINT('Ctrl Pts',(17.9826591490378,1.08305259160243,113.139896234827));
#52978=CARTESIAN_POINT('Ctrl Pts',(17.803524665933,0.978054082781836,113.152884087551));
#52979=CARTESIAN_POINT('Ctrl Pts',(17.6157274597086,0.808171438104614,113.168486383471));
#52980=CARTESIAN_POINT('Ctrl Pts',(17.4669698936293,0.603184371142723,113.184027320395));
#52981=CARTESIAN_POINT('Ctrl Pts',(17.3317154043875,0.297605532561133,113.204606209043));
#52982=CARTESIAN_POINT('Ctrl Pts',(17.2920324724794,-0.124072418916653,
113.230343010212));
#52983=CARTESIAN_POINT('Ctrl Pts',(17.4520170046263,-0.605055189514055,
113.261099028093));
#52984=CARTESIAN_POINT('Ctrl Pts',(17.7934912025519,-0.975855665840217,
113.291676037855));
#52985=CARTESIAN_POINT('Ctrl Pts',(18.2552189298271,-1.17453711052494,113.322168039442));
#52986=CARTESIAN_POINT('Ctrl Pts',(18.7551481137232,-1.16725239972225,113.35250943295));
#52987=CARTESIAN_POINT('Ctrl Pts',(19.2070991942618,-0.957223190961011,
113.382741513919));
#52988=CARTESIAN_POINT('Ctrl Pts',(19.5322973485556,-0.582468238754353,
113.412845200661));
#52989=CARTESIAN_POINT('Ctrl Pts',(19.67562911591,-0.109392115546574,113.4428364914));
#52990=CARTESIAN_POINT('Ctrl Pts',(19.6134333463132,0.379063695104254,113.472709212202));
#52991=CARTESIAN_POINT('Ctrl Pts',(19.3581335051897,0.797942154392361,113.502471576948));
#52992=CARTESIAN_POINT('Ctrl Pts',(18.9554988299117,1.07499280853608,113.532123455326));
#52993=CARTESIAN_POINT('Ctrl Pts',(18.4765513487883,1.16311071322141,113.561669163361));
#52994=CARTESIAN_POINT('Ctrl Pts',(18.0050418257343,1.04832938392337,113.591111034677));
#52995=CARTESIAN_POINT('Ctrl Pts',(17.6228462935274,0.751992898776048,113.620452417211));
#52996=CARTESIAN_POINT('Ctrl Pts',(17.3957735356024,0.326816053916071,113.649696269244));
#52997=CARTESIAN_POINT('Ctrl Pts',(17.3622692515483,-0.152473939923612,
113.678845838443));
#52998=CARTESIAN_POINT('Ctrl Pts',(17.5269312773492,-0.602238859891372,
113.707904360153));
#52999=CARTESIAN_POINT('Ctrl Pts',(17.8599195062755,-0.944488824492963,
113.736875095012));
#53000=CARTESIAN_POINT('Ctrl Pts',(18.3023688496958,-1.12037212295033,113.765761510337));
#53001=CARTESIAN_POINT('Ctrl Pts',(18.7767195011618,-1.10026390590182,113.79456682245));
#53002=CARTESIAN_POINT('Ctrl Pts',(19.20036232763,-0.888732269322817,113.823294822786));
#53003=CARTESIAN_POINT('Ctrl Pts',(19.4998782438405,-0.523565915353651,
113.851948718461));
#53004=CARTESIAN_POINT('Ctrl Pts',(19.6238287528582,-0.069042122852276,
113.880532304547));
#53005=CARTESIAN_POINT('Ctrl Pts',(19.5514932889337,0.395397386636452,113.909049120675));
#53006=CARTESIAN_POINT('Ctrl Pts',(19.2963413863882,0.788895724742068,113.937502807462));
#53007=CARTESIAN_POINT('Ctrl Pts',(18.9035408070196,1.04336396475033,113.965897201427));
#53008=CARTESIAN_POINT('Ctrl Pts',(18.5189033647821,1.10305718516976,113.989512715973));
#53009=CARTESIAN_POINT('Ctrl Pts',(18.2170935930471,1.05362629581146,114.008379364579));
#53010=CARTESIAN_POINT('Ctrl Pts',(17.9322721627584,0.942922183815482,114.027229373729));
#53011=CARTESIAN_POINT('Ctrl Pts',(17.6324657495509,0.696846674343144,114.050761688215));
#53012=CARTESIAN_POINT('Ctrl Pts',(17.425055503591,0.280959502915125,114.078956524793));
#53013=CARTESIAN_POINT('Ctrl Pts',(17.4055967944488,-0.18267754383417,114.10711104627));
#53014=CARTESIAN_POINT('Ctrl Pts',(17.576990714563,-0.613287408704696,114.135229246085));
#53015=CARTESIAN_POINT('Ctrl Pts',(17.9089222268986,-0.935960644535223,
114.163315083866));
#53016=CARTESIAN_POINT('Ctrl Pts',(18.3432587594393,-1.09476592174151,114.191372484275));
#53017=CARTESIAN_POINT('Ctrl Pts',(18.8041739436501,-1.0623506219891,114.219405440553));
#53018=CARTESIAN_POINT('Ctrl Pts',(19.2113568643764,-0.844671996115093,
114.247417994911));
#53019=CARTESIAN_POINT('Ctrl Pts',(19.4939565663678,-0.479881778207605,
114.275414073228));
#53020=CARTESIAN_POINT('Ctrl Pts',(19.602870578309,-0.0316875262133413,
114.303397813562));
#53021=CARTESIAN_POINT('Ctrl Pts',(19.5192551399362,0.421780427746786,114.331373149327));
#53022=CARTESIAN_POINT('Ctrl Pts',(19.2577675592491,0.801476804257206,114.359344171195));
#53023=CARTESIAN_POINT('Ctrl Pts',(18.8640009332427,1.04126649915409,114.38731491532));
#53024=CARTESIAN_POINT('Ctrl Pts',(18.4065801432745,1.09932167624799,114.415289415434));
#53025=CARTESIAN_POINT('Ctrl Pts',(17.9652147903995,0.96545323156242,114.443271718198));
#53026=CARTESIAN_POINT('Ctrl Pts',(17.6168702254584,0.662865250839041,114.471265856675));
#53027=CARTESIAN_POINT('Ctrl Pts',(17.4223821071987,0.244151515100728,114.499275850459));
#53028=CARTESIAN_POINT('Ctrl Pts',(17.4158632785575,-0.217801781149448,
114.527305731795));
#53029=CARTESIAN_POINT('Ctrl Pts',(17.5987504131071,-0.642504769055747,
114.555359471907));
#53030=CARTESIAN_POINT('Ctrl Pts',(17.9394763579509,-0.955758872656263,
114.583441117837));
#53031=CARTESIAN_POINT('Ctrl Pts',(18.3789494100587,-1.10274388324017,114.611554520772));
#53032=CARTESIAN_POINT('Ctrl Pts',(18.7637182180745,-1.06484365534075,114.635012295721));
#53033=CARTESIAN_POINT('Ctrl Pts',(19.0424508871426,-0.942156957769831,
114.653798255564));
#53034=CARTESIAN_POINT('Ctrl Pts',(19.2899308634949,-0.764306884233674,
114.672598064115));
#53035=CARTESIAN_POINT('Ctrl Pts',(19.518838095101,-0.45130503992922,114.696125280008));
#53036=CARTESIAN_POINT('Ctrl Pts',(19.6162389073555,0.00455291390653928,
114.724405194968));
#53037=CARTESIAN_POINT('Ctrl Pts',(19.5188245336469,0.461234783976204,114.752736506486));
#53038=CARTESIAN_POINT('Ctrl Pts',(19.2428261053621,0.839051333697012,114.781122846759));
#53039=CARTESIAN_POINT('Ctrl Pts',(18.8357513946072,1.07166142270989,114.809568076315));
#53040=CARTESIAN_POINT('Ctrl Pts',(18.3681476504267,1.11783506684874,114.838075840133));
#53041=CARTESIAN_POINT('Ctrl Pts',(17.9214186539348,0.968636637637708,114.866649900509));
#53042=CARTESIAN_POINT('Ctrl Pts',(17.5737644205555,0.649236686622199,114.89529376417));
#53043=CARTESIAN_POINT('Ctrl Pts',(17.3863524615981,0.214541218418958,114.924011236812));
#53044=CARTESIAN_POINT('Ctrl Pts',(17.3922208704093,-0.207242974567453,
114.94960607363));
#53045=CARTESIAN_POINT('Ctrl Pts',(17.5227598690108,-0.548669402825176,
114.972054178389));
#53046=CARTESIAN_POINT('Ctrl Pts',(17.6641415820603,-0.736782609523537,
114.986512013638));
#53047=CARTESIAN_POINT('Ctrl Pts',(17.7781139017909,-0.842900640788488,
114.996163146039));
#53048=CARTESIAN_POINT('Ctrl Pts',(17.8386189394227,-0.89190163183184,115.000990777876));
#53049=CARTESIAN_POINT('Ctrl Pts',(17.9025047204443,-0.936525093453351,
115.005820975394));
#53050=CARTESIAN_POINT('Ctrl Pts',(18.0361866047991,-1.01671821007154,115.01548556243));
#53051=CARTESIAN_POINT('Ctrl Pts',(18.2569977876937,-1.10101938230418,115.030001946653));
#53052=CARTESIAN_POINT('Ctrl Pts',(18.5715829573991,-1.12761634912618,115.049395535593));
#53053=CARTESIAN_POINT('Ctrl Pts',(18.8819962126928,-1.06591766988281,115.068830862058));
#53054=CARTESIAN_POINT('Ctrl Pts',(19.1636267310059,-0.920442194840922,
115.088307050796));
#53055=CARTESIAN_POINT('Ctrl Pts',(19.3947687720096,-0.70212716075079,115.10782662024));
#53056=CARTESIAN_POINT('Ctrl Pts',(19.5563007110438,-0.427877912966269,
115.12738920833));
#53057=CARTESIAN_POINT('Ctrl Pts',(19.6635151319163,-0.0156350059498499,
115.153532473423));
#53058=CARTESIAN_POINT('Ctrl Pts',(19.5902298913756,0.417659782748033,115.179766516309));
#53059=CARTESIAN_POINT('Ctrl Pts',(19.3810030950217,0.729410953616704,115.202803646746));
#53060=CARTESIAN_POINT('Ctrl Pts',(19.2284838333689,0.878004295306615,115.215992109533));
#53061=CARTESIAN_POINT('Ctrl Pts',(19.0560409141327,1.00394927534599,115.229196429705));
#53062=CARTESIAN_POINT('Ctrl Pts',(18.8841989149175,1.08097496755606,115.240771440897));
#53063=CARTESIAN_POINT('Ctrl Pts',(18.7286133688239,1.1198781075186,115.250708898067));
#53064=CARTESIAN_POINT('Ctrl Pts',(18.6496731094318,1.13387301836795,115.255680590934));
#53065=CARTESIAN_POINT('Ctrl Pts',(18.5831584169845,1.14091923213438,115.259826351878));
#53066=CARTESIAN_POINT('Ctrl Pts',(18.529723859708,1.14368192373088,115.263144386349));
#53067=CARTESIAN_POINT('Ctrl Pts',(18.3127780164777,1.14782594742841,115.276605547771));
#53068=CARTESIAN_POINT('Ctrl Pts',(17.9179435637465,1.04727289839551,115.301097431437));
#53069=CARTESIAN_POINT('Ctrl Pts',(17.5797257591974,0.733975186272521,115.328828941497));
#53070=CARTESIAN_POINT('Ctrl Pts',(17.4287664162094,0.450044946400393,115.348699385795));
#53071=CARTESIAN_POINT('Ctrl Pts',(17.377297606354,0.297583470120713,115.358650468053));
#53072=CARTESIAN_POINT('Ctrl Pts',(17.3519609865365,0.171470130867239,115.366620991551));
#53073=CARTESIAN_POINT('Ctrl Pts',(17.3216820304358,-0.0841604199737449,
115.382574280005));
#53074=CARTESIAN_POINT('Ctrl Pts',(17.3965706674047,-0.509890259835511,
115.408571625553));
#53075=CARTESIAN_POINT('Ctrl Pts',(17.7713689197723,-0.980625185002351,
115.444744657348));
#53076=CARTESIAN_POINT('Ctrl Pts',(18.2819379865731,-1.19600603977953,115.478069008485));
#53077=CARTESIAN_POINT('Ctrl Pts',(18.7809183594824,-1.17713157755211,115.508498307924));
#53078=CARTESIAN_POINT('Ctrl Pts',(19.1943175486507,-0.99711316860877,115.535989892722));
#53079=CARTESIAN_POINT('Ctrl Pts',(19.5146598255097,-0.676954515020953,
115.563588212045));
#53080=CARTESIAN_POINT('Ctrl Pts',(19.6661763275141,-0.32989171948242,115.586676645489));
#53081=CARTESIAN_POINT('Ctrl Pts',(19.7052193472369,-0.0324134677453485,
115.605202352555));
#53082=CARTESIAN_POINT('Ctrl Pts',(19.692655682188,0.192603294558637,115.619123708899));
#53083=CARTESIAN_POINT('Ctrl Pts',(19.6473498976196,0.375330813104559,115.630748323528));
#53084=CARTESIAN_POINT('Ctrl Pts',(19.5910991581474,0.514700455878096,115.640061743476));
#53085=CARTESIAN_POINT('Ctrl Pts',(19.4876393156613,0.715280090270079,115.654045643533));
#53086=CARTESIAN_POINT('Ctrl Pts',(19.2627069666146,0.976847606906025,115.675074306831));
#53087=CARTESIAN_POINT('Ctrl Pts',(18.8544665534226,1.19281133282252,115.703225108284));
#53088=CARTESIAN_POINT('Ctrl Pts',(18.393677139478,1.24490620452606,115.731490065512));
#53089=CARTESIAN_POINT('Ctrl Pts',(18.056361634715,1.15465435594138,115.752775030142));
#53090=CARTESIAN_POINT('Ctrl Pts',(17.8544284561031,1.04536165171525,115.767001240127));
#53091=CARTESIAN_POINT('Ctrl Pts',(17.7270316965588,0.960272597146169,115.776494950284));
#53092=CARTESIAN_POINT('Ctrl Pts',(17.5260449274305,0.780780317627104,115.793134808535));
#53093=CARTESIAN_POINT('Ctrl Pts',(17.3905754983703,0.565699995287968,115.808633253397));
#53094=CARTESIAN_POINT('Ctrl Pts',(17.3245418584892,0.384620256252072,115.820582816104));
#53095=CARTESIAN_POINT('Ctrl Pts',(17.3071994994432,0.329457947086177,115.824169558128));
#53096=CARTESIAN_POINT('Ctrl Pts',(17.2924988163125,0.273477103726421,115.82775812202));
#53097=CARTESIAN_POINT('Ctrl Pts',(17.2804085467132,0.216862498090847,115.831348541136));
#53098=CARTESIAN_POINT('Ctrl Pts',(17.2709542538249,0.159706819127325,115.834940788347));
#53099=CARTESIAN_POINT('Ctrl Pts',(17.2619835886696,0.0829558301171504,
115.839732913633));
#53100=CARTESIAN_POINT('Ctrl Pts',(17.2518755906627,-0.129650604723723,
115.852921292731));
#53101=CARTESIAN_POINT('Ctrl Pts',(17.3177516317266,-0.478447503488098,
115.874558104341));
#53102=CARTESIAN_POINT('Ctrl Pts',(17.5704423404208,-0.880957856936553,
115.903526095127));
#53103=CARTESIAN_POINT('Ctrl Pts',(17.9542909508241,-1.16448384868491,115.932614015954));
#53104=CARTESIAN_POINT('Ctrl Pts',(18.417126376734,-1.28868540595138,115.961822241747));
#53105=CARTESIAN_POINT('Ctrl Pts',(18.8952608905801,-1.23500217847673,115.991151380529));
#53106=CARTESIAN_POINT('Ctrl Pts',(19.3225816532175,-1.00939401338301,116.020601817174));
#53107=CARTESIAN_POINT('Ctrl Pts',(19.5687260020783,-0.723472536993288,
116.043602420908));
#53108=CARTESIAN_POINT('Ctrl Pts',(19.6871366689245,-0.485101521697199,
116.060076548169));
#53109=CARTESIAN_POINT('Ctrl Pts',(19.7574170551575,-0.283927256490408,
116.073274006638));
#53110=CARTESIAN_POINT('Ctrl Pts',(19.8141138999387,0.0878915372728727,
116.096417002363));
#53111=CARTESIAN_POINT('Ctrl Pts',(19.6917792758234,0.626135643997373,116.129614388622));
#53112=CARTESIAN_POINT('Ctrl Pts',(19.2511975416191,1.12597766448505,116.169669102103));
#53113=CARTESIAN_POINT('Ctrl Pts',(18.622047619994,1.35545557509057,116.209941813808));
#53114=CARTESIAN_POINT('Ctrl Pts',(17.9560191179098,1.25556816985742,116.250432479901));
#53115=CARTESIAN_POINT('Ctrl Pts',(17.4948646415439,0.906628969258929,116.285204179477));
#53116=CARTESIAN_POINT('Ctrl Pts',(17.2559669240318,0.500241385841883,116.314159466878));
#53117=CARTESIAN_POINT('Ctrl Pts',(17.1297804940034,0.015714509245307,116.344909451306));
#53118=CARTESIAN_POINT('Ctrl Pts',(17.237512260039,-0.622576246018601,116.383518153498));
#53119=CARTESIAN_POINT('Ctrl Pts',(17.7578889155714,-1.2058175514389,116.430121193854));
#53120=CARTESIAN_POINT('Ctrl Pts',(18.5130575993667,-1.42399276281197,116.47699518141));
#53121=CARTESIAN_POINT('Ctrl Pts',(19.2728466936298,-1.20579250691246,116.524138179076));
#53122=CARTESIAN_POINT('Ctrl Pts',(19.8032798723121,-0.613305417176101,
116.571547805714));
#53123=CARTESIAN_POINT('Ctrl Pts',(19.915047421943,0.0433029384755907,116.611275982938));
#53124=CARTESIAN_POINT('Ctrl Pts',(19.7843821034173,0.54631812459105,116.643188946666));
#53125=CARTESIAN_POINT('Ctrl Pts',(19.5864236858098,0.883085765125937,116.667188711933));
#53126=CARTESIAN_POINT('Ctrl Pts',(19.3014292475285,1.15192941594928,116.691252738917));
#53127=CARTESIAN_POINT('Ctrl Pts',(18.8365401016989,1.3933575076252,116.723423700013));
#53128=CARTESIAN_POINT('Ctrl Pts',(18.160779938749,1.43204211152419,116.763796184507));
#53129=CARTESIAN_POINT('Ctrl Pts',(17.4456352832677,1.0373977222983,116.812493703962));
#53130=CARTESIAN_POINT('Ctrl Pts',(17.0481573163662,0.319374993023183,116.861437446236));
#53131=CARTESIAN_POINT('Ctrl Pts',(17.0938117001638,-0.504232219701305,
116.910623011974));
#53132=CARTESIAN_POINT('Ctrl Pts',(17.5729853188264,-1.18048171398732,116.960045601005));
#53133=CARTESIAN_POINT('Ctrl Pts',(18.3420871113973,-1.49965465644313,117.009700188431));
#53134=CARTESIAN_POINT('Ctrl Pts',(19.1668659216703,-1.36005147654203,117.05958143723));
#53135=CARTESIAN_POINT('Ctrl Pts',(19.7937047525059,-0.800566639011249,
117.109683748806));
#53136=CARTESIAN_POINT('Ctrl Pts',(20.0277875120747,0.0101379512286132,
117.160001253962));
#53137=CARTESIAN_POINT('Ctrl Pts',(19.7936847629856,0.824483128183414,117.210527832844));
#53138=CARTESIAN_POINT('Ctrl Pts',(19.1596616311847,1.39171327988103,117.261257100749));
#53139=CARTESIAN_POINT('Ctrl Pts',(18.3177908939756,1.53521530422674,117.312182432211));
#53140=CARTESIAN_POINT('Ctrl Pts',(17.5256836268175,1.20758890493412,117.363296973471));
#53141=CARTESIAN_POINT('Ctrl Pts',(17.0275455794861,0.506255522428237,117.414593637324));
#53142=CARTESIAN_POINT('Ctrl Pts',(16.9787373259702,-0.35553973474002,117.466065106827));
#53143=CARTESIAN_POINT('Ctrl Pts',(17.3973002169671,-1.11364573044326,117.517703870815));
#53144=CARTESIAN_POINT('Ctrl Pts',(18.1573683126717,-1.53416286108214,117.569502207969));
#53145=CARTESIAN_POINT('Ctrl Pts',(19.0272538362356,-1.48564336837537,117.621452211899));
#53146=CARTESIAN_POINT('Ctrl Pts',(19.7398503747652,-0.980418717802992,
117.673545759339));
#53147=CARTESIAN_POINT('Ctrl Pts',(20.0754586522521,-0.171264234164207,
117.725774634931));
#53148=CARTESIAN_POINT('Ctrl Pts',(19.9528984809521,0.549983689228882,117.769404367946));
#53149=CARTESIAN_POINT('Ctrl Pts',(19.6356116093765,1.02260359458153,117.804367384591));
#53150=CARTESIAN_POINT('Ctrl Pts',(19.2010969873656,1.39125738920211,117.839368176335));
#53151=CARTESIAN_POINT('Ctrl Pts',(18.4951761944866,1.59511231389331,117.883187939005));
#53152=CARTESIAN_POINT('Ctrl Pts',(17.6460434343933,1.35061332593586,117.935872096955));
#53153=CARTESIAN_POINT('Ctrl Pts',(17.0561860951254,0.69088986844999,117.988648088627));
#53154=CARTESIAN_POINT('Ctrl Pts',(16.9074971438262,-0.183028294006347,
118.041506623448));
#53155=CARTESIAN_POINT('Ctrl Pts',(17.2470534207198,-1.00316234166999,118.094438626915));
#53156=CARTESIAN_POINT('Ctrl Pts',(17.9717910595105,-1.51758676734159,118.14743475339));
#53157=CARTESIAN_POINT('Ctrl Pts',(18.8600432872684,-1.56756420344383,118.200485682854));
#53158=CARTESIAN_POINT('Ctrl Pts',(19.6394161118673,-1.13697309564611,118.253581949951));
#53159=CARTESIAN_POINT('Ctrl Pts',(20.0704659672594,-0.357096634960048,
118.306714148656));
#53160=CARTESIAN_POINT('Ctrl Pts',(20.0205702328933,0.532844361309807,118.359872635996));
#53161=CARTESIAN_POINT('Ctrl Pts',(19.504486863852,1.26036618044964,118.413048064539));
#53162=CARTESIAN_POINT('Ctrl Pts',(18.8180055338568,1.54444373835792,118.457366755587));
#53163=CARTESIAN_POINT('Ctrl Pts',(18.2407925832158,1.52713411330168,118.492820814792));
#53164=CARTESIAN_POINT('Ctrl Pts',(17.8284336500578,1.39613252265381,118.519409239185));
#53165=CARTESIAN_POINT('Ctrl Pts',(17.4685051427223,1.1554090378971,118.545995092116));
#53166=CARTESIAN_POINT('Ctrl Pts',(17.1893258099538,0.824898120829929,118.572576342922));
#53167=CARTESIAN_POINT('Ctrl Pts',(17.0125879486417,0.429862370286751,118.599152630315));
#53168=CARTESIAN_POINT('Ctrl Pts',(16.9521470208911,0.00161163153818327,
118.625721994921));
#53169=CARTESIAN_POINT('Ctrl Pts',(17.0125764443851,-0.42667872826605,118.652283949504));
#53170=CARTESIAN_POINT('Ctrl Pts',(17.1597806759054,-0.755367532112567,
118.674411046438));
#53171=CARTESIAN_POINT('Ctrl Pts',(17.3285403893103,-0.986405868394619,
118.692108255428));
#53172=CARTESIAN_POINT('Ctrl Pts',(17.5279443674188,-1.19111295414712,118.70980104078));
#53173=CARTESIAN_POINT('Ctrl Pts',(17.9466035736572,-1.47210445803857,118.740754696099));
#53174=CARTESIAN_POINT('Ctrl Pts',(18.6767611048209,-1.59634272918696,118.784942220793));
#53175=CARTESIAN_POINT('Ctrl Pts',(19.4977275477546,-1.25611034638129,118.837908121638));
#53176=CARTESIAN_POINT('Ctrl Pts',(19.9249220966151,-0.65331003248227,118.881989304197));
#53177=CARTESIAN_POINT('Ctrl Pts',(20.0218459481189,-0.160631817687348,
118.912811545655));
#53178=CARTESIAN_POINT('Ctrl Pts',(20.0180508629822,0.12358736647769,118.930414576253));
#53179=CARTESIAN_POINT('Ctrl Pts',(19.9743985426673,0.404842513306318,118.948009763686));
#53180=CARTESIAN_POINT('Ctrl Pts',(19.8465496236101,0.738729994358177,118.969990762044));
#53181=CARTESIAN_POINT('Ctrl Pts',(19.503237250369,1.19676088527163,119.00512939206));
#53182=CARTESIAN_POINT('Ctrl Pts',(18.8596729577346,1.55243356672786,119.048992892846));
#53183=CARTESIAN_POINT('Ctrl Pts',(17.9799831327098,1.50276019726124,119.101523819356));
#53184=CARTESIAN_POINT('Ctrl Pts',(17.263212307717,0.993819888846933,119.153941103703));
#53185=CARTESIAN_POINT('Ctrl Pts',(16.9839792247278,0.318663513392033,119.197519819886));
#53186=CARTESIAN_POINT('Ctrl Pts',(17.001110435418,-0.247819246073101,119.232317729451));
#53187=CARTESIAN_POINT('Ctrl Pts',(17.1079830203791,-0.584651791505382,
119.254037650762));
#53188=CARTESIAN_POINT('Ctrl Pts',(17.2300818521728,-0.797813714445423,
119.269226964678));
#53189=CARTESIAN_POINT('Ctrl Pts',(17.3117280880498,-0.9113604666153,119.277901992599));
#53190=CARTESIAN_POINT('Ctrl Pts',(17.4012920935501,-1.0188850040393,119.286574041755));
#53191=CARTESIAN_POINT('Ctrl Pts',(17.5267955079385,-1.14092085905138,119.297408117074));
#53192=CARTESIAN_POINT('Ctrl Pts',(17.7528270107813,-1.30615819007779,119.31473153276));
#53193=CARTESIAN_POINT('Ctrl Pts',(18.0742528290313,-1.44998548783811,119.336361940194));
#53194=CARTESIAN_POINT('Ctrl Pts',(18.4921163795425,-1.50892176698877,119.362281087325));
#53195=CARTESIAN_POINT('Ctrl Pts',(18.9093083092125,-1.44998013204778,119.388160932157));
#53196=CARTESIAN_POINT('Ctrl Pts',(19.2932994283458,-1.27810698095492,119.414001246931));
#53197=CARTESIAN_POINT('Ctrl Pts',(19.6141891347275,-1.00707517579684,119.43980038992));
#53198=CARTESIAN_POINT('Ctrl Pts',(19.8471250805189,-0.658373354783552,
119.465558201273));
#53199=CARTESIAN_POINT('Ctrl Pts',(19.9742228972475,-0.259467245505255,
119.491272617658));
#53200=CARTESIAN_POINT('Ctrl Pts',(19.9858753700794,0.158301952850977,119.516944194725));
#53201=CARTESIAN_POINT('Ctrl Pts',(19.8990241695029,0.494979507521757,119.538299135457));
#53202=CARTESIAN_POINT('Ctrl Pts',(19.7757742210683,0.741612695103491,119.555361011189));
#53203=CARTESIAN_POINT('Ctrl Pts',(19.58069155028,1.0254111001558,119.576668756615));
#53204=CARTESIAN_POINT('Ctrl Pts',(19.2012637945808,1.33666302774039,119.606445571674));
#53205=CARTESIAN_POINT('Ctrl Pts',(18.59413116038,1.50218145374168,119.644622711453));
#53206=CARTESIAN_POINT('Ctrl Pts',(17.9741889539315,1.40557451760412,119.682689594233));
#53207=CARTESIAN_POINT('Ctrl Pts',(17.4493194520646,1.0651884348338,119.720643422888));
#53208=CARTESIAN_POINT('Ctrl Pts',(17.1103034219914,0.541698384717174,119.758481493696));
#53209=CARTESIAN_POINT('Ctrl Pts',(17.0149844688412,-0.0726480667363822,
119.796201073521));
#53210=CARTESIAN_POINT('Ctrl Pts',(17.1783582983629,-0.670477000498041,
119.833799757369));
#53211=CARTESIAN_POINT('Ctrl Pts',(17.5050878418038,-1.06819893534445,119.865028891154));
#53212=CARTESIAN_POINT('Ctrl Pts',(17.8458525729069,-1.28516330407485,119.889949495029));
#53213=CARTESIAN_POINT('Ctrl Pts',(18.2235157805367,-1.42666993037966,119.914827505529));
#53214=CARTESIAN_POINT('Ctrl Pts',(18.7343004495072,-1.44806142418328,119.945845031736));
#53215=CARTESIAN_POINT('Ctrl Pts',(19.3022641117884,-1.22179759041786,119.98293553694));
#53216=CARTESIAN_POINT('Ctrl Pts',(19.7267504298182,-0.784916367409439,
120.019893470825));
#53217=CARTESIAN_POINT('Ctrl Pts',(19.9350082684945,-0.214809342616007,
120.056716728399));
#53218=CARTESIAN_POINT('Ctrl Pts',(19.8923964259192,0.388373946010418,120.093403372529));
#53219=CARTESIAN_POINT('Ctrl Pts',(19.6082151774614,0.919535325612133,120.129951516022));
#53220=CARTESIAN_POINT('Ctrl Pts',(19.1336807132418,1.28688374926404,120.166359391381));
#53221=CARTESIAN_POINT('Ctrl Pts',(18.5527927781208,1.42780271129681,120.202625307385));
#53222=CARTESIAN_POINT('Ctrl Pts',(17.9672849430062,1.31962837356636,120.238747690412));
#53223=CARTESIAN_POINT('Ctrl Pts',(17.5604664448896,1.03912928877408,120.268728808256));
#53224=CARTESIAN_POINT('Ctrl Pts',(17.3255478081665,0.730808963275233,120.29264048669));
#53225=CARTESIAN_POINT('Ctrl Pts',(17.1598505083254,0.381251616548514,120.316503198891));
#53226=CARTESIAN_POINT('Ctrl Pts',(17.0983099735108,-0.104991940913315,
120.34623918748));
#53227=CARTESIAN_POINT('Ctrl Pts',(17.2685940660949,-0.665398892142992,
120.381773515751));
#53228=CARTESIAN_POINT('Ctrl Pts',(17.6512792739107,-1.10550385025771,120.41715783718));
#53229=CARTESIAN_POINT('Ctrl Pts',(18.1781005502915,-1.34987930889349,120.452391196463));
#53230=CARTESIAN_POINT('Ctrl Pts',(18.7562794468606,-1.35772126535799,120.487472684011));
#53231=CARTESIAN_POINT('Ctrl Pts',(19.2849262650991,-1.12972301595998,120.522401531095));
#53232=CARTESIAN_POINT('Ctrl Pts',(19.6726290138236,-0.707545247949752,
120.557177051768));
#53233=CARTESIAN_POINT('Ctrl Pts',(19.8532773460226,-0.16623998601176,120.59179867559));
#53234=CARTESIAN_POINT('Ctrl Pts',(19.797325294628,0.399107448838622,120.626265930169));
#53235=CARTESIAN_POINT('Ctrl Pts',(19.516604963237,0.890078600748408,120.66057845095));
#53236=CARTESIAN_POINT('Ctrl Pts',(19.0618960487862,1.22206271419135,120.694735976808));
#53237=CARTESIAN_POINT('Ctrl Pts',(18.5137492588806,1.33883473443734,120.728738352884));
#53238=CARTESIAN_POINT('Ctrl Pts',(17.968216849916,1.22206908408025,120.762585529099));
#53239=CARTESIAN_POINT('Ctrl Pts',(17.5200207911922,0.894176786428842,120.796277560609));
#53240=CARTESIAN_POINT('Ctrl Pts',(17.2461072346647,0.414037560067,120.829814607784));
#53241=CARTESIAN_POINT('Ctrl Pts',(17.1924430147546,-0.133565974408157,
120.863196936287));
#53242=CARTESIAN_POINT('Ctrl Pts',(17.366317551762,-0.652915584466722,120.896424916945));
#53243=CARTESIAN_POINT('Ctrl Pts',(17.7354356853631,-1.05408452248002,120.929499025204));
#53244=CARTESIAN_POINT('Ctrl Pts',(18.2338946800392,-1.26850207170023,120.962419840475));
#53245=CARTESIAN_POINT('Ctrl Pts',(18.7739421572114,-1.26066264713202,120.995188046564));
#53246=CARTESIAN_POINT('Ctrl Pts',(19.261417515124,-1.03398313097046,121.02780443056));
#53247=CARTESIAN_POINT('Ctrl Pts',(19.6121606614966,-0.629846282234725,
121.060269883735));
#53248=CARTESIAN_POINT('Ctrl Pts',(19.7665300506899,-0.120063655066437,
121.092585397355));
#53249=CARTESIAN_POINT('Ctrl Pts',(19.6995288695014,0.405875592196416,121.124752068354));
#53250=CARTESIAN_POINT('Ctrl Pts',(19.4248220741339,0.856499430305402,121.156771086707));
#53251=CARTESIAN_POINT('Ctrl Pts',(18.9920077149049,1.15425452722384,121.188643758256));
#53252=CARTESIAN_POINT('Ctrl Pts',(18.477675702841,1.24882569485176,121.22037145959));
#53253=CARTESIAN_POINT('Ctrl Pts',(17.9718722366947,1.12564015935962,121.25195571884));
#53254=CARTESIAN_POINT('Ctrl Pts',(17.5623444137067,0.808028409142753,121.283398060944));
#53255=CARTESIAN_POINT('Ctrl Pts',(17.3193477993976,0.35291029010133,121.314700295335));
#53256=CARTESIAN_POINT('Ctrl Pts',(17.2835915860888,-0.159531772662667,
121.345863968405));
#53257=CARTESIAN_POINT('Ctrl Pts',(17.4155057372333,-0.519645729494795,
121.369134581872));
#53258=CARTESIAN_POINT('Ctrl Pts',(17.5594893836391,-0.723752038926638,
121.384605922907));
#53259=CARTESIAN_POINT('Ctrl Pts',(17.668999693357,-0.848911852993158,121.39490936142));
#53260=CARTESIAN_POINT('Ctrl Pts',(17.8931906723513,-1.03579597290683,121.412910620692));
#53261=CARTESIAN_POINT('Ctrl Pts',(18.2857522897131,-1.19187578457209,121.438544180847));
#53262=CARTESIAN_POINT('Ctrl Pts',(18.7902002679314,-1.17038056405782,121.469173977415));
#53263=CARTESIAN_POINT('Ctrl Pts',(19.2399332524197,-0.945736597983726,
121.499675716141));
#53264=CARTESIAN_POINT('Ctrl Pts',(19.5574022269321,-0.558563760582848,
121.530051638976));
#53265=CARTESIAN_POINT('Ctrl Pts',(19.6884983642052,-0.0774725349686712,
121.560304199798));
#53266=CARTESIAN_POINT('Ctrl Pts',(19.6119798866289,0.413247003691924,121.590435869102));
#53267=CARTESIAN_POINT('Ctrl Pts',(19.3427638331946,0.828274604425165,121.620449235126));
#53268=CARTESIAN_POINT('Ctrl Pts',(18.9291167211882,1.09611529685852,121.650346948405));
#53269=CARTESIAN_POINT('Ctrl Pts',(18.4439871351089,1.17136126566376,121.680131747619));
#53270=CARTESIAN_POINT('Ctrl Pts',(17.9721852197242,1.04237957129896,121.709806443118));
#53271=CARTESIAN_POINT('Ctrl Pts',(17.5955767614254,0.733067066500168,121.739373920544));
#53272=CARTESIAN_POINT('Ctrl Pts',(17.3789145552552,0.298448464042141,121.768837139486));
#53273=CARTESIAN_POINT('Ctrl Pts',(17.3587311152265,-0.185091286281474,
121.798199127953));
#53274=CARTESIAN_POINT('Ctrl Pts',(17.5372040232563,-0.633201450870468,
121.827462989564));
#53275=CARTESIAN_POINT('Ctrl Pts',(17.882013145033,-0.968245111307221,121.856631880607));
#53276=CARTESIAN_POINT('Ctrl Pts',(18.3321736501231,-1.13271867310312,121.885709046681));
#53277=CARTESIAN_POINT('Ctrl Pts',(18.8087973084627,-1.09908843399563,121.914697746937));
#53278=CARTESIAN_POINT('Ctrl Pts',(19.2288806489506,-0.874386164600571,
121.943601393848));
#53279=CARTESIAN_POINT('Ctrl Pts',(19.5197284804084,-0.498764010730529,
121.972423284531));
#53280=CARTESIAN_POINT('Ctrl Pts',(19.631488858918,-0.0383710896155189,
122.001167096572));
#53281=CARTESIAN_POINT('Ctrl Pts',(19.5456822019558,0.42631741060901,122.029836034946));
#53282=CARTESIAN_POINT('Ctrl Pts',(19.2782376706958,0.814460654457481,122.058433950357));
#53283=CARTESIAN_POINT('Ctrl Pts',(18.8765333476415,1.05894522909086,122.086964325726));
#53284=CARTESIAN_POINT('Ctrl Pts',(18.411053545632,1.11790498477854,122.115430833469));
#53285=CARTESIAN_POINT('Ctrl Pts',(17.9630346452634,0.981894731140524,122.143837222082));
#53286=CARTESIAN_POINT('Ctrl Pts',(17.6103416604701,0.675370135250457,122.172187197682));
#53287=CARTESIAN_POINT('Ctrl Pts',(17.4139663666992,0.252314060233207,122.200484547726));
#53288=CARTESIAN_POINT('Ctrl Pts',(17.4075180258619,-0.213249102834493,
122.228733136097));
#53289=CARTESIAN_POINT('Ctrl Pts',(17.5914890882151,-0.640162939071301,
122.256936743679));
#53290=CARTESIAN_POINT('Ctrl Pts',(17.9332829313857,-0.954248513992901,
122.285099331242));
#53291=CARTESIAN_POINT('Ctrl Pts',(18.3729700883329,-1.10114856672374,122.313224762676));
#53292=CARTESIAN_POINT('Ctrl Pts',(18.8337656364914,-1.0557099732899,122.341316973501));
#53293=CARTESIAN_POINT('Ctrl Pts',(19.2353976864752,-0.826269100476284,
122.369379975043));
#53294=CARTESIAN_POINT('Ctrl Pts',(19.5080473835103,-0.453137156095097,
122.397417661645));
#53295=CARTESIAN_POINT('Ctrl Pts',(19.6044460345045,-0.00152756021506351,
122.425434134331));
#53296=CARTESIAN_POINT('Ctrl Pts',(19.5080490631313,0.449785662790224,122.453433287289));
#53297=CARTESIAN_POINT('Ctrl Pts',(19.2358501405623,0.822201779793111,122.481419310144));
#53298=CARTESIAN_POINT('Ctrl Pts',(18.8354297261873,1.05088321709065,122.509395984532));
#53299=CARTESIAN_POINT('Ctrl Pts',(18.3766008448291,1.09606510988091,122.537367609601));
#53300=CARTESIAN_POINT('Ctrl Pts',(17.9393577912152,0.949926431334445,122.565338058587));
#53301=CARTESIAN_POINT('Ctrl Pts',(17.5998948604504,0.637888425774447,122.593311446551));
#53302=CARTESIAN_POINT('Ctrl Pts',(17.4174396576394,0.214366012794586,122.621291806824));
#53303=CARTESIAN_POINT('Ctrl Pts',(17.4231623787231,-0.1957658757123,122.646172972246));
#53304=CARTESIAN_POINT('Ctrl Pts',(17.5499930456385,-0.526830239172015,
122.667953798238));
#53305=CARTESIAN_POINT('Ctrl Pts',(17.7932141540085,-0.851346049715726,
122.692856554516));
#53306=CARTESIAN_POINT('Ctrl Pts',(18.2501761462134,-1.10418600330839,122.72400778286));
#53307=CARTESIAN_POINT('Ctrl Pts',(18.8769616675777,-1.06908370626514,122.761434859433));
#53308=CARTESIAN_POINT('Ctrl Pts',(19.3896239215073,-0.70545262307287,122.798917126171));
#53309=CARTESIAN_POINT('Ctrl Pts',(19.6307566921668,-0.12384402484574,122.836463844081));
#53310=CARTESIAN_POINT('Ctrl Pts',(19.5252616357798,0.498282873588724,122.874084352006));
#53311=CARTESIAN_POINT('Ctrl Pts',(19.1742691062997,0.891055442512747,122.905503881039));
#53312=CARTESIAN_POINT('Ctrl Pts',(18.7996171429706,1.05785424932804,122.930685519148));
#53313=CARTESIAN_POINT('Ctrl Pts',(18.5061980272808,1.09969585165476,122.948895536135));
#53314=CARTESIAN_POINT('Ctrl Pts',(18.2235705570867,1.06394203818006,122.966427195679));
#53315=CARTESIAN_POINT('Ctrl Pts',(17.8835419458233,0.931126744519063,122.988895417304));
#53316=CARTESIAN_POINT('Ctrl Pts',(17.540325572912,0.612977032071075,123.017034360395));
#53317=CARTESIAN_POINT('Ctrl Pts',(17.3907978799752,0.168200478695434,123.045250354356));
#53318=CARTESIAN_POINT('Ctrl Pts',(17.4097069157206,-0.198885785314081,
123.067872011256));
#53319=CARTESIAN_POINT('Ctrl Pts',(17.5175585534041,-0.550747043662346,
123.090527691658));
#53320=CARTESIAN_POINT('Ctrl Pts',(17.811694265428,-0.920088885831626,123.118912113209));
#53321=CARTESIAN_POINT('Ctrl Pts',(18.2916876292038,-1.12241961155101,123.150236055638));
#53322=CARTESIAN_POINT('Ctrl Pts',(18.7599954609617,-1.10466062303536,123.178796710933));
#53323=CARTESIAN_POINT('Ctrl Pts',(19.1475491472277,-0.935850007334233,
123.204568881909));
#53324=CARTESIAN_POINT('Ctrl Pts',(19.4474303836746,-0.636042641389887,
123.230410947105));
#53325=CARTESIAN_POINT('Ctrl Pts',(19.6175361159645,-0.246469240807822,
123.256325134572));
#53326=CARTESIAN_POINT('Ctrl Pts',(19.6336055704725,0.179639336476098,123.282313928802));
#53327=CARTESIAN_POINT('Ctrl Pts',(19.4924664396755,0.583268923924529,123.308379216194));
#53328=CARTESIAN_POINT('Ctrl Pts',(19.2594187855067,0.854320734565662,123.330166333392));
#53329=CARTESIAN_POINT('Ctrl Pts',(19.0225876601379,1.00901198977016,123.347636263176));
#53330=CARTESIAN_POINT('Ctrl Pts',(18.7174728526583,1.13601015551723,123.368049966962));
#53331=CARTESIAN_POINT('Ctrl Pts',(18.2558875246191,1.15934765713978,123.395834765122));
#53332=CARTESIAN_POINT('Ctrl Pts',(17.8157869453812,0.947553194065168,123.425209130312));
#53333=CARTESIAN_POINT('Ctrl Pts',(17.5553879829031,0.666356292508678,123.448787444948));
#53334=CARTESIAN_POINT('Ctrl Pts',(17.4178065523958,0.413637397213519,123.466510938034));
#53335=CARTESIAN_POINT('Ctrl Pts',(17.3221820932953,0.0406364433144716,
123.490196526986));
#53336=CARTESIAN_POINT('Ctrl Pts',(17.3772635808422,-0.400356807765698,
123.516935032653));
#53337=CARTESIAN_POINT('Ctrl Pts',(17.637978375011,-0.814840216527707,123.546767553284));
#53338=CARTESIAN_POINT('Ctrl Pts',(18.0081494220083,-1.08849077489295,123.574836116967));
#53339=CARTESIAN_POINT('Ctrl Pts',(18.4775112774984,-1.20283620753728,123.604140665495));
#53340=CARTESIAN_POINT('Ctrl Pts',(18.9728689947087,-1.11170713766108,123.634699102384));
#53341=CARTESIAN_POINT('Ctrl Pts',(19.3548250710418,-0.848888554637065,
123.662829393191));
#53342=CARTESIAN_POINT('Ctrl Pts',(19.543864380145,-0.572027787550067,123.683364369092));
#53343=CARTESIAN_POINT('Ctrl Pts',(19.6489401612735,-0.315921957158224,
123.700513727019));
#53344=CARTESIAN_POINT('Ctrl Pts',(19.7008713985811,-0.0552588957866882,
123.716838067645));
#53345=CARTESIAN_POINT('Ctrl Pts',(19.6726256840306,0.280232965878121,123.737517870146));
#53346=CARTESIAN_POINT('Ctrl Pts',(19.5522795280404,0.595728848538907,123.7582584388));
#53347=CARTESIAN_POINT('Ctrl Pts',(19.3486831682667,0.866369771861213,123.779059848981));
#53348=CARTESIAN_POINT('Ctrl Pts',(19.0773416884718,1.07066171040279,123.799923006162));
#53349=CARTESIAN_POINT('Ctrl Pts',(18.7855851467281,1.18212492987368,123.819104474902));
#53350=CARTESIAN_POINT('Ctrl Pts',(18.5041991856914,1.21572785039616,123.836587848181));
#53351=CARTESIAN_POINT('Ctrl Pts',(18.1646934338967,1.18499174658801,123.857615096215));
#53352=CARTESIAN_POINT('Ctrl Pts',(17.7653832410379,1.01332364019048,123.883988407248));
#53353=CARTESIAN_POINT('Ctrl Pts',(17.4105724745461,0.627640142468378,123.91578041595));
#53354=CARTESIAN_POINT('Ctrl Pts',(17.2434553757277,0.12848973275699,123.947718069321));
#53355=CARTESIAN_POINT('Ctrl Pts',(17.2950338468023,-0.397842330961294,
123.979802636553));
#53356=CARTESIAN_POINT('Ctrl Pts',(17.5582954032972,-0.859299372811185,
124.012035412185));
#53357=CARTESIAN_POINT('Ctrl Pts',(17.9890647139176,-1.17444949802056,124.044417524025));
#53358=CARTESIAN_POINT('Ctrl Pts',(18.5134073925165,-1.28668013802211,124.076950033579));
#53359=CARTESIAN_POINT('Ctrl Pts',(19.040299183268,-1.17444205619667,124.109633881169));
#53360=CARTESIAN_POINT('Ctrl Pts',(19.477419740777,-0.855306063337771,124.142469914755));
#53361=CARTESIAN_POINT('Ctrl Pts',(19.747318196117,-0.383277623495378,124.175458873959));
#53362=CARTESIAN_POINT('Ctrl Pts',(19.8011287001543,0.160339974187855,124.20860139743));
#53363=CARTESIAN_POINT('Ctrl Pts',(19.6274041961022,0.680932515573491,124.241898017848));
#53364=CARTESIAN_POINT('Ctrl Pts',(19.2544751124545,1.08703964110571,124.275349164061));
#53365=CARTESIAN_POINT('Ctrl Pts',(18.7458556784281,1.30641671855503,124.308955159866));
#53366=CARTESIAN_POINT('Ctrl Pts',(18.189437375636,1.29888227807384,124.342716224406));
#53367=CARTESIAN_POINT('Ctrl Pts',(17.6823055406022,1.06366182687317,124.37663247134));
#53368=CARTESIAN_POINT('Ctrl Pts',(17.3138010055331,0.639890347952039,124.410703908926));
#53369=CARTESIAN_POINT('Ctrl Pts',(17.1497814706464,0.100118900233251,124.444930440075));
#53370=CARTESIAN_POINT('Ctrl Pts',(17.2208555754922,-0.462100903720547,
124.479311862771));
#53371=CARTESIAN_POINT('Ctrl Pts',(17.5166919909782,-0.948431814978525,
124.513847869957));
#53372=CARTESIAN_POINT('Ctrl Pts',(17.9874589398796,-1.27295449876341,124.548538049416));
#53373=CARTESIAN_POINT('Ctrl Pts',(18.5522074356213,-1.37734955352004,124.583381884254));
#53374=CARTESIAN_POINT('Ctrl Pts',(19.1127907478127,-1.24137444588285,124.61837875334));
#53375=CARTESIAN_POINT('Ctrl Pts',(19.570927231329,-0.886752979347359,124.653527932135));
#53376=CARTESIAN_POINT('Ctrl Pts',(19.8454390955441,-0.373734529845406,
124.6888285926));
#53377=CARTESIAN_POINT('Ctrl Pts',(19.8866416789606,0.209138420975833,124.724279803654));
#53378=CARTESIAN_POINT('Ctrl Pts',(19.6853313203903,0.760317927546962,124.759880531932));
#53379=CARTESIAN_POINT('Ctrl Pts',(19.274746020493,1.18295333165501,124.795629642769));
#53380=CARTESIAN_POINT('Ctrl Pts',(18.7250932562895,1.40192119416919,124.831525901343));
#53381=CARTESIAN_POINT('Ctrl Pts',(18.1315421099629,1.37718539583083,124.8675679727));
#53382=CARTESIAN_POINT('Ctrl Pts',(17.5977335091393,1.11110962070016,124.90375442263));
#53383=CARTESIAN_POINT('Ctrl Pts',(17.2176675190692,0.648387246466477,124.940083718826));
#53384=CARTESIAN_POINT('Ctrl Pts',(17.0591358261671,0.0685399773490914,
124.976554232237));
#53385=CARTESIAN_POINT('Ctrl Pts',(17.1516223906728,-0.527757683984189,
125.013164238674));
#53386=CARTESIAN_POINT('Ctrl Pts',(17.4808337728012,-1.03617512245347,125.049911918955));
#53387=CARTESIAN_POINT('Ctrl Pts',(17.9908722758733,-1.36699968915259,125.086795359982));
#53388=CARTESIAN_POINT('Ctrl Pts',(18.5937293060452,-1.46098376939424,125.123812556508));
#53389=CARTESIAN_POINT('Ctrl Pts',(19.1844869028144,-1.29996231384015,125.160961412641));
#53390=CARTESIAN_POINT('Ctrl Pts',(19.6595994719402,-0.910336227375098,
125.198239744056));
#53391=CARTESIAN_POINT('Ctrl Pts',(19.935066233012,-0.358757208946706,125.235645278193));
#53392=CARTESIAN_POINT('Ctrl Pts',(19.9613007891063,0.259283810673803,125.273175655495));
#53393=CARTESIAN_POINT('Ctrl Pts',(19.7320620910867,0.836009611459873,125.310828431745));
#53394=CARTESIAN_POINT('Ctrl Pts',(19.2858368185977,1.27017821405643,125.348601079706));
#53395=CARTESIAN_POINT('Ctrl Pts',(18.6993793782574,1.48488146702807,125.386490991953));
#53396=CARTESIAN_POINT('Ctrl Pts',(18.0744929819311,1.44118677993217,125.424495481034));
#53397=CARTESIAN_POINT('Ctrl Pts',(17.5203309456295,1.14519868643357,125.462611781001));
#53398=CARTESIAN_POINT('Ctrl Pts',(17.1342996581372,0.647258515357208,125.500837050006));
#53399=CARTESIAN_POINT('Ctrl Pts',(16.9849097134977,0.0333749870028357,
125.539168372337));
#53400=CARTESIAN_POINT('Ctrl Pts',(17.0995994614457,-0.589654791868995,
125.577602761599));
#53401=CARTESIAN_POINT('Ctrl Pts',(17.4596986530298,-1.11285616969424,125.616137161058));
#53402=CARTESIAN_POINT('Ctrl Pts',(18.0034565556922,-1.44417105987669,125.654768445165));
#53403=CARTESIAN_POINT('Ctrl Pts',(18.6366460765495,-1.52468380343448,125.693493422678));
#53404=CARTESIAN_POINT('Ctrl Pts',(19.2489206681697,-1.33911367710705,125.732308838738));
#53405=CARTESIAN_POINT('Ctrl Pts',(19.7330798824833,-0.918702162929582,
125.771211378595));
#53406=CARTESIAN_POINT('Ctrl Pts',(20.003873712581,-0.335951044009737,125.810197667968));
#53407=CARTESIAN_POINT('Ctrl Pts',(20.0130409900718,0.307902407747933,125.849264274755));
#53408=CARTESIAN_POINT('Ctrl Pts',(19.7579238844887,0.900506033918292,125.888407712264));
#53409=CARTESIAN_POINT('Ctrl Pts',(19.282118126251,1.3380365586316,125.927624441706));
#53410=CARTESIAN_POINT('Ctrl Pts',(18.6680121178992,1.54342523826848,125.966910876023));
#53411=CARTESIAN_POINT('Ctrl Pts',(18.0224934653108,1.479959447458,126.006263380594));
#53412=CARTESIAN_POINT('Ctrl Pts',(17.4583073090084,1.1578549526847,126.045678274836));
#53413=CARTESIAN_POINT('Ctrl Pts',(17.0743240513896,0.632620214794982,126.08515183572));
#53414=CARTESIAN_POINT('Ctrl Pts',(16.9381771242321,-0.00452739822763612,
126.124680300394));
#53415=CARTESIAN_POINT('Ctrl Pts',(17.0743261534331,-0.64253589142097,126.164259870224));
#53416=CARTESIAN_POINT('Ctrl Pts',(17.4596567592957,-1.16991519259679,126.203886711707));
#53417=CARTESIAN_POINT('Ctrl Pts',(18.0274097244559,-1.49426106398949,126.243556958088));
#53418=CARTESIAN_POINT('Ctrl Pts',(18.6787710739259,-1.55848016466035,126.283266712911));
#53419=CARTESIAN_POINT('Ctrl Pts',(19.3001068465522,-1.35086105258382,126.323012052985));
#53420=CARTESIAN_POINT('Ctrl Pts',(19.7828302049358,-0.907210804819137,
126.36278903232));
#53421=CARTESIAN_POINT('Ctrl Pts',(20.0424196828473,-0.304667060645809,
126.402593683509));
#53422=CARTESIAN_POINT('Ctrl Pts',(20.0332506859797,0.351742851216847,126.442422019401));
#53423=CARTESIAN_POINT('Ctrl Pts',(19.7566314877895,0.947449108115339,126.4822700359));
#53424=CARTESIAN_POINT('Ctrl Pts',(19.2606259379933,1.37838027922372,126.522133716601));
#53425=CARTESIAN_POINT('Ctrl Pts',(18.6316832039008,1.56918550021926,126.562009034018));
#53426=CARTESIAN_POINT('Ctrl Pts',(17.9795384681277,1.4864383553722,126.601891956083));
#53427=CARTESIAN_POINT('Ctrl Pts',(17.4180219901316,1.14450714080288,126.64177843909));
#53428=CARTESIAN_POINT('Ctrl Pts',(17.0451507093673,0.60305178731209,126.681664446109));
#53429=CARTESIAN_POINT('Ctrl Pts',(16.9259721145279,-0.0434035665844907,
126.721545922569));
#53430=CARTESIAN_POINT('Ctrl Pts',(17.0812073691357,-0.682018342919702,
126.761418852013));
#53431=CARTESIAN_POINT('Ctrl Pts',(17.48361106064,-1.20135795626228,126.801279160675));
#53432=CARTESIAN_POINT('Ctrl Pts',(18.0628189959856,-1.51091507882325,126.841122901587));
#53433=CARTESIAN_POINT('Ctrl Pts',(18.7175753989508,-1.55685481943617,126.880945914479));
#53434=CARTESIAN_POINT('Ctrl Pts',(19.3336690282003,-1.33151582505569,126.920744475439));
#53435=CARTESIAN_POINT('Ctrl Pts',(19.7252122247228,-0.950635904975706,
126.95388579676));
#53436=CARTESIAN_POINT('Ctrl Pts',(19.9246599065469,-0.570211393078723,
126.980382990007));
#53437=CARTESIAN_POINT('Ctrl Pts',(20.0410084568928,-0.156926761860616,
127.00686812107));
#53438=CARTESIAN_POINT('Ctrl Pts',(20.0180960753438,0.387885002702108,127.03995229568));
#53439=CARTESIAN_POINT('Ctrl Pts',(19.7261197888881,0.972790423017701,127.079612454345));
#53440=CARTESIAN_POINT('Ctrl Pts',(19.2213375973188,1.38696677386596,127.119228496333));
#53441=CARTESIAN_POINT('Ctrl Pts',(18.5921407553839,1.55862427081998,127.158796244357));
#53442=CARTESIAN_POINT('Ctrl Pts',(17.9485754461998,1.45844625626644,127.19831204202));
#53443=CARTESIAN_POINT('Ctrl Pts',(17.4028219204161,1.10463821938839,127.237772008334));
#53444=CARTESIAN_POINT('Ctrl Pts',(17.0497229688341,0.55959920647719,127.277172437709));
#53445=CARTESIAN_POINT('Ctrl Pts',(16.9502018159956,-0.0810954772450534,
127.316509591208));
#53446=CARTESIAN_POINT('Ctrl Pts',(17.1207658108625,-0.705493479039353,
127.355779812835));
#53447=CARTESIAN_POINT('Ctrl Pts',(17.5307517205212,-1.20486476242342,127.39497947225));
#53448=CARTESIAN_POINT('Ctrl Pts',(18.107855145551,-1.49267495326757,127.434104996807));
#53449=CARTESIAN_POINT('Ctrl Pts',(18.7509009483514,-1.51960879688507,127.473152857691));
#53450=CARTESIAN_POINT('Ctrl Pts',(19.3476186900617,-1.28203401909253,127.512119582085));
#53451=CARTESIAN_POINT('Ctrl Pts',(19.7942807409555,-0.822448911396595,
127.551001750383));
#53452=CARTESIAN_POINT('Ctrl Pts',(20.013768325998,-0.221869682102491,127.589796006502));
#53453=CARTESIAN_POINT('Ctrl Pts',(19.9689094941412,0.414477136693096,127.628499035169));
#53454=CARTESIAN_POINT('Ctrl Pts',(19.668779827001,0.975626090422456,127.667107634863));
#53455=CARTESIAN_POINT('Ctrl Pts',(19.1668970355953,1.36425684437746,127.70561854479));
#53456=CARTESIAN_POINT('Ctrl Pts',(18.5516662094274,1.51360466839347,127.744028818514));
#53457=CARTESIAN_POINT('Ctrl Pts',(17.9307733025901,1.39894337967582,127.782335107277));
#53458=CARTESIAN_POINT('Ctrl Pts',(17.4123242174242,1.04167741959983,127.820535082458));
#53459=CARTESIAN_POINT('Ctrl Pts',(17.0859506034826,0.505353855619343,127.858624432456));
#53460=CARTESIAN_POINT('Ctrl Pts',(17.0073468000548,-0.115660539147105,
127.896603287419));
#53461=CARTESIAN_POINT('Ctrl Pts',(17.1887082901287,-0.712804426518825,
127.934463445259));
#53462=CARTESIAN_POINT('Ctrl Pts',(17.5968242247701,-1.18228848738728,127.972211070178));
#53463=CARTESIAN_POINT('Ctrl Pts',(18.1594647751005,-1.44338028586681,128.009830189198));
#53464=CARTESIAN_POINT('Ctrl Pts',(18.7773792661455,-1.45169262750987,128.04733985285));
#53465=CARTESIAN_POINT('Ctrl Pts',(19.3431050379592,-1.20800514227934,128.08469883111));
#53466=CARTESIAN_POINT('Ctrl Pts',(19.7588133155117,-0.755575471850324,
128.121972631757));
#53467=CARTESIAN_POINT('Ctrl Pts',(19.951297760402,-0.175292515373662,128.159067356881));
#53468=CARTESIAN_POINT('Ctrl Pts',(19.9034340295258,0.329415031944361,128.189872819389));
#53469=CARTESIAN_POINT('Ctrl Pts',(19.7415614504299,0.695520735101091,128.214527494858));
#53470=CARTESIAN_POINT('Ctrl Pts',(19.565222236119,0.937848553101471,128.232911803911));
#53471=CARTESIAN_POINT('Ctrl Pts',(19.3448274084493,1.13736399322295,128.251234940316));
#53472=CARTESIAN_POINT('Ctrl Pts',(19.091755510318,1.28568634008855,128.269574561488));
#53473=CARTESIAN_POINT('Ctrl Pts',(18.8137135895315,1.37704884322017,128.28795209244));
#53474=CARTESIAN_POINT('Ctrl Pts',(18.6151599929778,1.39831377343028,128.300122981779));
#53475=CARTESIAN_POINT('Ctrl Pts',(18.5130392122771,1.39917328141053,128.306168212023));
#53476=CARTESIAN_POINT('Ctrl Pts',(18.5113516871238,1.39953897393561,113.105914026714));
#53477=CARTESIAN_POINT('Ctrl Pts',(18.3589863122547,1.39825657818145,113.114933579443));
#53478=CARTESIAN_POINT('Ctrl Pts',(18.1642992852404,1.36721421031762,113.127075590873));
#53479=CARTESIAN_POINT('Ctrl Pts',(17.8942839195588,1.26218430764902,113.145316932379));
#53480=CARTESIAN_POINT('Ctrl Pts',(17.6851880183204,1.13963755329772,113.16047473423));
#53481=CARTESIAN_POINT('Ctrl Pts',(17.4673934822047,0.942389681177235,113.178581302361));
#53482=CARTESIAN_POINT('Ctrl Pts',(17.2940773743872,0.70403936319175,113.196661733656));
#53483=CARTESIAN_POINT('Ctrl Pts',(17.1357187151386,0.345774791719098,113.220785229217));
#53484=CARTESIAN_POINT('Ctrl Pts',(17.0894823718046,-0.145861162010181,
113.250790855953));
#53485=CARTESIAN_POINT('Ctrl Pts',(17.2759930636586,-0.706633555871871,
113.286647905341));
#53486=CARTESIAN_POINT('Ctrl Pts',(17.6749864517915,-1.14012578485946,113.322389111944));
#53487=CARTESIAN_POINT('Ctrl Pts',(18.2137084295675,-1.37171410552075,113.357954662974));
#53488=CARTESIAN_POINT('Ctrl Pts',(18.7974084932161,-1.36336584604869,113.393386644682));
#53489=CARTESIAN_POINT('Ctrl Pts',(19.3247627673478,-1.11816214646004,113.428659966589));
#53490=CARTESIAN_POINT('Ctrl Pts',(19.7041885325999,-0.680967221982905,
113.463785874814));
#53491=CARTESIAN_POINT('Ctrl Pts',(19.8712822536032,-0.129268651081804,
113.498757168997));
#53492=CARTESIAN_POINT('Ctrl Pts',(19.7987670025229,0.440037112002971,113.533576759984));
#53493=CARTESIAN_POINT('Ctrl Pts',(19.5013596035167,0.927912782061419,113.568241981718));
#53494=CARTESIAN_POINT('Ctrl Pts',(19.0327193807973,1.25032157235679,113.602753439165));
#53495=CARTESIAN_POINT('Ctrl Pts',(18.4757666540105,1.35273464100996,113.63711018654));
#53496=CARTESIAN_POINT('Ctrl Pts',(17.9280414761478,1.21933376337218,113.67131219649));
#53497=CARTESIAN_POINT('Ctrl Pts',(17.4845929117289,0.875417320108831,113.705359156385));
#53498=CARTESIAN_POINT('Ctrl Pts',(17.2214967953587,0.382626263301629,113.739251050795));
#53499=CARTESIAN_POINT('Ctrl Pts',(17.1828026342533,-0.172095488110439,
113.772987868005));
#53500=CARTESIAN_POINT('Ctrl Pts',(17.3731808698039,-0.691842439720159,
113.806569762154));
#53501=CARTESIAN_POINT('Ctrl Pts',(17.7574604796447,-1.08667234074387,113.839996948255));
#53502=CARTESIAN_POINT('Ctrl Pts',(18.2671343378151,-1.28916901243406,113.873269790971));
#53503=CARTESIAN_POINT('Ctrl Pts',(18.8125146649335,-1.26594080045812,113.906388695895));
#53504=CARTESIAN_POINT('Ctrl Pts',(19.2985966148297,-1.02310331013343,113.93935427002));
#53505=CARTESIAN_POINT('Ctrl Pts',(19.6414920790201,-0.604858544715025,
113.972167107524));
#53506=CARTESIAN_POINT('Ctrl Pts',(19.7830009043026,-0.0854650173762428,
114.004828006579));
#53507=CARTESIAN_POINT('Ctrl Pts',(19.7004051738126,0.443986345750033,114.037337813179));
#53508=CARTESIAN_POINT('Ctrl Pts',(19.4101107233049,0.891426522117437,114.069697472386));
#53509=CARTESIAN_POINT('Ctrl Pts',(18.9644376547088,1.17997469370865,114.101908096569));
#53510=CARTESIAN_POINT('Ctrl Pts',(18.5292359593294,1.2473874871807,114.128626980292));
#53511=CARTESIAN_POINT('Ctrl Pts',(18.1884808231005,1.1915529185394,114.149928831447));
#53512=CARTESIAN_POINT('Ctrl Pts',(17.867350669578,1.06670828297356,114.171182018965));
#53513=CARTESIAN_POINT('Ctrl Pts',(17.5301291320079,0.789751537535966,114.197657653242));
#53514=CARTESIAN_POINT('Ctrl Pts',(17.2976207784108,0.323162814182794,114.229284668447));
#53515=CARTESIAN_POINT('Ctrl Pts',(17.2760307589781,-0.195322300576695,
114.260769422979));
#53516=CARTESIAN_POINT('Ctrl Pts',(17.4672530148769,-0.675270737380106,
114.292113588026));
#53517=CARTESIAN_POINT('Ctrl Pts',(17.8361784311516,-1.03365374413639,114.323318935717));
#53518=CARTESIAN_POINT('Ctrl Pts',(18.3171896252618,-1.20932699187921,114.354387290873));
#53519=CARTESIAN_POINT('Ctrl Pts',(18.8257788687749,-1.17336834058296,114.385320598929));
#53520=CARTESIAN_POINT('Ctrl Pts',(19.2733928879841,-0.933855304247329,
114.416120915472));
#53521=CARTESIAN_POINT('Ctrl Pts',(19.5828209898627,-0.534110071302645,
114.446790313512));
#53522=CARTESIAN_POINT('Ctrl Pts',(19.7014910385769,-0.0449140169986757,
114.477331070014));
#53523=CARTESIAN_POINT('Ctrl Pts',(19.6103829036543,0.448052163986159,114.507745421826));
#53524=CARTESIAN_POINT('Ctrl Pts',(19.3270409336854,0.859114585275451,114.538035790502));
#53525=CARTESIAN_POINT('Ctrl Pts',(18.902219003043,1.11756691087476,114.568204633005));
#53526=CARTESIAN_POINT('Ctrl Pts',(18.4108359765105,1.17971542272961,114.598254500916));
#53527=CARTESIAN_POINT('Ctrl Pts',(17.938757082736,1.03630336296344,114.628188026478));
#53528=CARTESIAN_POINT('Ctrl Pts',(17.5678384414828,0.713813950315308,114.658007922532));
#53529=CARTESIAN_POINT('Ctrl Pts',(17.3617553520377,0.269607479199184,114.687716968681));
#53530=CARTESIAN_POINT('Ctrl Pts',(17.3550963866736,-0.218243764897947,
114.717318043725));
#53531=CARTESIAN_POINT('Ctrl Pts',(17.5475950744081,-0.664690998735179,
114.7468140547));
#53532=CARTESIAN_POINT('Ctrl Pts',(17.9043991100135,-0.992416595278079,
114.776208065471));
#53533=CARTESIAN_POINT('Ctrl Pts',(18.3624169483923,-1.14535975384611,114.805503046249));
#53534=CARTESIAN_POINT('Ctrl Pts',(18.7615170178427,-1.10585452867801,114.829835796926));
#53535=CARTESIAN_POINT('Ctrl Pts',(19.0496294954737,-0.978997161595419,
114.849255587645));
#53536=CARTESIAN_POINT('Ctrl Pts',(19.3048574786947,-0.79553250362716,114.868645042624));
#53537=CARTESIAN_POINT('Ctrl Pts',(19.5399712571078,-0.473714416566306,
114.892826185557));
#53538=CARTESIAN_POINT('Ctrl Pts',(19.6393850634584,-0.00730971802335478,
114.921757393726));
#53539=CARTESIAN_POINT('Ctrl Pts',(19.5399625820036,0.457663098314685,114.950606072505));
#53540=CARTESIAN_POINT('Ctrl Pts',(19.2600489521841,0.8404401746431,114.979375535716));
#53541=CARTESIAN_POINT('Ctrl Pts',(18.8493002660062,1.0748791204869,115.008069367643));
#53542=CARTESIAN_POINT('Ctrl Pts',(18.3798045540622,1.12100379325741,115.03669105096));
#53543=CARTESIAN_POINT('Ctrl Pts',(17.9334761702293,0.971691728884436,115.065244271503));
#53544=CARTESIAN_POINT('Ctrl Pts',(17.5878676214356,0.65385534597262,115.093732542151));
#53545=CARTESIAN_POINT('Ctrl Pts',(17.4025647057155,0.223459828864383,115.122159793198));
#53546=CARTESIAN_POINT('Ctrl Pts',(17.4085502873789,-0.19209819495059,115.147377124544));
#53547=CARTESIAN_POINT('Ctrl Pts',(17.5367356176809,-0.527142367594399,
115.169408004386));
#53548=CARTESIAN_POINT('Ctrl Pts',(17.6750977312951,-0.711158333094599,
115.183552912859));
#53549=CARTESIAN_POINT('Ctrl Pts',(17.7863885808917,-0.814774883732063,
115.192976963383));
#53550=CARTESIAN_POINT('Ctrl Pts',(17.8454247819276,-0.862585781096137,
115.197687300119));
#53551=CARTESIAN_POINT('Ctrl Pts',(17.9077104618947,-0.906089824707936,
115.202396522212));
#53552=CARTESIAN_POINT('Ctrl Pts',(18.0379443370074,-0.984212744282978,
115.211811648537));
#53553=CARTESIAN_POINT('Ctrl Pts',(18.2526617065583,-1.06613325129506,115.225926301068));
#53554=CARTESIAN_POINT('Ctrl Pts',(18.5576019510004,-1.0918497608244,115.244724894711));
#53555=CARTESIAN_POINT('Ctrl Pts',(18.8575606192194,-1.03215987599148,115.263506537009));
#53556=CARTESIAN_POINT('Ctrl Pts',(19.1288588143958,-0.891952186562153,
115.28227013416));
#53557=CARTESIAN_POINT('Ctrl Pts',(19.3508251361679,-0.682207124521765,
115.301018799015));
#53558=CARTESIAN_POINT('Ctrl Pts',(19.5054574638842,-0.419560801893519,
115.319752073714));
#53559=CARTESIAN_POINT('Ctrl Pts',(19.6077308631518,-0.0259263154196786,
115.344712356295));
#53560=CARTESIAN_POINT('Ctrl Pts',(19.5377477746489,0.38586915460951,115.369647933046));
#53561=CARTESIAN_POINT('Ctrl Pts',(19.3396914214431,0.680822124532718,115.391448755122));
#53562=CARTESIAN_POINT('Ctrl Pts',(19.1956630207076,0.821138998095959,115.403902493605));
#53563=CARTESIAN_POINT('Ctrl Pts',(19.0330562168647,0.939881008679034,115.416353054312));
#53564=CARTESIAN_POINT('Ctrl Pts',(18.8713590570001,1.01232560464736,115.427243762488));
#53565=CARTESIAN_POINT('Ctrl Pts',(18.725228959151,1.04886022864609,115.436577314987));
#53566=CARTESIAN_POINT('Ctrl Pts',(18.6511396870949,1.06199516467199,115.441243483769));
#53567=CARTESIAN_POINT('Ctrl Pts',(18.5887552060792,1.06860250803456,115.445131759822));
#53568=CARTESIAN_POINT('Ctrl Pts',(18.5386687908435,1.07119204246765,115.448241987292));
#53569=CARTESIAN_POINT('Ctrl Pts',(18.335367217824,1.07507497226287,115.460855897531));
#53570=CARTESIAN_POINT('Ctrl Pts',(17.9664424762471,0.980875509761386,115.483744741735));
#53571=CARTESIAN_POINT('Ctrl Pts',(17.6520792257115,0.689325937350842,115.509534368755));
#53572=CARTESIAN_POINT('Ctrl Pts',(17.5121694936909,0.42613007298751,115.527953977153));
#53573=CARTESIAN_POINT('Ctrl Pts',(17.4645396133996,0.2850154477201,115.537163914722));
#53574=CARTESIAN_POINT('Ctrl Pts',(17.441120994326,0.168435469558622,115.544532136209));
#53575=CARTESIAN_POINT('Ctrl Pts',(17.4131560783799,-0.0676969984065009,
115.559267961778));
#53576=CARTESIAN_POINT('Ctrl Pts',(17.4823658039121,-0.459825862112777,
115.583215931233));
#53577=CARTESIAN_POINT('Ctrl Pts',(17.8262853295745,-0.891269399178329,
115.616384804494));
#53578=CARTESIAN_POINT('Ctrl Pts',(18.2924680185614,-1.08762744645822,115.64680542441));
#53579=CARTESIAN_POINT('Ctrl Pts',(18.7462270489574,-1.0703230621042,115.674477878059));
#53580=CARTESIAN_POINT('Ctrl Pts',(19.1209344877883,-0.907026557236116,
115.699399300559));
#53581=CARTESIAN_POINT('Ctrl Pts',(19.4103418070842,-0.617613192611829,
115.724339949641));
#53582=CARTESIAN_POINT('Ctrl Pts',(19.546765896882,-0.304888187420353,115.745141645372));
#53583=CARTESIAN_POINT('Ctrl Pts',(19.581845245331,-0.0374613907239736,
115.76179592779));
#53584=CARTESIAN_POINT('Ctrl Pts',(19.5705544130237,0.16452246986593,115.774292242788));
#53585=CARTESIAN_POINT('Ctrl Pts',(19.5299314232032,0.3283161944619,115.78471254347));
#53586=CARTESIAN_POINT('Ctrl Pts',(19.4795616558565,0.453109334487188,115.793051979174));
#53587=CARTESIAN_POINT('Ctrl Pts',(19.3869833795747,0.632584070260413,115.805564455334));
#53588=CARTESIAN_POINT('Ctrl Pts',(19.1860046219035,0.866177552115459,115.824348246596));
#53589=CARTESIAN_POINT('Ctrl Pts',(18.8222879048801,1.05846861458212,115.84942542723));
#53590=CARTESIAN_POINT('Ctrl Pts',(18.4128715286235,1.10465772425926,115.874538537355));
#53591=CARTESIAN_POINT('Ctrl Pts',(18.1139470962793,1.02460139690338,115.8934021608));
#53592=CARTESIAN_POINT('Ctrl Pts',(17.935263979171,0.927889961734541,115.905990634769));
#53593=CARTESIAN_POINT('Ctrl Pts',(17.8226045130323,0.852641962694081,115.91438613578));
#53594=CARTESIAN_POINT('Ctrl Pts',(17.6450265571346,0.694036087225085,115.929088683311));
#53595=CARTESIAN_POINT('Ctrl Pts',(17.5255867282254,0.504314599272793,115.942757778983));
#53596=CARTESIAN_POINT('Ctrl Pts',(17.4674220030132,0.344811226726132,115.953283647491));
#53597=CARTESIAN_POINT('Ctrl Pts',(17.4521496715754,0.296233089264299,115.956442243962));
#53598=CARTESIAN_POINT('Ctrl Pts',(17.439207974003,0.246949331300578,115.959601506988));
#53599=CARTESIAN_POINT('Ctrl Pts',(17.4285669872276,0.197121087776645,115.962761544684));
#53600=CARTESIAN_POINT('Ctrl Pts',(17.4202486700005,0.146830936758464,115.965922273101));
#53601=CARTESIAN_POINT('Ctrl Pts',(17.412357915538,0.0793192050127272,115.970137566166));
#53602=CARTESIAN_POINT('Ctrl Pts',(17.4034732364542,-0.107616603328217,
115.981733364604));
#53603=CARTESIAN_POINT('Ctrl Pts',(17.461377849773,-0.41387644231022,116.000732291017));
#53604=CARTESIAN_POINT('Ctrl Pts',(17.6828616627857,-0.766524560243698,
116.026114794632));
#53605=CARTESIAN_POINT('Ctrl Pts',(18.0185767554592,-1.01440331549217,116.051551886574));
#53606=CARTESIAN_POINT('Ctrl Pts',(18.4225665632467,-1.12273838760728,116.077045286512));
#53607=CARTESIAN_POINT('Ctrl Pts',(18.83912791779,-1.07589746406352,116.102598001197));
#53608=CARTESIAN_POINT('Ctrl Pts',(19.2107527297005,-0.8796214031171,116.128212039234));
#53609=CARTESIAN_POINT('Ctrl Pts',(19.424451551719,-0.631313603440492,116.148184292881));
#53610=CARTESIAN_POINT('Ctrl Pts',(19.5271584694527,-0.424547170861779,
116.162474157721));
#53611=CARTESIAN_POINT('Ctrl Pts',(19.5880911897583,-0.250123727488174,
116.173916708735));
#53612=CARTESIAN_POINT('Ctrl Pts',(19.6371899862326,0.072010671089548,116.193966675555));
#53613=CARTESIAN_POINT('Ctrl Pts',(19.5312491458833,0.537649088107642,116.22268737364));
#53614=CARTESIAN_POINT('Ctrl Pts',(19.1506475461343,0.969263331407848,116.257281026004));
#53615=CARTESIAN_POINT('Ctrl Pts',(18.6080789065826,1.16704974088591,116.292009350826));
#53616=CARTESIAN_POINT('Ctrl Pts',(18.0345517634555,1.08093962226307,116.326877318219));
#53617=CARTESIAN_POINT('Ctrl Pts',(17.6379610394385,0.780764466937685,116.356784161276));
#53618=CARTESIAN_POINT('Ctrl Pts',(17.4326718707591,0.431520171549925,116.381667699098));
#53619=CARTESIAN_POINT('Ctrl Pts',(17.3243036095994,0.0153408501438764,
116.408079506778));
#53620=CARTESIAN_POINT('Ctrl Pts',(17.4168359598342,-0.532483913432153,
116.441216842383));
#53621=CARTESIAN_POINT('Ctrl Pts',(17.8631699482747,-1.03264209362388,116.481184742038));
#53622=CARTESIAN_POINT('Ctrl Pts',(18.5104604520464,-1.21960339016096,116.521361981733));
#53623=CARTESIAN_POINT('Ctrl Pts',(19.1614492145997,-1.03262237061467,116.561754669311));
#53624=CARTESIAN_POINT('Ctrl Pts',(19.6158431880161,-0.525056657258863,
116.602368748702));
#53625=CARTESIAN_POINT('Ctrl Pts',(19.711601838574,0.0374389790684584,116.636402738718));
#53626=CARTESIAN_POINT('Ctrl Pts',(19.5996504879164,0.468431902550626,116.66374624569));
#53627=CARTESIAN_POINT('Ctrl Pts',(19.4300177437899,0.75701849348732,116.684312306879));
#53628=CARTESIAN_POINT('Ctrl Pts',(19.185748019025,0.98745395999935,116.704937967889));
#53629=CARTESIAN_POINT('Ctrl Pts',(18.7872001223434,1.19443636121172,116.732518393314));
#53630=CARTESIAN_POINT('Ctrl Pts',(18.2076140535373,1.22767049755924,116.767145372071));
#53631=CARTESIAN_POINT('Ctrl Pts',(17.5937432616692,0.889007641910738,116.808944015097));
#53632=CARTESIAN_POINT('Ctrl Pts',(17.2521681574792,0.272180427293588,116.850993272138));
#53633=CARTESIAN_POINT('Ctrl Pts',(17.2913162457654,-0.436194779844278,
116.893296892387));
#53634=CARTESIAN_POINT('Ctrl Pts',(17.7038571015148,-1.01864243864716,116.935858467641));
#53635=CARTESIAN_POINT('Ctrl Pts',(18.3670800933445,-1.29404223866986,116.978681197049));
#53636=CARTESIAN_POINT('Ctrl Pts',(19.0795409122072,-1.17362287387417,117.021768008785));
#53637=CARTESIAN_POINT('Ctrl Pts',(19.6220674999244,-0.689641540177797,
117.065121491555));
#53638=CARTESIAN_POINT('Ctrl Pts',(19.8251990236932,0.0131357064283045,
117.108743921761));
#53639=CARTESIAN_POINT('Ctrl Pts',(19.6220412864902,0.720631070474546,117.152637244666));
#53640=CARTESIAN_POINT('Ctrl Pts',(19.0702069383145,1.21464681696053,117.196803085261));
#53641=CARTESIAN_POINT('Ctrl Pts',(18.3355975639786,1.34012022714546,117.241242736065));
#53642=CARTESIAN_POINT('Ctrl Pts',(17.6425703116435,1.05376306472665,117.285957159459));
#53643=CARTESIAN_POINT('Ctrl Pts',(17.2054487318153,0.438821315496588,117.330946987677));
#53644=CARTESIAN_POINT('Ctrl Pts',(17.1622294713761,-0.319048897988897,
117.376212520113));
#53645=CARTESIAN_POINT('Ctrl Pts',(17.531095775153,-0.98778618784794,117.421753723563));
#53646=CARTESIAN_POINT('Ctrl Pts',(18.2032302806575,-1.36002403472624,117.467570232336));
#53647=CARTESIAN_POINT('Ctrl Pts',(18.9750292819446,-1.31731515605936,117.513661349979));
#53648=CARTESIAN_POINT('Ctrl Pts',(19.6094611826802,-0.867937834405175,
117.560026043846));
#53649=CARTESIAN_POINT('Ctrl Pts',(19.9094757960212,-0.145559704600647,
117.60666296168));
#53650=CARTESIAN_POINT('Ctrl Pts',(19.7999774806316,0.500689885182389,117.645752497943));
#53651=CARTESIAN_POINT('Ctrl Pts',(19.5150122013445,0.925278807945587,117.677158402211));
#53652=CARTESIAN_POINT('Ctrl Pts',(19.1240773404713,1.25704056473757,117.708653378912));
#53653=CARTESIAN_POINT('Ctrl Pts',(18.4872767009066,1.44128037713583,117.748188539166));
#53654=CARTESIAN_POINT('Ctrl Pts',(17.7182695158132,1.22028704524381,117.795894191709));
#53655=CARTESIAN_POINT('Ctrl Pts',(17.1818536479469,0.6209694352788,117.84386042374));
#53656=CARTESIAN_POINT('Ctrl Pts',(17.0457729949993,-0.176241227277537,
117.892083891781));
#53657=CARTESIAN_POINT('Ctrl Pts',(17.356339229752,-0.927521629412933,117.940561028213));
#53658=CARTESIAN_POINT('Ctrl Pts',(18.0224285226418,-1.40087677191055,117.989287906266));
#53659=CARTESIAN_POINT('Ctrl Pts',(18.8423662647727,-1.44747689273984,118.038260331711));
#53660=CARTESIAN_POINT('Ctrl Pts',(19.564973581273,-1.04879126733954,118.087473779158));
#53661=CARTESIAN_POINT('Ctrl Pts',(19.9665731208934,-0.323199709536255,
118.136923494836));
#53662=CARTESIAN_POINT('Ctrl Pts',(19.9204307603646,0.508545196077463,118.186604326532));
#53663=CARTESIAN_POINT('Ctrl Pts',(19.4364850154724,1.19163922937571,118.236511041213));
#53664=CARTESIAN_POINT('Ctrl Pts',(18.7896014129428,1.45977975239074,118.278283324362));
#53665=CARTESIAN_POINT('Ctrl Pts',(18.2437658807907,1.44350219297019,118.311808461719));
#53666=CARTESIAN_POINT('Ctrl Pts',(17.8529857116712,1.31941501771739,118.337004909982));
#53667=CARTESIAN_POINT('Ctrl Pts',(17.5111199319821,1.09085297848017,118.362253631037));
#53668=CARTESIAN_POINT('Ctrl Pts',(17.2453545367621,0.776316639682611,118.387553332054));
#53669=CARTESIAN_POINT('Ctrl Pts',(17.0767100831229,0.399529811958646,118.412903698764));
#53670=CARTESIAN_POINT('Ctrl Pts',(17.0188671438186,-0.00986043940601462,
118.438303460264));
#53671=CARTESIAN_POINT('Ctrl Pts',(17.0766989112945,-0.420209281010889,
118.463752185059));
#53672=CARTESIAN_POINT('Ctrl Pts',(17.2180009588825,-0.735846803400231,
118.484999124376));
#53673=CARTESIAN_POINT('Ctrl Pts',(17.3803055651797,-0.958070010311263,
118.502020602052));
#53674=CARTESIAN_POINT('Ctrl Pts',(17.5723108800011,-1.15519143488245,118.519057008924));
#53675=CARTESIAN_POINT('Ctrl Pts',(17.976044057097,-1.42626434895589,118.548911965511));
#53676=CARTESIAN_POINT('Ctrl Pts',(18.6825732967982,-1.5469332305085,118.591674536592));
#53677=CARTESIAN_POINT('Ctrl Pts',(19.480862487031,-1.21670551212833,118.643163512056));
#53678=CARTESIAN_POINT('Ctrl Pts',(19.898397453744,-0.628314262383973,118.686209676539));
#53679=CARTESIAN_POINT('Ctrl Pts',(19.9934589586098,-0.145556018009749,
118.716410875295));
#53680=CARTESIAN_POINT('Ctrl Pts',(19.9897381597335,0.133405879333075,118.733688581356));
#53681=CARTESIAN_POINT('Ctrl Pts',(19.9468629952409,0.409779100114465,118.75097829491));
#53682=CARTESIAN_POINT('Ctrl Pts',(19.8210589677851,0.738453944597032,118.772614532919));
#53683=CARTESIAN_POINT('Ctrl Pts',(19.482458213577,1.19036691859332,118.807280917743));
#53684=CARTESIAN_POINT('Ctrl Pts',(18.8455916039526,1.54286230442063,118.850703191666));
#53685=CARTESIAN_POINT('Ctrl Pts',(17.9707351056379,1.49403227262935,118.902943815855));
#53686=CARTESIAN_POINT('Ctrl Pts',(17.2543258704413,0.986046184208814,118.955310331053));
#53687=CARTESIAN_POINT('Ctrl Pts',(16.9736545538739,0.308628892705175,118.999046375777));
#53688=CARTESIAN_POINT('Ctrl Pts',(16.9908076007375,-0.261884195942545,
119.034089856028));
#53689=CARTESIAN_POINT('Ctrl Pts',(17.0986304843311,-0.60187232667865,119.056013023723));
#53690=CARTESIAN_POINT('Ctrl Pts',(17.2220725601196,-0.817412115664082,
119.071370791807));
#53691=CARTESIAN_POINT('Ctrl Pts',(17.3046947454948,-0.932313588781289,
119.080149511234));
#53692=CARTESIAN_POINT('Ctrl Pts',(17.3953791605744,-1.041187868381,119.088930231404));
#53693=CARTESIAN_POINT('Ctrl Pts',(17.522559367852,-1.16486266553002,119.099909408076));
#53694=CARTESIAN_POINT('Ctrl Pts',(17.7518728090185,-1.33251390437618,119.117484980784));
#53695=CARTESIAN_POINT('Ctrl Pts',(18.0785092162954,-1.47873509889951,119.139467629877));
#53696=CARTESIAN_POINT('Ctrl Pts',(18.5041370739365,-1.5388357928971,119.165868977217));
#53697=CARTESIAN_POINT('Ctrl Pts',(18.9300650017773,-1.47872940044093,119.192290133091));
#53698=CARTESIAN_POINT('Ctrl Pts',(19.3230070662878,-1.30292433215567,119.218730941718));
#53699=CARTESIAN_POINT('Ctrl Pts',(19.6521414527707,-1.02501935198784,119.245189343596));
#53700=CARTESIAN_POINT('Ctrl Pts',(19.8916273980147,-0.666633644247205,
119.271665261632));
#53701=CARTESIAN_POINT('Ctrl Pts',(20.022628534436,-0.255704738726529,119.298156046695));
#53702=CARTESIAN_POINT('Ctrl Pts',(20.0347268900414,0.175649279097044,119.324662499476));
#53703=CARTESIAN_POINT('Ctrl Pts',(19.944906803099,0.524066451041732,119.346761205289));
#53704=CARTESIAN_POINT('Ctrl Pts',(19.817156023757,0.779729444103676,119.364447186537));
#53705=CARTESIAN_POINT('Ctrl Pts',(19.6147295341782,1.07423777764439,119.386558876142));
#53706=CARTESIAN_POINT('Ctrl Pts',(19.2202188753249,1.39809308905388,119.417528285369));
#53707=CARTESIAN_POINT('Ctrl Pts',(18.5867241883604,1.57103813761991,119.457366923459));
#53708=CARTESIAN_POINT('Ctrl Pts',(17.9376186369372,1.47011788769029,119.4972223696));
#53709=CARTESIAN_POINT('Ctrl Pts',(17.3861508706095,1.11275405579027,119.537090587226));
#53710=CARTESIAN_POINT('Ctrl Pts',(17.028676399318,0.561178042742845,119.576967614436));
#53711=CARTESIAN_POINT('Ctrl Pts',(16.9276717633489,-0.0883484362600774,
119.616849261155));
#53712=CARTESIAN_POINT('Ctrl Pts',(17.1007536383431,-0.722549055594297,
119.656731792094));
#53713=CARTESIAN_POINT('Ctrl Pts',(17.448299666744,-1.14590146394558,119.689964100819));
#53714=CARTESIAN_POINT('Ctrl Pts',(17.8117792744431,-1.37737020083668,119.716546697506));
#53715=CARTESIAN_POINT('Ctrl Pts',(18.215243549761,-1.52858309297296,119.743125722118));
#53716=CARTESIAN_POINT('Ctrl Pts',(18.762237993062,-1.55167189010214,119.776342653443));
#53717=CARTESIAN_POINT('Ctrl Pts',(19.3724575824767,-1.30880681937892,119.816187384569));
#53718=CARTESIAN_POINT('Ctrl Pts',(19.8300303495297,-0.838178157233193,
119.856012717496));
#53719=CARTESIAN_POINT('Ctrl Pts',(20.0553319706966,-0.222028446015196,
119.895814549444));
#53720=CARTESIAN_POINT('Ctrl Pts',(20.0093412860961,0.431937143886497,119.935588953089));
#53721=CARTESIAN_POINT('Ctrl Pts',(19.7004996494563,1.0096265526074,119.975331924619));
#53722=CARTESIAN_POINT('Ctrl Pts',(19.1830809519466,1.41042933555735,120.015039549248));
#53723=CARTESIAN_POINT('Ctrl Pts',(18.5477417148256,1.56476304383288,120.054707867703));
#53724=CARTESIAN_POINT('Ctrl Pts',(17.9054220875877,1.44629301140049,120.094333047644));
#53725=CARTESIAN_POINT('Ctrl Pts',(17.457794562179,1.13785264331078,120.127314767186));
#53726=CARTESIAN_POINT('Ctrl Pts',(17.1987941750473,0.797975612371571,120.15367472761));
#53727=CARTESIAN_POINT('Ctrl Pts',(17.0158521800977,0.412114272847593,120.180017209918));
#53728=CARTESIAN_POINT('Ctrl Pts',(16.947623315073,-0.125744883561413,120.212910946089));
#53729=CARTESIAN_POINT('Ctrl Pts',(17.136323471403,-0.747393162690755,120.252325078772));
#53730=CARTESIAN_POINT('Ctrl Pts',(17.5617842077802,-1.23696498855081,120.291677025785));
#53731=CARTESIAN_POINT('Ctrl Pts',(18.1491297132522,-1.50960991539734,120.330963166602));
#53732=CARTESIAN_POINT('Ctrl Pts',(18.7954584704689,-1.51854825462399,120.370179815259));
#53733=CARTESIAN_POINT('Ctrl Pts',(19.3879619651131,-1.26319238361003,120.409323412335));
#53734=CARTESIAN_POINT('Ctrl Pts',(19.8236300342295,-0.789026463960243,
120.448390403264));
#53735=CARTESIAN_POINT('Ctrl Pts',(20.0272069290065,-0.179520794684316,
120.487377310988));
#53736=CARTESIAN_POINT('Ctrl Pts',(19.9642079867834,0.458605653018268,120.526280699406));
#53737=CARTESIAN_POINT('Ctrl Pts',(19.6467700311826,1.01409833734176,120.565097195004));
#53738=CARTESIAN_POINT('Ctrl Pts',(19.1313271507666,1.39060526020685,120.603823479438));
#53739=CARTESIAN_POINT('Ctrl Pts',(18.5085629232136,1.52341751453039,120.642456297882));
#53740=CARTESIAN_POINT('Ctrl Pts',(17.8874269014854,1.39060921920092,120.680992458869));
#53741=CARTESIAN_POINT('Ctrl Pts',(17.376040183818,1.01665067198976,120.71942883698));
#53742=CARTESIAN_POINT('Ctrl Pts',(17.0628414097054,0.467903960283591,120.757762373191));
#53743=CARTESIAN_POINT('Ctrl Pts',(17.0012673452733,-0.159171624986709,
120.795990078213));
#53744=CARTESIAN_POINT('Ctrl Pts',(17.2006255114261,-0.755003713793607,
120.834109034869));
#53745=CARTESIAN_POINT('Ctrl Pts',(17.6247193648195,-1.21608511592836,120.87211640052));
#53746=CARTESIAN_POINT('Ctrl Pts',(18.1984219080174,-1.46298378556885,120.910009408484));
#53747=CARTESIAN_POINT('Ctrl Pts',(18.8210031809677,-1.45404564397339,120.947785368188));
#53748=CARTESIAN_POINT('Ctrl Pts',(19.3838435340945,-1.19242410821281,120.985441669183));
#53749=CARTESIAN_POINT('Ctrl Pts',(19.7894128883475,-0.725248797040647,
121.022975781176));
#53750=CARTESIAN_POINT('Ctrl Pts',(19.968194413284,-0.135131499300795,121.060385259496));
#53751=CARTESIAN_POINT('Ctrl Pts',(19.8906126551429,0.474463548421036,121.097667740759));
#53752=CARTESIAN_POINT('Ctrl Pts',(19.5719166839362,0.997380748400016,121.134820952923));
#53753=CARTESIAN_POINT('Ctrl Pts',(19.0692161746709,1.34329155662882,121.171842700173));
#53754=CARTESIAN_POINT('Ctrl Pts',(18.4712387268708,1.45330105771547,121.208730897588));
#53755=CARTESIAN_POINT('Ctrl Pts',(17.8826539013599,1.31000788465432,121.245483511077));
#53756=CARTESIAN_POINT('Ctrl Pts',(17.4057248129287,0.940178434972456,121.282098674275));
#53757=CARTESIAN_POINT('Ctrl Pts',(17.1225303971144,0.409857233817631,121.318574471326));
#53758=CARTESIAN_POINT('Ctrl Pts',(17.0808109556991,-0.18761576406713,121.354909351532));
#53759=CARTESIAN_POINT('Ctrl Pts',(17.234662884993,-0.60767734320799,121.382053320561));
#53760=CARTESIAN_POINT('Ctrl Pts',(17.4026562098279,-0.845818839371914,
121.400104492057));
#53761=CARTESIAN_POINT('Ctrl Pts',(17.5304295290375,-0.991852754127738,
121.412126298005));
#53762=CARTESIAN_POINT('Ctrl Pts',(17.7920501977231,-1.20994146748006,121.433133107686));
#53763=CARTESIAN_POINT('Ctrl Pts',(18.2502296129569,-1.39212149316642,121.463051648494));
#53764=CARTESIAN_POINT('Ctrl Pts',(18.8390918948479,-1.36703543517734,121.498806978423));
#53765=CARTESIAN_POINT('Ctrl Pts',(19.3641003985679,-1.10478925936658,121.534414063249));
#53766=CARTESIAN_POINT('Ctrl Pts',(19.7346755496411,-0.652838433166381,
121.569871802645));
#53767=CARTESIAN_POINT('Ctrl Pts',(19.8876619889454,-0.0913592885263403,
121.605179139474));
#53768=CARTESIAN_POINT('Ctrl Pts',(19.7983634546371,0.481182887673296,121.640335149));
#53769=CARTESIAN_POINT('Ctrl Pts',(19.4843596671287,0.96520447245087,121.675338992639));
#53770=CARTESIAN_POINT('Ctrl Pts',(19.0021632434605,1.27739010659383,121.710189943609));
#53771=CARTESIAN_POINT('Ctrl Pts',(18.4370107635688,1.3650059559128,121.744887374439));
#53772=CARTESIAN_POINT('Ctrl Pts',(17.8878131855026,1.21481569708191,121.779430764563));
#53773=CARTESIAN_POINT('Ctrl Pts',(17.4498271981239,0.855022050904291,121.813819696406));
#53774=CARTESIAN_POINT('Ctrl Pts',(17.19813616434,0.349998239521284,121.848053857948));
#53775=CARTESIAN_POINT('Ctrl Pts',(17.1747784662698,-0.211228605711279,
121.882133041112));
#53776=CARTESIAN_POINT('Ctrl Pts',(17.3817429545998,-0.73067256982998,121.916057144785));
#53777=CARTESIAN_POINT('Ctrl Pts',(17.780987988533,-1.11849653673519,121.949826170361));
#53778=CARTESIAN_POINT('Ctrl Pts',(18.3014175564027,-1.30855030916415,121.983440229557));
#53779=CARTESIAN_POINT('Ctrl Pts',(18.8515390403575,-1.26963899436222,122.016899529174));
#53780=CARTESIAN_POINT('Ctrl Pts',(19.3355425449402,-1.01063164342207,122.050204399541));
#53781=CARTESIAN_POINT('Ctrl Pts',(19.6699894411733,-0.578525953406879,
122.083355241515));
#53782=CARTESIAN_POINT('Ctrl Pts',(19.7981784976235,-0.049975975244043,
122.116352625486));
#53783=CARTESIAN_POINT('Ctrl Pts',(19.6997563641334,0.482371917081139,122.149197120449));
#53784=CARTESIAN_POINT('Ctrl Pts',(19.3939165927788,0.926015911083455,122.181889518331));
#53785=CARTESIAN_POINT('Ctrl Pts',(18.9356726261446,1.20475735757232,122.214430632586));
#53786=CARTESIAN_POINT('Ctrl Pts',(18.4060062045841,1.27170816166094,122.246821402389));
#53787=CARTESIAN_POINT('Ctrl Pts',(17.8975424573268,1.11719794305827,122.279062885459));
#53788=CARTESIAN_POINT('Ctrl Pts',(17.4983771377944,0.770086744703878,122.311156214457));
#53789=CARTESIAN_POINT('Ctrl Pts',(17.2768186093101,0.292410270944587,122.343102633485));
#53790=CARTESIAN_POINT('Ctrl Pts',(17.269719437291,-0.231700508547156,122.374903504129));
#53791=CARTESIAN_POINT('Ctrl Pts',(17.4763670890499,-0.710818699113158,
122.406560242296));
#53792=CARTESIAN_POINT('Ctrl Pts',(17.8589529235959,-1.06215785962516,122.438074418514));
#53793=CARTESIAN_POINT('Ctrl Pts',(18.3494690676881,-1.2258552099751,122.469447653676));
#53794=CARTESIAN_POINT('Ctrl Pts',(18.8617822651652,-1.17515551048656,122.500681677063));
#53795=CARTESIAN_POINT('Ctrl Pts',(19.306740267383,-0.92075115531246,122.531778343629));
#53796=CARTESIAN_POINT('Ctrl Pts',(19.6076666503762,-0.508600801661367,
122.562739531444));
#53797=CARTESIAN_POINT('Ctrl Pts',(19.7135494146674,-0.0116339705090276,
122.593567307384));
#53798=CARTESIAN_POINT('Ctrl Pts',(19.6076731364699,0.483114779154934,122.624263713906));
#53799=CARTESIAN_POINT('Ctrl Pts',(19.3102051188471,0.889762136113708,122.654831033973));
#53800=CARTESIAN_POINT('Ctrl Pts',(18.8744209204798,1.13840436181491,122.685271410186));
#53801=CARTESIAN_POINT('Ctrl Pts',(18.3771167267049,1.1871652605314,122.71558735378));
#53802=CARTESIAN_POINT('Ctrl Pts',(17.9051830307953,1.029208997682,122.745781222973));
#53803=CARTESIAN_POINT('Ctrl Pts',(17.5403703562541,0.693576750726723,122.77585559056));
#53804=CARTESIAN_POINT('Ctrl Pts',(17.3452208922813,0.240041357799779,122.805813070685));
#53805=CARTESIAN_POINT('Ctrl Pts',(17.3515208693343,-0.197222450308024,
122.832340402984));
#53806=CARTESIAN_POINT('Ctrl Pts',(17.4863244070343,-0.548895301526989,
122.85547963802));
#53807=CARTESIAN_POINT('Ctrl Pts',(17.7440611200262,-0.892625678754596,
122.881859502068));
#53808=CARTESIAN_POINT('Ctrl Pts',(18.2262426351603,-1.15890748220768,122.914714845542));
#53809=CARTESIAN_POINT('Ctrl Pts',(18.8833930837132,-1.12154607814807,122.953956867101));
#53810=CARTESIAN_POINT('Ctrl Pts',(19.417378773027,-0.742108947509844,122.993021846801));
#53811=CARTESIAN_POINT('Ctrl Pts',(19.6666571462621,-0.139392568668771,
123.031917160417));
#53812=CARTESIAN_POINT('Ctrl Pts',(19.557479197789,0.501041105718899,123.070650511539));
#53813=CARTESIAN_POINT('Ctrl Pts',(19.1979910414516,0.902623177622933,123.102799827228));
#53814=CARTESIAN_POINT('Ctrl Pts',(18.8164093817205,1.07240048839272,123.128446232696));
#53815=CARTESIAN_POINT('Ctrl Pts',(18.5184865862346,1.11482117402686,123.146934468807));
#53816=CARTESIAN_POINT('Ctrl Pts',(18.2324054828255,1.07857876720517,123.164681440727));
#53817=CARTESIAN_POINT('Ctrl Pts',(17.8891655916273,0.944438997380313,123.187362255959));
#53818=CARTESIAN_POINT('Ctrl Pts',(17.5443717314018,0.624378993516739,123.21564875382));
#53819=CARTESIAN_POINT('Ctrl Pts',(17.3952088655578,0.179660540296838,123.243854556847));
#53820=CARTESIAN_POINT('Ctrl Pts',(17.4140954128167,-0.185732646246057,
123.266373423675));
#53821=CARTESIAN_POINT('Ctrl Pts',(17.5212227395653,-0.535021075635455,
123.288863256363));
#53822=CARTESIAN_POINT('Ctrl Pts',(17.812244787014,-0.899924705335984,123.316922183842));
#53823=CARTESIAN_POINT('Ctrl Pts',(18.2842319058948,-1.09849765273693,123.347715096373));
#53824=CARTESIAN_POINT('Ctrl Pts',(18.7423557254701,-1.08094335039291,123.375655800996));
#53825=CARTESIAN_POINT('Ctrl Pts',(19.1198741467514,-0.916334604468255,
123.4007644734));
#53826=CARTESIAN_POINT('Ctrl Pts',(19.4107202134498,-0.625331903211328,
123.425837870652));
#53827=CARTESIAN_POINT('Ctrl Pts',(19.5749506858235,-0.248827358969858,
123.450878596324));
#53828=CARTESIAN_POINT('Ctrl Pts',(19.5902582672216,0.161256534828828,123.47588966774));
#53829=CARTESIAN_POINT('Ctrl Pts',(19.4548322547901,0.548086758583229,123.500873384082));
#53830=CARTESIAN_POINT('Ctrl Pts',(19.2322452136596,0.806774003836304,123.521673295525));
#53831=CARTESIAN_POINT('Ctrl Pts',(19.0068132440525,0.953991375109464,123.538302073525));
#53832=CARTESIAN_POINT('Ctrl Pts',(18.7169314442061,1.07461791635357,123.557694757307));
#53833=CARTESIAN_POINT('Ctrl Pts',(18.2799908654444,1.09642297116301,123.583995307696));
#53834=CARTESIAN_POINT('Ctrl Pts',(17.8656644604746,0.896711667502387,123.611657850074));
#53835=CARTESIAN_POINT('Ctrl Pts',(17.6214240384758,0.632872186368461,123.633778060455));
#53836=CARTESIAN_POINT('Ctrl Pts',(17.4927046928802,0.396360692377051,123.650363822077));
#53837=CARTESIAN_POINT('Ctrl Pts',(17.4034992587404,0.0481367539224208,
123.672474132222));
#53838=CARTESIAN_POINT('Ctrl Pts',(17.4549679685944,-0.361979267228126,
123.697342438129));
#53839=CARTESIAN_POINT('Ctrl Pts',(17.6965579170255,-0.745759415090237,
123.724971781578));
#53840=CARTESIAN_POINT('Ctrl Pts',(18.0382603256698,-0.998195883246386,
123.750875322465));
#53841=CARTESIAN_POINT('Ctrl Pts',(18.4698637772213,-1.10315324998456,123.777819593015));
#53842=CARTESIAN_POINT('Ctrl Pts',(18.9235437736981,-1.01950381091171,123.80580909134));
#53843=CARTESIAN_POINT('Ctrl Pts',(19.2719865687262,-0.779544885220034,
123.831478142263));
#53844=CARTESIAN_POINT('Ctrl Pts',(19.4438761068751,-0.527684719547219,
123.8501564127));
#53845=CARTESIAN_POINT('Ctrl Pts',(19.5392742119118,-0.295150402427171,
123.865727180495));
#53846=CARTESIAN_POINT('Ctrl Pts',(19.586310736526,-0.0588575645688193,
123.880524776365));
#53847=CARTESIAN_POINT('Ctrl Pts',(19.5607154879257,0.244538156461791,123.899226477669));
#53848=CARTESIAN_POINT('Ctrl Pts',(19.4520859293862,0.529189150664088,123.91794037051));
#53849=CARTESIAN_POINT('Ctrl Pts',(19.2687581561598,0.772802794422214,123.936666822134));
#53850=CARTESIAN_POINT('Ctrl Pts',(19.0249947092009,0.956277148756344,123.955407545818));
#53851=CARTESIAN_POINT('Ctrl Pts',(18.7634668055328,1.05614295662185,123.972600525356));
#53852=CARTESIAN_POINT('Ctrl Pts',(18.511720320822,1.08618824432886,123.988242368963));
#53853=CARTESIAN_POINT('Ctrl Pts',(18.2084450486932,1.05870460262302,124.007025488382));
#53854=CARTESIAN_POINT('Ctrl Pts',(17.8526151266173,0.905597689373487,124.030530147954));
#53855=CARTESIAN_POINT('Ctrl Pts',(17.5374400251935,0.562785005443856,124.058780242183));
#53856=CARTESIAN_POINT('Ctrl Pts',(17.3894936022145,0.120463896426673,124.087079007616));
#53857=CARTESIAN_POINT('Ctrl Pts',(17.4352024530028,-0.344609559390143,
124.115430101927));
#53858=CARTESIAN_POINT('Ctrl Pts',(17.6673292304641,-0.751235919597019,
124.1438373954));
#53859=CARTESIAN_POINT('Ctrl Pts',(18.0460913057333,-1.02818689353757,124.172304589377));
#53860=CARTESIAN_POINT('Ctrl Pts',(18.5059607229931,-1.12649870064859,124.200835414131));
#53861=CARTESIAN_POINT('Ctrl Pts',(18.9669634259195,-1.02818302776601,124.229433518268));
#53862=CARTESIAN_POINT('Ctrl Pts',(19.3485491824866,-0.749461895391517,
124.25810252464));
#53863=CARTESIAN_POINT('Ctrl Pts',(19.5836265981341,-0.338131649402405,
124.286845998617));
#53864=CARTESIAN_POINT('Ctrl Pts',(19.630327822603,0.134618946327238,124.315667460856));
#53865=CARTESIAN_POINT('Ctrl Pts',(19.479443753127,0.58648760418091,124.344570375802));
#53866=CARTESIAN_POINT('Ctrl Pts',(19.1562137849851,0.938351901614487,124.373558153265));
#53867=CARTESIAN_POINT('Ctrl Pts',(18.7161248921632,1.12808670585089,124.40263414441));
#53868=CARTESIAN_POINT('Ctrl Pts',(18.2354148456271,1.12150629368483,124.431801642351));
#53869=CARTESIAN_POINT('Ctrl Pts',(17.7978998529863,0.918503883878429,124.461063877912));
#53870=CARTESIAN_POINT('Ctrl Pts',(17.4803961934958,0.553291510869809,124.490424017647));
#53871=CARTESIAN_POINT('Ctrl Pts',(17.3392647593072,0.0886576147994413,
124.519885160673));
#53872=CARTESIAN_POINT('Ctrl Pts',(17.4004301179553,-0.394798461775283,
124.549450337333));
#53873=CARTESIAN_POINT('Ctrl Pts',(17.6546385235008,-0.812615333546038,
124.579122508661));
#53874=CARTESIAN_POINT('Ctrl Pts',(18.0588194470523,-1.09119301111203,124.608904563076));
#53875=CARTESIAN_POINT('Ctrl Pts',(18.543358419133,-1.1807302345264,124.638799314424));
#53876=CARTESIAN_POINT('Ctrl Pts',(19.0240583854348,-1.06410629338754,124.668809499231));
#53877=CARTESIAN_POINT('Ctrl Pts',(19.4167402982424,-0.76012623588515,124.698937775415));
#53878=CARTESIAN_POINT('Ctrl Pts',(19.6519563673511,-0.32051767699258,124.729186721845));
#53879=CARTESIAN_POINT('Ctrl Pts',(19.6872486278557,0.178847159515111,124.759558835612));
#53880=CARTESIAN_POINT('Ctrl Pts',(19.5147929916102,0.651019381077076,124.790056530126));
#53881=CARTESIAN_POINT('Ctrl Pts',(19.1630554166896,1.01308604539074,124.820682132959));
#53882=CARTESIAN_POINT('Ctrl Pts',(18.6921194093106,1.2007058017599,124.851437884561));
#53883=CARTESIAN_POINT('Ctrl Pts',(18.1834458222145,1.17952283900347,124.882325937953));
#53884=CARTESIAN_POINT('Ctrl Pts',(17.7258058475007,0.951436951498519,124.913348356572));
#53885=CARTESIAN_POINT('Ctrl Pts',(17.3998118739641,0.554588535229773,124.944507112499));
#53886=CARTESIAN_POINT('Ctrl Pts',(17.26373753905,0.0570046141073459,124.975804084871));
#53887=CARTESIAN_POINT('Ctrl Pts',(17.3431180960944,-0.455041055169738,
125.0072410587));
#53888=CARTESIAN_POINT('Ctrl Pts',(17.6259851648555,-0.891966644984383,
125.038819724726));
#53889=CARTESIAN_POINT('Ctrl Pts',(18.0646216855069,-1.17653632770684,125.070541677722));
#53890=CARTESIAN_POINT('Ctrl Pts',(18.5835903524298,-1.25749741759416,125.102408415057));
#53891=CARTESIAN_POINT('Ctrl Pts',(19.0926894321616,-1.11879529614231,125.134421335534));
#53892=CARTESIAN_POINT('Ctrl Pts',(19.5026149129719,-0.782711247384195,
125.166581738493));
#53893=CARTESIAN_POINT('Ctrl Pts',(19.7406123902142,-0.306315724372236,
125.198890823782));
#53894=CARTESIAN_POINT('Ctrl Pts',(19.763377196559,0.228205370079604,125.231349690489));
#53895=CARTESIAN_POINT('Ctrl Pts',(19.5649172248906,0.727715249646334,125.263959335904));
#53896=CARTESIAN_POINT('Ctrl Pts',(19.1779529512479,1.10434350393728,125.296720654766));
#53897=CARTESIAN_POINT('Ctrl Pts',(18.6685471091754,1.29093449008952,125.329634438753));
#53898=CARTESIAN_POINT('Ctrl Pts',(18.1248397471563,1.25301197202037,125.362701376505));
#53899=CARTESIAN_POINT('Ctrl Pts',(17.6418067436561,0.995129105561402,125.395922052864));
#53900=CARTESIAN_POINT('Ctrl Pts',(17.304675613873,0.560436926500678,125.429296948111));
#53901=CARTESIAN_POINT('Ctrl Pts',(17.1738931640657,0.0234819648278402,
125.462826437776));
#53902=CARTESIAN_POINT('Ctrl Pts',(17.2742957831578,-0.522569202305958,
125.496510792449));
#53903=CARTESIAN_POINT('Ctrl Pts',(17.5904222067807,-0.982091337162969,
125.530350177997));
#53904=CARTESIAN_POINT('Ctrl Pts',(18.0688496230519,-1.27374502034201,125.564344655041));
#53905=CARTESIAN_POINT('Ctrl Pts',(18.6272097306155,-1.34487226270198,125.598494178829));
#53906=CARTESIAN_POINT('Ctrl Pts',(19.1683660928709,-1.1809955468391,125.632798599234));
#53907=CARTESIAN_POINT('Ctrl Pts',(19.5973138861129,-0.808707366036644,
125.66725766123));
#53908=CARTESIAN_POINT('Ctrl Pts',(19.8378617402874,-0.291381019313683,
125.701871005098));
#53909=CARTESIAN_POINT('Ctrl Pts',(19.8461655054361,0.281611275571365,125.736638166297));
#53910=CARTESIAN_POINT('Ctrl Pts',(19.6187093753557,0.810340152829362,125.771558575736));
#53911=CARTESIAN_POINT('Ctrl Pts',(19.1932825865189,1.2017528384317,125.80663156022));
#53912=CARTESIAN_POINT('Ctrl Pts',(18.6427164183581,1.38605643974671,125.84185634338));
#53913=CARTESIAN_POINT('Ctrl Pts',(18.06241569551,1.32916466473217,125.877232046069));
#53914=CARTESIAN_POINT('Ctrl Pts',(17.5538188909499,1.03898710476137,125.912757686413));
#53915=CARTESIAN_POINT('Ctrl Pts',(17.2066554729585,0.564402394819162,125.948432180681));
#53916=CARTESIAN_POINT('Ctrl Pts',(17.0831057440289,-0.0129682738891071,
125.984254343941));
#53917=CARTESIAN_POINT('Ctrl Pts',(17.206661494287,-0.592804847205485,126.020222891627));
#53918=CARTESIAN_POINT('Ctrl Pts',(17.5576842541618,-1.07353244121064,126.056336440009));
#53919=CARTESIAN_POINT('Ctrl Pts',(18.0764978235536,-1.37013019917798,126.092593506525));
#53920=CARTESIAN_POINT('Ctrl Pts',(18.6735343577048,-1.42917975270743,126.128992511042));
#53921=CARTESIAN_POINT('Ctrl Pts',(19.244809461307,-1.23848730738719,126.165531776955));
#53922=CARTESIAN_POINT('Ctrl Pts',(19.6900510063658,-0.82954528750613,126.202209533138));
#53923=CARTESIAN_POINT('Ctrl Pts',(19.9303178180715,-0.27234395879086,126.239023914679));
#53924=CARTESIAN_POINT('Ctrl Pts',(19.9220090897997,0.336615072122217,126.275972963622));
#53925=CARTESIAN_POINT('Ctrl Pts',(19.6647751325692,0.891050062438758,126.31305462995));
#53926=CARTESIAN_POINT('Ctrl Pts',(19.2018945677896,1.2934708225086,126.350266774275));
#53927=CARTESIAN_POINT('Ctrl Pts',(18.6129942519167,1.47234279082316,126.387607168055));
#53928=CARTESIAN_POINT('Ctrl Pts',(18.0003383532154,1.39481561583623,126.425073498411));
#53929=CARTESIAN_POINT('Ctrl Pts',(17.4710441936286,1.07275201436481,126.462663362284));
#53930=CARTESIAN_POINT('Ctrl Pts',(17.1183317039518,0.560944190799558,126.50037427996));
#53931=CARTESIAN_POINT('Ctrl Pts',(17.005074408946,-0.0522090232566247,
126.538203675335));
#53932=CARTESIAN_POINT('Ctrl Pts',(17.1525942214981,-0.660000712358473,
126.576148919226));
#53933=CARTESIAN_POINT('Ctrl Pts',(17.5366335567734,-1.15599588704851,126.61420725445));
#53934=CARTESIAN_POINT('Ctrl Pts',(18.091387243059,-1.45273381657987,126.652375940072));
#53935=CARTESIAN_POINT('Ctrl Pts',(18.7206933102241,-1.49710973462917,126.690651984097));
#53936=CARTESIAN_POINT('Ctrl Pts',(19.3149140521246,-1.28001029482722,126.729032652734));
#53937=CARTESIAN_POINT('Ctrl Pts',(19.6939106937694,-0.911595961366083,
126.761100859654));
#53938=CARTESIAN_POINT('Ctrl Pts',(19.8874259515692,-0.542567102648363,
126.786804946702));
#53939=CARTESIAN_POINT('Ctrl Pts',(20.0005163718621,-0.140992715157832,
126.812540864656));
#53940=CARTESIAN_POINT('Ctrl Pts',(19.9783846453537,0.389756960668105,126.844770741793));
#53941=CARTESIAN_POINT('Ctrl Pts',(19.6931858388931,0.961601125511805,126.883538256357));
#53942=CARTESIAN_POINT('Ctrl Pts',(19.1982285350886,1.36801288546453,126.922394650787));
#53943=CARTESIAN_POINT('Ctrl Pts',(18.5790486568211,1.53717771774434,126.961336325338));
#53944=CARTESIAN_POINT('Ctrl Pts',(17.9434620985098,1.43847641014473,127.00036001531));
#53945=CARTESIAN_POINT('Ctrl Pts',(17.4025305069054,1.08807198436899,127.039462191361));
#53946=CARTESIAN_POINT('Ctrl Pts',(17.0512361470141,0.54624806009065,127.078639381396));
#53947=CARTESIAN_POINT('Ctrl Pts',(16.9517077315689,-0.0929686702243292,
127.117888002863));
#53948=CARTESIAN_POINT('Ctrl Pts',(17.1222463114711,-0.718163540663969,
127.157204457133));
#53949=CARTESIAN_POINT('Ctrl Pts',(17.5339434625442,-1.21998914182436,127.19658508366));
#53950=CARTESIAN_POINT('Ctrl Pts',(18.1155967869452,-1.51033102531911,127.236026186941));
#53951=CARTESIAN_POINT('Ctrl Pts',(18.7660430040738,-1.53781009856395,127.275524023559));
#53952=CARTESIAN_POINT('Ctrl Pts',(19.3717918130506,-1.29689267540796,127.315074816817));
#53953=CARTESIAN_POINT('Ctrl Pts',(19.8268676166408,-0.828987338375049,
127.354674747443));
#53954=CARTESIAN_POINT('Ctrl Pts',(20.0513901487869,-0.215314584492064,
127.394319979104));
#53955=CARTESIAN_POINT('Ctrl Pts',(20.0056247885481,0.437220847592708,127.434006605569));
#53956=CARTESIAN_POINT('Ctrl Pts',(19.6970292834836,1.01469415427502,127.473730785989));
#53957=CARTESIAN_POINT('Ctrl Pts',(19.1790406081284,1.41609068632597,127.513488447827));
#53958=CARTESIAN_POINT('Ctrl Pts',(18.5418069825858,1.57101927908706,127.553275902336));
#53959=CARTESIAN_POINT('Ctrl Pts',(17.8964518857884,1.45207521426841,127.593088663885));
#53960=CARTESIAN_POINT('Ctrl Pts',(17.3556834232758,1.07970902742724,127.632923803203));
#53961=CARTESIAN_POINT('Ctrl Pts',(17.0140118977188,0.51868953019775,127.67277499967));
#53962=CARTESIAN_POINT('Ctrl Pts',(16.9312778521344,-0.133172545850757,
127.712643022715));
#53963=CARTESIAN_POINT('Ctrl Pts',(17.1220561745599,-0.76213953351389,127.752514978792));
#53964=CARTESIAN_POINT('Ctrl Pts',(17.5531223975555,-1.25833079809336,127.792401469815));
#53965=CARTESIAN_POINT('Ctrl Pts',(18.1494131749782,-1.53533610223328,127.832275370586));
#53966=CARTESIAN_POINT('Ctrl Pts',(18.8065933902536,-1.54432387682768,127.872171702413));
#53967=CARTESIAN_POINT('Ctrl Pts',(19.4100846272743,-1.28470708623083,127.912013923037));
#53968=CARTESIAN_POINT('Ctrl Pts',(19.8553100567167,-0.800375183111611,
127.951925887971));
#53969=CARTESIAN_POINT('Ctrl Pts',(20.0620620209392,-0.177762818146075,
127.991730529943));
#53970=CARTESIAN_POINT('Ctrl Pts',(20.0107296154146,0.365589401403285,128.024893024048));
#53971=CARTESIAN_POINT('Ctrl Pts',(19.8357953855363,0.761539243405002,128.051554711982));
#53972=CARTESIAN_POINT('Ctrl Pts',(19.6452972740319,1.02316795505993,128.071406241808));
#53973=CARTESIAN_POINT('Ctrl Pts',(19.407210271182,1.23882439608857,128.091206748466));
#53974=CARTESIAN_POINT('Ctrl Pts',(19.1325396712143,1.39988486175236,128.11111275206));
#53975=CARTESIAN_POINT('Ctrl Pts',(18.8296995883577,1.49940467423635,128.13113008268));
#53976=CARTESIAN_POINT('Ctrl Pts',(18.6146747329585,1.52230732399087,128.14430771094));
#53977=CARTESIAN_POINT('Ctrl Pts',(18.5048864505563,1.5232313661321,128.150806833261));
#53978=CARTESIAN_POINT('Ctrl Pts',(18.503702102348,1.49187608452152,112.989819674269));
#53979=CARTESIAN_POINT('Ctrl Pts',(18.3422645099611,1.49051733169978,112.999376273846));
#53980=CARTESIAN_POINT('Ctrl Pts',(18.1342705602965,1.45751807004094,113.012344390846));
#53981=CARTESIAN_POINT('Ctrl Pts',(17.8452633513425,1.34504789031967,113.031870507882));
#53982=CARTESIAN_POINT('Ctrl Pts',(17.6217687342541,1.21407386996056,113.048070801922));
#53983=CARTESIAN_POINT('Ctrl Pts',(17.3892912666459,1.00346179778602,113.067402258741));
#53984=CARTESIAN_POINT('Ctrl Pts',(17.2037216055837,0.748497642797482,113.086747828487));
#53985=CARTESIAN_POINT('Ctrl Pts',(17.0336365108725,0.363545641583294,113.112667763901));
#53986=CARTESIAN_POINT('Ctrl Pts',(16.9838992701375,-0.164270544608415,
113.144881746288));
#53987=CARTESIAN_POINT('Ctrl Pts',(17.184414544988,-0.767606361945544,113.183457189884));
#53988=CARTESIAN_POINT('Ctrl Pts',(17.6148373907955,-1.23555595231335,113.22202910865));
#53989=CARTESIAN_POINT('Ctrl Pts',(18.1969329026072,-1.48583931834946,113.260456741484));
#53990=CARTESIAN_POINT('Ctrl Pts',(18.8291856162506,-1.47700694025217,113.298838743469));
#53991=CARTESIAN_POINT('Ctrl Pts',(19.4015066537589,-1.21098811797121,113.33711466563));
#53992=CARTESIAN_POINT('Ctrl Pts',(19.8142041984067,-0.735692713550003,
113.375312027302));
#53993=CARTESIAN_POINT('Ctrl Pts',(19.9963547857532,-0.134671109049916,
113.413410387617));
#53994=CARTESIAN_POINT('Ctrl Pts',(19.917330891654,0.486756209803174,113.451417790248));
#53995=CARTESIAN_POINT('Ctrl Pts',(19.5922047575127,1.02032870198499,113.489324957824));
#53996=CARTESIAN_POINT('Ctrl Pts',(19.078874366281,1.37362515945365,113.52713270191));
#53997=CARTESIAN_POINT('Ctrl Pts',(18.4676774825549,1.48612836610816,113.564836685417));
#53998=CARTESIAN_POINT('Ctrl Pts',(17.8655356424751,1.33958682630473,113.602435135098));
#53999=CARTESIAN_POINT('Ctrl Pts',(17.3771760059416,0.960974919452283,113.639925184264));
#54000=CARTESIAN_POINT('Ctrl Pts',(17.0869162747918,0.417523224711967,113.677304608079));
#54001=CARTESIAN_POINT('Ctrl Pts',(17.0440749027117,-0.195226772711976,
113.71457097036));
#54002=CARTESIAN_POINT('Ctrl Pts',(17.2545974993079,-0.770247029667065,
113.751722040204));
#54003=CARTESIAN_POINT('Ctrl Pts',(17.6802710535475,-1.20773830122854,113.788755639842));
#54004=CARTESIAN_POINT('Ctrl Pts',(18.2456876606402,-1.43247667120123,113.825669614301));
#54005=CARTESIAN_POINT('Ctrl Pts',(18.8515648963708,-1.40675519342341,113.862462044251));
#54006=CARTESIAN_POINT('Ctrl Pts',(19.3922868480658,-1.13670944017846,113.899130819509));
#54007=CARTESIAN_POINT('Ctrl Pts',(19.7742257196495,-0.670960827012895,
113.935674250634));
#54008=CARTESIAN_POINT('Ctrl Pts',(19.9320734373548,-0.0918667144545759,
113.972090450819));
#54009=CARTESIAN_POINT('Ctrl Pts',(19.8399466317867,0.499115736790983,114.008377780349));
#54010=CARTESIAN_POINT('Ctrl Pts',(19.5156401611027,0.999094041612395,114.04453464138));
#54011=CARTESIAN_POINT('Ctrl Pts',(19.0172239827432,1.32186020605331,114.080559487712));
#54012=CARTESIAN_POINT('Ctrl Pts',(18.5300585493413,1.39736634472576,114.110469050883));
#54013=CARTESIAN_POINT('Ctrl Pts',(18.1483743883582,1.33483384505807,114.134329289553));
#54014=CARTESIAN_POINT('Ctrl Pts',(17.7885335979758,1.19494779695115,114.158144392525));
#54015=CARTESIAN_POINT('Ctrl Pts',(17.4104234910095,0.884458943355539,114.187828360597));
#54016=CARTESIAN_POINT('Ctrl Pts',(17.149528329175,0.360991850767247,114.223311911424));
#54017=CARTESIAN_POINT('Ctrl Pts',(17.1252556722554,-0.221068002059184,
114.258657303518));
#54018=CARTESIAN_POINT('Ctrl Pts',(17.3400117396107,-0.760164790222631,
114.293863534424));
#54019=CARTESIAN_POINT('Ctrl Pts',(17.7545646722328,-1.16290679171789,114.328929746419));
#54020=CARTESIAN_POINT('Ctrl Pts',(18.2952857435863,-1.36040896104986,114.363855170088));
#54021=CARTESIAN_POINT('Ctrl Pts',(18.8671866034673,-1.31998953853843,114.398639127519));
#54022=CARTESIAN_POINT('Ctrl Pts',(19.3706351176622,-1.05061228142374,114.433281034536));
#54023=CARTESIAN_POINT('Ctrl Pts',(19.7187089419615,-0.600950303027163,
114.467780414332));
#54024=CARTESIAN_POINT('Ctrl Pts',(19.8522062868052,-0.0506348125539401,
114.502136873029));
#54025=CARTESIAN_POINT('Ctrl Pts',(19.7497138563351,0.503904640082804,114.536350121929));
#54026=CARTESIAN_POINT('Ctrl Pts',(19.431010210694,0.966252463287474,114.570419973524));
#54027=CARTESIAN_POINT('Ctrl Pts',(18.9532691100971,1.25688267561954,114.604346322718));
#54028=CARTESIAN_POINT('Ctrl Pts',(18.4008406216132,1.32673243891578,114.638129178272));
#54029=CARTESIAN_POINT('Ctrl Pts',(17.8703226360875,1.16554167126788,114.671768634545));
#54030=CARTESIAN_POINT('Ctrl Pts',(17.4536942068799,0.803271481279279,114.705264891447));
#54031=CARTESIAN_POINT('Ctrl Pts',(17.2223629014042,0.304561077237039,114.738618237817));
#54032=CARTESIAN_POINT('Ctrl Pts',(17.2149314218132,-0.242783176148081,
114.77182907043));
#54033=CARTESIAN_POINT('Ctrl Pts',(17.4307882423904,-0.743289781556822,
114.804897864875));
#54034=CARTESIAN_POINT('Ctrl Pts',(17.8305161533526,-1.11037437400687,114.837825225747));
#54035=CARTESIAN_POINT('Ctrl Pts',(18.3431414371818,-1.28149381786692,114.870611792906));
#54036=CARTESIAN_POINT('Ctrl Pts',(18.7893553523156,-1.23727626130552,114.897817313457));
#54037=CARTESIAN_POINT('Ctrl Pts',(19.1112128056895,-1.09554793991547,114.919512124933));
#54038=CARTESIAN_POINT('Ctrl Pts',(19.396175350928,-0.890697859688692,114.941160733749));
#54039=CARTESIAN_POINT('Ctrl Pts',(19.6584018411182,-0.531669188250831,
114.968135177746));
#54040=CARTESIAN_POINT('Ctrl Pts',(19.76908647096,-0.0120339067964489,115.000367371872));
#54041=CARTESIAN_POINT('Ctrl Pts',(19.6583942300963,0.505266606576981,115.032463636213));
#54042=CARTESIAN_POINT('Ctrl Pts',(19.3473557859062,0.93046495841335,115.064425180333));
#54043=CARTESIAN_POINT('Ctrl Pts',(18.8916950780005,1.19043640343731,115.096253363284));
#54044=CARTESIAN_POINT('Ctrl Pts',(18.3717570032792,1.24142340224108,115.127949584784));
#54045=CARTESIAN_POINT('Ctrl Pts',(17.8783677920246,1.07626545587742,115.15951539726));
#54046=CARTESIAN_POINT('Ctrl Pts',(17.4970559877627,0.725456658754698,115.190952339247));
#54047=CARTESIAN_POINT('Ctrl Pts',(17.2930596087315,0.251374726199106,115.222262219888));
#54048=CARTESIAN_POINT('Ctrl Pts',(17.2997368545718,-0.205413166433051,
115.249981653063));
#54049=CARTESIAN_POINT('Ctrl Pts',(17.4404319127292,-0.573042786265209,
115.274156363673));
#54050=CARTESIAN_POINT('Ctrl Pts',(17.592066785102,-0.774671677260083,115.289656127754));
#54051=CARTESIAN_POINT('Ctrl Pts',(17.7139015205345,-0.888101474402246,
115.29997296064));
#54052=CARTESIAN_POINT('Ctrl Pts',(17.7785097005419,-0.940424780251118,
115.305127839623));
#54053=CARTESIAN_POINT('Ctrl Pts',(17.8466470444457,-0.98801547265171,115.310279486813));
#54054=CARTESIAN_POINT('Ctrl Pts',(17.989070409944,-1.07344813179845,115.320575730976));
#54055=CARTESIAN_POINT('Ctrl Pts',(18.2236591817274,-1.16292300047207,115.335996045863));
#54056=CARTESIAN_POINT('Ctrl Pts',(18.5563155957279,-1.19093988306076,115.3565030506));
#54057=CARTESIAN_POINT('Ctrl Pts',(18.8830047845655,-1.12589266484945,115.376958878633));
#54058=CARTESIAN_POINT('Ctrl Pts',(19.1780050081399,-0.9733951898541,115.397362889332));
#54059=CARTESIAN_POINT('Ctrl Pts',(19.4189487015537,-0.745659756110988,
115.417716885332));
#54060=CARTESIAN_POINT('Ctrl Pts',(19.586513319755,-0.460981781034244,115.438020595246));
#54061=CARTESIAN_POINT('Ctrl Pts',(19.6971134584733,-0.0350499051287504,
115.465026998031));
#54062=CARTESIAN_POINT('Ctrl Pts',(19.6213835081677,0.409308743056556,115.491936476127));
#54063=CARTESIAN_POINT('Ctrl Pts',(19.4081815400465,0.726708802320049,115.515399793606));
#54064=CARTESIAN_POINT('Ctrl Pts',(19.2533820709519,0.877517364647426,115.528784631642));
#54065=CARTESIAN_POINT('Ctrl Pts',(19.0787709601167,1.00501199378957,115.542153884178));
#54066=CARTESIAN_POINT('Ctrl Pts',(18.9053740303453,1.0826747173383,115.553831967145));
#54067=CARTESIAN_POINT('Ctrl Pts',(18.7488682526583,1.1217999761029,115.56382821947));
#54068=CARTESIAN_POINT('Ctrl Pts',(18.6695549654301,1.13586113853869,115.568823416288));
#54069=CARTESIAN_POINT('Ctrl Pts',(18.6028029629378,1.14293032142239,115.57298384464));
#54070=CARTESIAN_POINT('Ctrl Pts',(18.5492301296799,1.14569963267631,115.576310658733));
#54071=CARTESIAN_POINT('Ctrl Pts',(18.3318189962245,1.14985398886929,115.589799489503));
#54072=CARTESIAN_POINT('Ctrl Pts',(17.93807646621,1.04913122524392,115.61423125823));
#54073=CARTESIAN_POINT('Ctrl Pts',(17.6038273489929,0.738872428658555,115.641663000481));
#54074=CARTESIAN_POINT('Ctrl Pts',(17.4553862402826,0.459584671101082,115.661208854169));
#54075=CARTESIAN_POINT('Ctrl Pts',(17.404909185234,0.310016726484566,115.670970109025));
#54076=CARTESIAN_POINT('Ctrl Pts',(17.3801146498094,0.186574169585243,115.67877223044));
#54077=CARTESIAN_POINT('Ctrl Pts',(17.3505224034491,-0.0633246010535821,
115.694366612529));
#54078=CARTESIAN_POINT('Ctrl Pts',(17.4237971555624,-0.477375899585048,
115.719655510759));
#54079=CARTESIAN_POINT('Ctrl Pts',(17.7858376869751,-0.931108485774203,
115.754551104908));
#54080=CARTESIAN_POINT('Ctrl Pts',(18.2745211046451,-1.13667010750685,115.786433819311));
#54081=CARTESIAN_POINT('Ctrl Pts',(18.7484690587498,-1.11846305743127,115.81533834407));
#54082=CARTESIAN_POINT('Ctrl Pts',(19.1386709996485,-0.948289610488192,
115.84129311261));
#54083=CARTESIAN_POINT('Ctrl Pts',(19.4390996247751,-0.647682388358762,
115.867191006533));
#54084=CARTESIAN_POINT('Ctrl Pts',(19.5802476090257,-0.323886197170617,
115.888726654306));
#54085=CARTESIAN_POINT('Ctrl Pts',(19.6164608276318,-0.0476515215733575,
115.905929464203));
#54086=CARTESIAN_POINT('Ctrl Pts',(19.6048021299846,0.160672150153393,115.918818002215));
#54087=CARTESIAN_POINT('Ctrl Pts',(19.5629552356086,0.329344380429827,115.92954886288));
#54088=CARTESIAN_POINT('Ctrl Pts',(19.5111419167609,0.457709038523884,115.938127090231));
#54089=CARTESIAN_POINT('Ctrl Pts',(19.4159798157258,0.642183917490576,115.950988089536));
#54090=CARTESIAN_POINT('Ctrl Pts',(19.2097310734986,0.881763831274916,115.970258025515));
#54091=CARTESIAN_POINT('Ctrl Pts',(18.8376888372652,1.07831902356411,115.995905289709));
#54092=CARTESIAN_POINT('Ctrl Pts',(18.420246143728,1.12529003433152,116.021509895766));
#54093=CARTESIAN_POINT('Ctrl Pts',(18.1164398186431,1.04383241287061,116.040683067193));
#54094=CARTESIAN_POINT('Ctrl Pts',(17.935182926549,0.945722916711651,116.053453203537));
#54095=CARTESIAN_POINT('Ctrl Pts',(17.8209867836636,0.869446264038907,116.061963256023));
#54096=CARTESIAN_POINT('Ctrl Pts',(17.6412091504734,0.708850503681455,116.076848878371));
#54097=CARTESIAN_POINT('Ctrl Pts',(17.5206165699508,0.517177860963483,116.090655859422));
#54098=CARTESIAN_POINT('Ctrl Pts',(17.4619719522485,0.356352158450434,116.101269186923));
#54099=CARTESIAN_POINT('Ctrl Pts',(17.4465783138213,0.307388824240754,116.104452776497));
#54100=CARTESIAN_POINT('Ctrl Pts',(17.4335399348317,0.257734727890675,116.107635795408));
#54101=CARTESIAN_POINT('Ctrl Pts',(17.4228231536783,0.207551498411839,116.110818346632));
#54102=CARTESIAN_POINT('Ctrl Pts',(17.4144491679001,0.156922359184113,116.114000351126));
#54103=CARTESIAN_POINT('Ctrl Pts',(17.4065086961841,0.0889837600333896,
116.118242356133));
#54104=CARTESIAN_POINT('Ctrl Pts',(17.3975764169991,-0.0990303571900397,
116.129904811033));
#54105=CARTESIAN_POINT('Ctrl Pts',(17.4557897410273,-0.406430268110572,
116.148975549028));
#54106=CARTESIAN_POINT('Ctrl Pts',(17.6775193909147,-0.759239865060753,
116.174374346993));
#54107=CARTESIAN_POINT('Ctrl Pts',(18.0124729574942,-1.00640471012008,116.199748244809));
#54108=CARTESIAN_POINT('Ctrl Pts',(18.4142334421369,-1.11401582947692,116.225098996324));
#54109=CARTESIAN_POINT('Ctrl Pts',(18.8271625055921,-1.0674620377526,116.250429703679));
#54110=CARTESIAN_POINT('Ctrl Pts',(19.1943590995122,-0.873386967180604,
116.275742455032));
#54111=CARTESIAN_POINT('Ctrl Pts',(19.4048227403936,-0.628698108618376,
116.295418901538));
#54112=CARTESIAN_POINT('Ctrl Pts',(19.5057918819382,-0.425410293547205,
116.309468193535));
#54113=CARTESIAN_POINT('Ctrl Pts',(19.5656339219958,-0.254098208903609,
116.320706689353));
#54114=CARTESIAN_POINT('Ctrl Pts',(19.6137410150594,0.0618235256489764,
116.340368827849));
#54115=CARTESIAN_POINT('Ctrl Pts',(19.5099378325633,0.517016389985175,116.368448290932));
#54116=CARTESIAN_POINT('Ctrl Pts',(19.1391182957214,0.937107132493867,116.40213348579));
#54117=CARTESIAN_POINT('Ctrl Pts',(18.6128054716757,1.12867451927067,116.435815336319));
#54118=CARTESIAN_POINT('Ctrl Pts',(18.058785719797,1.04521466627339,116.469499752536));
#54119=CARTESIAN_POINT('Ctrl Pts',(17.6772819616439,0.756169197308419,116.498279566654));
#54120=CARTESIAN_POINT('Ctrl Pts',(17.4803749568857,0.421072765008975,116.522153929673));
#54121=CARTESIAN_POINT('Ctrl Pts',(17.3766797417797,0.0225849405462479,
116.547440772492));
#54122=CARTESIAN_POINT('Ctrl Pts',(17.465295524311,-0.500202217111396,116.579066566679));
#54123=CARTESIAN_POINT('Ctrl Pts',(17.889792472491,-0.975335446352908,116.617054365501));
#54124=CARTESIAN_POINT('Ctrl Pts',(18.502637561406,-1.15197604515318,116.655087623956));
#54125=CARTESIAN_POINT('Ctrl Pts',(19.1163786805987,-0.975332764938637,
116.693175009599));
#54126=CARTESIAN_POINT('Ctrl Pts',(19.5429506803428,-0.49832909128163,116.73132532745));
#54127=CARTESIAN_POINT('Ctrl Pts',(19.6323015217028,0.0281297749259298,
116.763176460355));
#54128=CARTESIAN_POINT('Ctrl Pts',(19.5277627412065,0.430370844822526,116.788697635011));
#54129=CARTESIAN_POINT('Ctrl Pts',(19.369679999767,0.6992353885053,116.807859099239));
#54130=CARTESIAN_POINT('Ctrl Pts',(19.1424632389321,0.913533103672042,116.827043111286));
#54131=CARTESIAN_POINT('Ctrl Pts',(18.772367790744,1.10567953941629,116.852652017112));
#54132=CARTESIAN_POINT('Ctrl Pts',(18.2355341126458,1.13621815304612,116.884723808745));
#54133=CARTESIAN_POINT('Ctrl Pts',(17.6689198164127,0.823295827742766,116.923314310429));
#54134=CARTESIAN_POINT('Ctrl Pts',(17.3547647490283,0.255422345016107,116.962017521189));
#54135=CARTESIAN_POINT('Ctrl Pts',(17.3909543071043,-0.394665908212814,
117.00084115596));
#54136=CARTESIAN_POINT('Ctrl Pts',(17.7687099122216,-0.927569838505474,
117.039793042541));
#54137=CARTESIAN_POINT('Ctrl Pts',(18.3741755754646,-1.17872989356506,117.078880711992));
#54138=CARTESIAN_POINT('Ctrl Pts',(19.0228384514425,-1.06886607959656,117.118111607769));
#54139=CARTESIAN_POINT('Ctrl Pts',(19.5155163757392,-0.629071317918103,
117.15749296697));
#54140=CARTESIAN_POINT('Ctrl Pts',(19.6994420911959,0.00797209925389068,
117.197031859252));
#54141=CARTESIAN_POINT('Ctrl Pts',(19.515500647011,0.647878257780649,117.23673514959));
#54142=CARTESIAN_POINT('Ctrl Pts',(19.0171733063539,1.09376372921043,117.27660952184));
#54143=CARTESIAN_POINT('Ctrl Pts',(18.3550699462677,1.20669326786917,117.316661446212));
#54144=CARTESIAN_POINT('Ctrl Pts',(17.731513825934,0.948886060096873,117.356897172836));
#54145=CARTESIAN_POINT('Ctrl Pts',(17.3388450878967,0.396256579223924,117.39732273553));
#54146=CARTESIAN_POINT('Ctrl Pts',(17.3001759338416,-0.283860165024669,
117.437943945886));
#54147=CARTESIAN_POINT('Ctrl Pts',(17.6309104423397,-0.883255559054568,
117.478766367029));
#54148=CARTESIAN_POINT('Ctrl Pts',(18.2328525117844,-1.21651929036585,117.519795325694));
#54149=CARTESIAN_POINT('Ctrl Pts',(18.9234234044072,-1.17823144343809,117.561035895459));
#54150=CARTESIAN_POINT('Ctrl Pts',(19.4906656002749,-0.776372273993139,
117.602492914177));
#54151=CARTESIAN_POINT('Ctrl Pts',(19.7587364840262,-0.13078846109893,117.644170910344));
#54152=CARTESIAN_POINT('Ctrl Pts',(19.6608941213843,0.446513363382881,117.679090346474));
#54153=CARTESIAN_POINT('Ctrl Pts',(19.4063763506229,0.825732225186209,117.707140502678));
#54154=CARTESIAN_POINT('Ctrl Pts',(19.0572403859771,1.12201758553148,117.735267815038));
#54155=CARTESIAN_POINT('Ctrl Pts',(18.4885802358337,1.2865381867526,117.770572480421));
#54156=CARTESIAN_POINT('Ctrl Pts',(17.801838273725,1.08919683440124,117.813174713138));
#54157=CARTESIAN_POINT('Ctrl Pts',(17.3227121836494,0.553921475501694,117.856016594786));
#54158=CARTESIAN_POINT('Ctrl Pts',(17.2010966707053,-0.158326099518395,
117.899101101152));
#54159=CARTESIAN_POINT('Ctrl Pts',(17.4786390279773,-0.829851682392695,
117.942430781901));
#54160=CARTESIAN_POINT('Ctrl Pts',(18.0742946344301,-1.25323173475652,117.986007964128));
#54161=CARTESIAN_POINT('Ctrl Pts',(18.8080726935777,-1.29501226255686,118.029834639599));
#54162=CARTESIAN_POINT('Ctrl Pts',(19.4553159300046,-0.938010475541138,
118.073912516848));
#54163=CARTESIAN_POINT('Ctrl Pts',(19.8154307819553,-0.287585555372444,
118.118242990085));
#54164=CARTESIAN_POINT('Ctrl Pts',(19.7741366820081,0.458836644666698,118.16282715909));
#54165=CARTESIAN_POINT('Ctrl Pts',(19.3394435327949,1.07263691503397,118.207665807633));
#54166=CARTESIAN_POINT('Ctrl Pts',(18.7575552739269,1.31396042818269,118.24524382035));
#54167=CARTESIAN_POINT('Ctrl Pts',(18.2660136694013,1.29932960507879,118.275433796398));
#54168=CARTESIAN_POINT('Ctrl Pts',(17.9138511199113,1.18752313651639,118.298140055659));
#54169=CARTESIAN_POINT('Ctrl Pts',(17.6055358088652,0.98141598551866,118.320910047554));
#54170=CARTESIAN_POINT('Ctrl Pts',(17.3656586969673,0.69755141465935,118.343743757908));
#54171=CARTESIAN_POINT('Ctrl Pts',(17.2133153242065,0.357232692236245,118.366641084558));
#54172=CARTESIAN_POINT('Ctrl Pts',(17.1610033132225,-0.0128449924121692,
118.389601986026));
#54173=CARTESIAN_POINT('Ctrl Pts',(17.2133047298867,-0.384104530010112,
118.412626315514));
#54174=CARTESIAN_POINT('Ctrl Pts',(17.3412396152671,-0.669931994924582,
118.431866032995));
#54175=CARTESIAN_POINT('Ctrl Pts',(17.4883028212069,-0.871293451744624,
118.447289433679));
#54176=CARTESIAN_POINT('Ctrl Pts',(17.6623643786738,-1.04999788798832,118.46273378822));
#54177=CARTESIAN_POINT('Ctrl Pts',(18.0285864515854,-1.29592018799767,118.489816685333));
#54178=CARTESIAN_POINT('Ctrl Pts',(18.6703881436677,-1.40571108227618,118.528663586766));
#54179=CARTESIAN_POINT('Ctrl Pts',(19.3970876386868,-1.1053408950482,118.575529603312));
#54180=CARTESIAN_POINT('Ctrl Pts',(19.7780709579159,-0.568789994131528,
118.614791183341));
#54181=CARTESIAN_POINT('Ctrl Pts',(19.8649536567208,-0.127762187171968,
118.642381544121));
#54182=CARTESIAN_POINT('Ctrl Pts',(19.8615540247625,0.127284981139844,118.658178190531));
#54183=CARTESIAN_POINT('Ctrl Pts',(19.8223396408192,0.380112246085207,118.673994886313));
#54184=CARTESIAN_POINT('Ctrl Pts',(19.7071782081534,0.681042071721743,118.693803936495));
#54185=CARTESIAN_POINT('Ctrl Pts',(19.3968645270032,1.09527626728677,118.725578754282));
#54186=CARTESIAN_POINT('Ctrl Pts',(18.8122225330156,1.41911251137611,118.76544746249));
#54187=CARTESIAN_POINT('Ctrl Pts',(18.007042177151,1.3744471680488,118.813526770773));
#54188=CARTESIAN_POINT('Ctrl Pts',(17.3459220719172,0.90601479701624,118.86183971331));
#54189=CARTESIAN_POINT('Ctrl Pts',(17.0861041214154,0.279551870891405,118.902291882144));
#54190=CARTESIAN_POINT('Ctrl Pts',(17.1019462138081,-0.24916096313258,118.93476676582));
#54191=CARTESIAN_POINT('Ctrl Pts',(17.2019719756035,-0.564646975838234,
118.955109853082));
#54192=CARTESIAN_POINT('Ctrl Pts',(17.3166223801635,-0.764853864695036,
118.96937458627));
#54193=CARTESIAN_POINT('Ctrl Pts',(17.3934033772786,-0.871630377869911,
118.977532651056));
#54194=CARTESIAN_POINT('Ctrl Pts',(17.477703283774,-0.972842734233704,118.985695303595));
#54195=CARTESIAN_POINT('Ctrl Pts',(17.5959908064179,-1.08787346995914,118.995906958726));
#54196=CARTESIAN_POINT('Ctrl Pts',(17.80940624637,-1.24391112239919,119.012264402582));
#54197=CARTESIAN_POINT('Ctrl Pts',(18.1137047432836,-1.38016569420815,119.032744595313));
#54198=CARTESIAN_POINT('Ctrl Pts',(18.5107756099825,-1.43627485577155,119.057374894024));
#54199=CARTESIAN_POINT('Ctrl Pts',(18.9086887725081,-1.38015979004093,119.082057931785));
#54200=CARTESIAN_POINT('Ctrl Pts',(19.2763086985662,-1.21572919182316,119.106793694273));
#54201=CARTESIAN_POINT('Ctrl Pts',(19.5846796723198,-0.955406316030372,
119.131580970565));
#54202=CARTESIAN_POINT('Ctrl Pts',(19.809392321284,-0.619204248974561,119.15641978872));
#54203=CARTESIAN_POINT('Ctrl Pts',(19.9325091524558,-0.233138195850857,
119.181308555028));
#54204=CARTESIAN_POINT('Ctrl Pts',(19.9439344589339,0.172710845827226,119.206247801915));
#54205=CARTESIAN_POINT('Ctrl Pts',(19.859333630366,0.501021221890519,119.227070700593));
#54206=CARTESIAN_POINT('Ctrl Pts',(19.7388322341717,0.742192001820556,119.243753783559));
#54207=CARTESIAN_POINT('Ctrl Pts',(19.5477513775307,1.02020898738615,119.264627237985));
#54208=CARTESIAN_POINT('Ctrl Pts',(19.1748525603661,1.32647007207184,119.293905797606));
#54209=CARTESIAN_POINT('Ctrl Pts',(18.5746327535004,1.49048570425054,119.33165434782));
#54210=CARTESIAN_POINT('Ctrl Pts',(17.9581548867158,1.3947907252162,119.369505012355));
#54211=CARTESIAN_POINT('Ctrl Pts',(17.433136470404,1.05474858337055,119.407455104193));
#54212=CARTESIAN_POINT('Ctrl Pts',(17.0919383518421,0.528571566609064,119.445501954772));
#54213=CARTESIAN_POINT('Ctrl Pts',(16.9951890882095,-0.0925769725045345,
119.48364264785));
#54214=CARTESIAN_POINT('Ctrl Pts',(17.1609540266251,-0.700571381474122,
119.52187456006));
#54215=CARTESIAN_POINT('Ctrl Pts',(17.4948116280989,-1.10745799563107,119.553807683116));
#54216=CARTESIAN_POINT('Ctrl Pts',(17.8447023681615,-1.33030493897242,119.579397106812));
#54217=CARTESIAN_POINT('Ctrl Pts',(18.2335472691901,-1.47606655473774,119.605014075801));
#54218=CARTESIAN_POINT('Ctrl Pts',(18.7616932453127,-1.49849508652994,119.637086847695));
#54219=CARTESIAN_POINT('Ctrl Pts',(19.3523944101162,-1.26357563907783,119.675653098896));
#54220=CARTESIAN_POINT('Ctrl Pts',(19.796491636114,-0.807043559144156,119.714295292846));
#54221=CARTESIAN_POINT('Ctrl Pts',(20.0157970505624,-0.207778260258124,
119.753010147915));
#54222=CARTESIAN_POINT('Ctrl Pts',(19.9711184784079,0.429920342496358,119.791794464769));
#54223=CARTESIAN_POINT('Ctrl Pts',(19.6693616238384,0.994715766881195,119.830644916317));
#54224=CARTESIAN_POINT('Ctrl Pts',(19.1623979919676,1.38763506879075,119.869558191545));
#54225=CARTESIAN_POINT('Ctrl Pts',(18.5382405530733,1.53942785144906,119.908530869871));
#54226=CARTESIAN_POINT('Ctrl Pts',(17.9055587368166,1.42291065228989,119.947559593151));
#54227=CARTESIAN_POINT('Ctrl Pts',(17.4634685402937,1.11845970679053,119.980127250936));
#54228=CARTESIAN_POINT('Ctrl Pts',(17.2072047563733,0.782220751904666,120.006205932695));
#54229=CARTESIAN_POINT('Ctrl Pts',(17.0259624642235,0.400010121518591,120.032300468687));
#54230=CARTESIAN_POINT('Ctrl Pts',(16.9581031072095,-0.133786264742428,
120.064946918911));
#54231=CARTESIAN_POINT('Ctrl Pts',(17.1456963710106,-0.752388312245989,
120.104164686953));
#54232=CARTESIAN_POINT('Ctrl Pts',(17.5699893730723,-1.2408823945971,120.143420804628));
#54233=CARTESIAN_POINT('Ctrl Pts',(18.1573322171588,-1.51371900905838,120.182711703032));
#54234=CARTESIAN_POINT('Ctrl Pts',(18.8053948529502,-1.52285657093314,120.222033701872));
#54235=CARTESIAN_POINT('Ctrl Pts',(19.4010838377385,-1.26631875735931,120.261383165299));
#54236=CARTESIAN_POINT('Ctrl Pts',(19.8402963026219,-0.788554594843257,
120.30075640158));
#54237=CARTESIAN_POINT('Ctrl Pts',(20.0461617582727,-0.172750782040334,
120.340149724409));
#54238=CARTESIAN_POINT('Ctrl Pts',(19.9825174326225,0.473697806244577,120.379559422821));
#54239=CARTESIAN_POINT('Ctrl Pts',(19.6602768883809,1.03794772706267,120.4189817794));
#54240=CARTESIAN_POINT('Ctrl Pts',(19.1355536795428,1.42145008827222,120.45841306485));
#54241=CARTESIAN_POINT('Ctrl Pts',(18.4998707433376,1.55719588396314,120.497849545716));
#54242=CARTESIAN_POINT('Ctrl Pts',(17.864163205303,1.42145001008791,120.537287485317));
#54243=CARTESIAN_POINT('Ctrl Pts',(17.3393787989982,1.03790924248084,120.57672314656));
#54244=CARTESIAN_POINT('Ctrl Pts',(17.017074206874,0.473557355218691,120.616152792451));
#54245=CARTESIAN_POINT('Ctrl Pts',(16.953408471598,-0.173057796539594,120.655572689844));
#54246=CARTESIAN_POINT('Ctrl Pts',(17.1593374262179,-0.789068501312153,
120.694979112502));
#54247=CARTESIAN_POINT('Ctrl Pts',(17.5987249550259,-1.26702928001241,120.734368344241));
#54248=CARTESIAN_POINT('Ctrl Pts',(18.1946971056568,-1.52369644517567,120.773736681215));
#54249=CARTESIAN_POINT('Ctrl Pts',(18.8431194373237,-1.51455574960213,120.813080431625));
#54250=CARTESIAN_POINT('Ctrl Pts',(19.4308298620431,-1.24155842999136,120.852395921515));
#54251=CARTESIAN_POINT('Ctrl Pts',(19.8554281123154,-0.752716870273097,
120.891679493858));
#54252=CARTESIAN_POINT('Ctrl Pts',(20.0431536703053,-0.133645042672799,
120.930927518414));
#54253=CARTESIAN_POINT('Ctrl Pts',(19.9617251011364,0.507468436214418,120.970136382216));
#54254=CARTESIAN_POINT('Ctrl Pts',(19.6259005154625,1.05880076011582,121.009302510876));
#54255=CARTESIAN_POINT('Ctrl Pts',(19.0948017776786,1.42444673699063,121.048422333788));
#54256=CARTESIAN_POINT('Ctrl Pts',(18.4614843836788,1.5411183959411,121.087492358667));
#54257=CARTESIAN_POINT('Ctrl Pts',(17.8366037551925,1.38915003243965,121.12650904033));
#54258=CARTESIAN_POINT('Ctrl Pts',(17.3290377823205,0.995758540539347,121.165469034314));
#54259=CARTESIAN_POINT('Ctrl Pts',(17.0268896562641,0.430268183212111,121.204368725407));
#54260=CARTESIAN_POINT('Ctrl Pts',(16.9821482492727,-0.208328248111488,
121.243205126464));
#54261=CARTESIAN_POINT('Ctrl Pts',(17.1468513998485,-0.658338107284023,
121.272281854363));
#54262=CARTESIAN_POINT('Ctrl Pts',(17.3270527013809,-0.913793541276511,
121.2916449787));
#54263=CARTESIAN_POINT('Ctrl Pts',(17.46418185158,-1.0705239622011,121.304547220258));
#54264=CARTESIAN_POINT('Ctrl Pts',(17.7451790402857,-1.30479380949971,121.327111265409));
#54265=CARTESIAN_POINT('Ctrl Pts',(18.2380695380599,-1.50090249377063,121.359299336153));
#54266=CARTESIAN_POINT('Ctrl Pts',(18.872952337819,-1.47399830138094,121.397848602223));
#54267=CARTESIAN_POINT('Ctrl Pts',(19.4402270507624,-1.19079335758157,121.43631807797));
#54268=CARTESIAN_POINT('Ctrl Pts',(19.8415184192534,-0.701595659415583,
121.47470479001));
#54269=CARTESIAN_POINT('Ctrl Pts',(20.0076038779129,-0.0925460055625223,
121.513005657936));
#54270=CARTESIAN_POINT('Ctrl Pts',(19.9106710958716,0.529786710311653,121.551217745528));
#54271=CARTESIAN_POINT('Ctrl Pts',(19.5688165951267,1.05697212875173,121.589338130621));
#54272=CARTESIAN_POINT('Ctrl Pts',(19.0427596201426,1.39770166829743,121.62736397679));
#54273=CARTESIAN_POINT('Ctrl Pts',(18.4249973670875,1.4935958090029,121.665292499313));
#54274=CARTESIAN_POINT('Ctrl Pts',(17.8235396206654,1.32923563625104,121.703120986417));
#54275=CARTESIAN_POINT('Ctrl Pts',(17.3429817574642,0.934618133209399,121.740846791978));
#54276=CARTESIAN_POINT('Ctrl Pts',(17.0662946299328,0.379687410860908,121.778467339518));
#54277=CARTESIAN_POINT('Ctrl Pts',(17.0404764052604,-0.238080819165208,
121.815980124477));
#54278=CARTESIAN_POINT('Ctrl Pts',(17.2685662738785,-0.810825747926414,
121.853382712339));
#54279=CARTESIAN_POINT('Ctrl Pts',(17.7093700547578,-1.23915893357272,121.890672750573));
#54280=CARTESIAN_POINT('Ctrl Pts',(18.2849022360115,-1.44943799786466,121.927847950456));
#54281=CARTESIAN_POINT('Ctrl Pts',(18.8942013046416,-1.4064333916413,121.964906125628));
#54282=CARTESIAN_POINT('Ctrl Pts',(19.4310600024741,-1.11924200067342,122.001845121409));
#54283=CARTESIAN_POINT('Ctrl Pts',(19.8025684779115,-0.639390170128088,
122.038662952609));
#54284=CARTESIAN_POINT('Ctrl Pts',(19.9451989003155,-0.051637223723163,
122.075357550695));
#54285=CARTESIAN_POINT('Ctrl Pts',(19.8356891395559,0.541102670830277,122.111927198002));
#54286=CARTESIAN_POINT('Ctrl Pts',(19.4948233406496,1.03568092690009,122.1483699589));
#54287=CARTESIAN_POINT('Ctrl Pts',(18.9834812980339,1.34680051480277,122.184684197437));
#54288=CARTESIAN_POINT('Ctrl Pts',(18.3917927004701,1.42165473989535,122.220868285127));
#54289=CARTESIAN_POINT('Ctrl Pts',(17.823211725378,1.24893790158853,122.256920676789));
#54290=CARTESIAN_POINT('Ctrl Pts',(17.376424697306,0.860487459682125,122.292839947562));
#54291=CARTESIAN_POINT('Ctrl Pts',(17.1282004735361,0.325438701500939,122.328624743665));
#54292=CARTESIAN_POINT('Ctrl Pts',(17.1201969314303,-0.262093773310703,
122.364273793238));
#54293=CARTESIAN_POINT('Ctrl Pts',(17.3519746550279,-0.799579240414161,
122.39978595058));
#54294=CARTESIAN_POINT('Ctrl Pts',(17.7813972457046,-1.19397853058097,122.435160118652));
#54295=CARTESIAN_POINT('Ctrl Pts',(18.3322852669273,-1.3778564057377,122.470395332238));
#54296=CARTESIAN_POINT('Ctrl Pts',(18.9079366722081,-1.32091501639784,122.50549070087));
#54297=CARTESIAN_POINT('Ctrl Pts',(19.408110174119,-1.03496607388862,122.540445426145));
#54298=CARTESIAN_POINT('Ctrl Pts',(19.7464914273704,-0.571545265474727,
122.575258824259));
#54299=CARTESIAN_POINT('Ctrl Pts',(19.8655874804599,-0.0126175132191439,
122.609930280511));
#54300=CARTESIAN_POINT('Ctrl Pts',(19.7464983590342,0.543905007067228,122.644459305606));
#54301=CARTESIAN_POINT('Ctrl Pts',(19.4118682240342,1.00135709037548,122.678845474284));
#54302=CARTESIAN_POINT('Ctrl Pts',(18.9216435947912,1.28105760502164,122.713088499641));
#54303=CARTESIAN_POINT('Ctrl Pts',(18.3622701529655,1.33589566146183,122.747188144647));
#54304=CARTESIAN_POINT('Ctrl Pts',(17.8315352721831,1.15824493019145,122.781144309059));
#54305=CARTESIAN_POINT('Ctrl Pts',(17.4213882328109,0.780879052378252,122.814956965966));
#54306=CARTESIAN_POINT('Ctrl Pts',(17.2020806893666,0.271141102260439,122.848626198319));
#54307=CARTESIAN_POINT('Ctrl Pts',(17.209183784722,-0.220082502602327,122.878427070648));
#54308=CARTESIAN_POINT('Ctrl Pts',(17.3605649792115,-0.61497008299745,122.904410163103));
#54309=CARTESIAN_POINT('Ctrl Pts',(17.6498776696226,-1.00079015878131,122.934020544251));
#54310=CARTESIAN_POINT('Ctrl Pts',(18.1907942060837,-1.29941447755314,122.97087522974));
#54311=CARTESIAN_POINT('Ctrl Pts',(18.9271744385363,-1.25743252782069,123.014848789226));
#54312=CARTESIAN_POINT('Ctrl Pts',(19.5247563273938,-0.832644021409292,
123.058571824615));
#54313=CARTESIAN_POINT('Ctrl Pts',(19.80324675155,-0.158914336827329,123.102046150492));
#54314=CARTESIAN_POINT('Ctrl Pts',(19.681237596879,0.555806024003187,123.145273911019));
#54315=CARTESIAN_POINT('Ctrl Pts',(19.2805996484641,1.00313565776361,123.181093571345));
#54316=CARTESIAN_POINT('Ctrl Pts',(18.8560336820417,1.19200190630298,123.209628597104));
#54317=CARTESIAN_POINT('Ctrl Pts',(18.5248663207615,1.2391334244017,123.230179459196));
#54318=CARTESIAN_POINT('Ctrl Pts',(18.2071745052378,1.19886853894009,123.249887786568));
#54319=CARTESIAN_POINT('Ctrl Pts',(17.826353246682,1.05001593167474,123.275052032664));
#54320=CARTESIAN_POINT('Ctrl Pts',(17.4444385755585,0.695322823220176,123.306391013143));
#54321=CARTESIAN_POINT('Ctrl Pts',(17.2796430128223,0.203571410228621,123.337577098318));
#54322=CARTESIAN_POINT('Ctrl Pts',(17.3005198205283,-0.199770590504172,
123.362435390156));
#54323=CARTESIAN_POINT('Ctrl Pts',(17.4186728528587,-0.584917553785751,
123.38723397063));
#54324=CARTESIAN_POINT('Ctrl Pts',(17.7391439823498,-0.986504330030103,
123.418120743375));
#54325=CARTESIAN_POINT('Ctrl Pts',(18.2575183309786,-1.204406059504,123.451935767405));
#54326=CARTESIAN_POINT('Ctrl Pts',(18.7594894991427,-1.18507959151576,123.482551288236));
#54327=CARTESIAN_POINT('Ctrl Pts',(19.1723107596392,-1.00498843556934,123.510009958442));
#54328=CARTESIAN_POINT('Ctrl Pts',(19.4896744215185,-0.687329613632877,
123.537374781882));
#54329=CARTESIAN_POINT('Ctrl Pts',(19.6684610038165,-0.277235805793136,
123.564647175546));
#54330=CARTESIAN_POINT('Ctrl Pts',(19.6850058219944,0.168442379631604,123.591828854406));
#54331=CARTESIAN_POINT('Ctrl Pts',(19.5380627655275,0.587887775867897,123.618921130316));
#54332=CARTESIAN_POINT('Ctrl Pts',(19.2971766673034,0.867720598171421,123.641425289948));
#54333=CARTESIAN_POINT('Ctrl Pts',(19.0536927608711,1.02670708997575,123.659385419846));
#54334=CARTESIAN_POINT('Ctrl Pts',(18.7409543977456,1.15682572255536,123.68030601116));
#54335=CARTESIAN_POINT('Ctrl Pts',(18.2706071539656,1.1801061135358,123.708616815304));
#54336=CARTESIAN_POINT('Ctrl Pts',(17.8261572337802,0.965650573995201,123.738296470758));
#54337=CARTESIAN_POINT('Ctrl Pts',(17.5648082264945,0.68326279516643,123.761969786547));
#54338=CARTESIAN_POINT('Ctrl Pts',(17.4273072068287,0.430564305475234,123.779689920843));
#54339=CARTESIAN_POINT('Ctrl Pts',(17.3322102326942,0.059145117553956,123.803271515764));
#54340=CARTESIAN_POINT('Ctrl Pts',(17.3871448081339,-0.37709051742884,123.829725176229));
#54341=CARTESIAN_POINT('Ctrl Pts',(17.6434368073176,-0.783983692022225,
123.859023845048));
#54342=CARTESIAN_POINT('Ctrl Pts',(18.0048650575429,-1.05085396041933,123.886417549706));
#54343=CARTESIAN_POINT('Ctrl Pts',(18.4599937002107,-1.16137052462561,123.914827963259));
#54344=CARTESIAN_POINT('Ctrl Pts',(18.9368144658537,-1.07328772322286,123.944247051069));
#54345=CARTESIAN_POINT('Ctrl Pts',(19.3017920039295,-0.821759581235761,
123.97114044685));
#54346=CARTESIAN_POINT('Ctrl Pts',(19.4813108346333,-0.558607347098734,
123.990653830343));
#54347=CARTESIAN_POINT('Ctrl Pts',(19.5808068475382,-0.316073333612912,
124.006894030936));
#54348=CARTESIAN_POINT('Ctrl Pts',(19.629751852434,-0.06998782398746,124.022304363409));
#54349=CARTESIAN_POINT('Ctrl Pts',(19.6031073407298,0.245268476315917,124.041737432005));
#54350=CARTESIAN_POINT('Ctrl Pts',(19.490435145498,0.54037060471732,124.061139593497));
#54351=CARTESIAN_POINT('Ctrl Pts',(19.30075188909,0.792347731402688,124.08051122595));
#54352=CARTESIAN_POINT('Ctrl Pts',(19.049131072318,0.981672676667765,124.099853680021));
#54353=CARTESIAN_POINT('Ctrl Pts',(18.7798028011389,1.08446740519912,124.117558351805));
#54354=CARTESIAN_POINT('Ctrl Pts',(18.5210831823971,1.1153216790555,124.133633467999));
#54355=CARTESIAN_POINT('Ctrl Pts',(18.2099403540505,1.08709601876646,124.152903665108));
#54356=CARTESIAN_POINT('Ctrl Pts',(17.8458847551693,0.930292968214851,124.176955303819));
#54357=CARTESIAN_POINT('Ctrl Pts',(17.5246246286783,0.580601914550535,124.205762463781));
#54358=CARTESIAN_POINT('Ctrl Pts',(17.3744527732723,0.131077359721622,124.234518546367));
#54359=CARTESIAN_POINT('Ctrl Pts',(17.420912508539,-0.33984008099323,124.263226930259));
#54360=CARTESIAN_POINT('Ctrl Pts',(17.6552915800908,-0.750058113066199,
124.29189122665));
#54361=CARTESIAN_POINT('Ctrl Pts',(18.0362401675348,-1.02839061850904,124.320514971321));
#54362=CARTESIAN_POINT('Ctrl Pts',(18.4970485505493,-1.12672401782067,124.349101783714));
#54363=CARTESIAN_POINT('Ctrl Pts',(18.9572956550727,-1.02839086361948,124.377655277085));
#54364=CARTESIAN_POINT('Ctrl Pts',(19.3368462626138,-0.750940541881326,
124.406179103129));
#54365=CARTESIAN_POINT('Ctrl Pts',(19.5697640099691,-0.343039664832534,
124.434676926364));
#54366=CARTESIAN_POINT('Ctrl Pts',(19.6157329190913,0.12405321556001,124.463152433765));
#54367=CARTESIAN_POINT('Ctrl Pts',(19.4670145957621,0.568894309768287,124.491609324847));
#54368=CARTESIAN_POINT('Ctrl Pts',(19.1497451133398,0.914018292969703,124.520051311987));
#54369=CARTESIAN_POINT('Ctrl Pts',(18.7193548376009,1.09938769324324,124.548482116557));
#54370=CARTESIAN_POINT('Ctrl Pts',(18.2509114822612,1.09280765444621,124.576905469337));
#54371=CARTESIAN_POINT('Ctrl Pts',(17.8260645738587,0.895500222610984,124.605325106134));
#54372=CARTESIAN_POINT('Ctrl Pts',(17.5188553213113,0.541878966350906,124.63374476536));
#54373=CARTESIAN_POINT('Ctrl Pts',(17.382850290681,0.093564086594701,124.662168184265));
#54374=CARTESIAN_POINT('Ctrl Pts',(17.4418279527753,-0.37132399975189,124.690599097016));
#54375=CARTESIAN_POINT('Ctrl Pts',(17.6856332696909,-0.771738353190144,
124.719041234205));
#54376=CARTESIAN_POINT('Ctrl Pts',(18.0719208541219,-1.0377941227316,124.747498318936));
#54377=CARTESIAN_POINT('Ctrl Pts',(18.5334880205951,-1.12293055385139,124.775974064255));
#54378=CARTESIAN_POINT('Ctrl Pts',(18.9899319402798,-1.01203632565444,124.804472169489));
#54379=CARTESIAN_POINT('Ctrl Pts',(19.3616153839255,-0.724124170918624,
124.832996318148));
#54380=CARTESIAN_POINT('Ctrl Pts',(19.5835222166062,-0.309081980170988,
124.861550177472));
#54381=CARTESIAN_POINT('Ctrl Pts',(19.6165983611862,0.160946203785086,124.890137394828));
#54382=CARTESIAN_POINT('Ctrl Pts',(19.4546059082149,0.604064532424729,124.918761594942));
#54383=CARTESIAN_POINT('Ctrl Pts',(19.12529087406,0.942854524119908,124.947426376577));
#54384=CARTESIAN_POINT('Ctrl Pts',(18.6856469205026,1.11786424593928,124.976135310182));
#54385=CARTESIAN_POINT('Ctrl Pts',(18.2120799303225,1.09801324094038,125.004891937497));
#54386=CARTESIAN_POINT('Ctrl Pts',(17.7871660062907,0.886096535343215,125.033699768365));
#54387=CARTESIAN_POINT('Ctrl Pts',(17.4852914068756,0.518415965617182,125.062562277764));
#54388=CARTESIAN_POINT('Ctrl Pts',(17.3596644142994,0.058581772485024,125.091482902918));
#54389=CARTESIAN_POINT('Ctrl Pts',(17.4329608753223,-0.413461509346148,
125.120465040703));
#54390=CARTESIAN_POINT('Ctrl Pts',(17.6932446010896,-0.815297582192034,
125.149512047381));
#54391=CARTESIAN_POINT('Ctrl Pts',(18.0958948026965,-1.07639147921999,125.178627235761));
#54392=CARTESIAN_POINT('Ctrl Pts',(18.5712323214369,-1.15044002046434,125.207813872217));
#54393=CARTESIAN_POINT('Ctrl Pts',(19.0365458838211,-1.02356262279525,125.237075174163));
#54394=CARTESIAN_POINT('Ctrl Pts',(19.4104490395663,-0.716886765308683,
125.266414307353));
#54395=CARTESIAN_POINT('Ctrl Pts',(19.6270820726689,-0.283048207401995,
125.295834385718));
#54396=CARTESIAN_POINT('Ctrl Pts',(19.6476857815032,0.202818052033419,125.325338468895));
#54397=CARTESIAN_POINT('Ctrl Pts',(19.4675178551793,0.656058587293851,125.354929559319));
#54398=CARTESIAN_POINT('Ctrl Pts',(19.1168805933481,0.997217593821377,125.384610600053));
#54399=CARTESIAN_POINT('Ctrl Pts',(18.6560450313014,1.16593620672317,125.414384472115));
#54400=CARTESIAN_POINT('Ctrl Pts',(18.1649169151261,1.13160848108037,125.444253994345));
#54401=CARTESIAN_POINT('Ctrl Pts',(17.7292116516687,0.898915887111277,125.474221921416));
#54402=CARTESIAN_POINT('Ctrl Pts',(17.4255249022822,0.507242292692671,125.504290940928));
#54403=CARTESIAN_POINT('Ctrl Pts',(17.3078934945542,0.0240300154227973,
125.53446367174));
#54404=CARTESIAN_POINT('Ctrl Pts',(17.3982001119431,-0.466807092465915,
125.564742661308));
#54405=CARTESIAN_POINT('Ctrl Pts',(17.6821230641009,-0.87942821936793,125.595130385731));
#54406=CARTESIAN_POINT('Ctrl Pts',(18.1113783174984,-1.141051483794,125.625629247964));
#54407=CARTESIAN_POINT('Ctrl Pts',(18.6119087122778,-1.20476940486866,125.656241575366));
#54408=CARTESIAN_POINT('Ctrl Pts',(19.0966360138455,-1.05794126721894,125.686969618127));
#54409=CARTESIAN_POINT('Ctrl Pts',(19.4805851121993,-0.724663367359761,
125.717815547067));
#54410=CARTESIAN_POINT('Ctrl Pts',(19.6957581501257,-0.261839052557402,
125.748781453597));
#54411=CARTESIAN_POINT('Ctrl Pts',(19.7031582372028,0.250515854950012,125.779869348315));
#54412=CARTESIAN_POINT('Ctrl Pts',(19.4998395183547,0.723084549280525,125.811081158878));
#54413=CARTESIAN_POINT('Ctrl Pts',(19.1197116159269,1.07279807162807,125.84241872872));
#54414=CARTESIAN_POINT('Ctrl Pts',(18.627906276719,1.23741873324107,125.873883815249));
#54415=CARTESIAN_POINT('Ctrl Pts',(18.1096368884415,1.1866007561655,125.905478089829));
#54416=CARTESIAN_POINT('Ctrl Pts',(17.6554525278437,0.927464176176284,125.9372031366));
#54417=CARTESIAN_POINT('Ctrl Pts',(17.3454350244466,0.503660979214375,125.969060450953));
#54418=CARTESIAN_POINT('Ctrl Pts',(17.2350938113461,-0.0119586159299856,
126.001051438261));
#54419=CARTESIAN_POINT('Ctrl Pts',(17.3454405769833,-0.529852130208938,
126.033177412798));
#54420=CARTESIAN_POINT('Ctrl Pts',(17.6590169493212,-0.959319950908805,
126.065439597576));
#54421=CARTESIAN_POINT('Ctrl Pts',(18.1226226383629,-1.2243768780413,126.097839123514));
#54422=CARTESIAN_POINT('Ctrl Pts',(18.6563248547008,-1.2771846378208,126.130377028335));
#54423=CARTESIAN_POINT('Ctrl Pts',(19.167226814877,-1.10667254207858,126.163054255594));
#54424=CARTESIAN_POINT('Ctrl Pts',(19.5656267761898,-0.740794449404953,
126.195871654093));
#54425=CARTESIAN_POINT('Ctrl Pts',(19.7807587891991,-0.241970054075206,
126.228829977697));
#54426=CARTESIAN_POINT('Ctrl Pts',(19.7733541251805,0.303551363615882,126.261929884968));
#54427=CARTESIAN_POINT('Ctrl Pts',(19.5427940986679,0.800595193788684,126.295171938242));
#54428=CARTESIAN_POINT('Ctrl Pts',(19.1275540954992,1.16165967036617,126.328556603354));
#54429=CARTESIAN_POINT('Ctrl Pts',(18.5987999963076,1.322315594875,126.362084248977));
#54430=CARTESIAN_POINT('Ctrl Pts',(18.0482010527672,1.25269600798768,126.395755147454));
#54431=CARTESIAN_POINT('Ctrl Pts',(17.5720393499126,0.963030431464114,126.429569473199));
#54432=CARTESIAN_POINT('Ctrl Pts',(17.2543787451364,0.50219434471344,126.463527304884));
#54433=CARTESIAN_POINT('Ctrl Pts',(17.1522183182203,-0.050520473058097,
126.497628620392));
#54434=CARTESIAN_POINT('Ctrl Pts',(17.28528388398,-0.599054499403936,126.531873306385));
#54435=CARTESIAN_POINT('Ctrl Pts',(17.6322269450083,-1.04725813489579,126.566261140912));
#54436=CARTESIAN_POINT('Ctrl Pts',(18.1340686566346,-1.31578098033913,126.600791826669));
#54437=CARTESIAN_POINT('Ctrl Pts',(18.7041317748905,-1.35605913470818,126.635464928542));
#54438=CARTESIAN_POINT('Ctrl Pts',(19.2431776225041,-1.15920835547423,126.670279991304));
#54439=CARTESIAN_POINT('Ctrl Pts',(19.5875030126131,-0.824597610573135,
126.699410261134));
#54440=CARTESIAN_POINT('Ctrl Pts',(19.7634957162678,-0.489016487416052,
126.722784870598));
#54441=CARTESIAN_POINT('Ctrl Pts',(19.8664282376008,-0.123567048111276,
126.746206118278));
#54442=CARTESIAN_POINT('Ctrl Pts',(19.8463416048187,0.359992052614654,126.775570193968));
#54443=CARTESIAN_POINT('Ctrl Pts',(19.5861832716794,0.881849521800832,126.810945948462));
#54444=CARTESIAN_POINT('Ctrl Pts',(19.1338679365761,1.25337686761882,126.846459712541));
#54445=CARTESIAN_POINT('Ctrl Pts',(18.5670443327571,1.40834569449497,126.882110345098));
#54446=CARTESIAN_POINT('Ctrl Pts',(17.9841681512631,1.31793789072804,126.917896712725));
#54447=CARTESIAN_POINT('Ctrl Pts',(17.4871872481259,0.996134996799377,126.953817536565));
#54448=CARTESIAN_POINT('Ctrl Pts',(17.1638036554832,0.497567483767361,126.989871474656));
#54449=CARTESIAN_POINT('Ctrl Pts',(17.0719279933258,-0.091745800871305,
127.026057079263));
#54450=CARTESIAN_POINT('Ctrl Pts',(17.2293359710647,-0.669255689424998,
127.062372821794));
#54451=CARTESIAN_POINT('Ctrl Pts',(17.610241253734,-1.13374033526755,127.098817081293));
#54452=CARTESIAN_POINT('Ctrl Pts',(18.1495133445035,-1.4030660398855,127.135388152441));
#54453=CARTESIAN_POINT('Ctrl Pts',(18.7538151252911,-1.42872296525937,127.172084240549));
#54454=CARTESIAN_POINT('Ctrl Pts',(19.3177758940829,-1.20456511272855,127.208903469833));
#54455=CARTESIAN_POINT('Ctrl Pts',(19.7423836723087,-0.768176629582259,
127.245843874445));
#54456=CARTESIAN_POINT('Ctrl Pts',(19.9523892723162,-0.194574417684047,
127.282903420998));
#54457=CARTESIAN_POINT('Ctrl Pts',(19.9096554818046,0.416699120440095,127.320079963011));
#54458=CARTESIAN_POINT('Ctrl Pts',(19.6200821414386,0.958872434979693,127.357371346452));
#54459=CARTESIAN_POINT('Ctrl Pts',(19.1328479733187,1.33661667025399,127.394775187569));
#54460=CARTESIAN_POINT('Ctrl Pts',(18.5320571866121,1.4828332255706,127.432289321894));
#54461=CARTESIAN_POINT('Ctrl Pts',(17.9221948628147,1.37057956323489,127.469910942846));
#54462=CARTESIAN_POINT('Ctrl Pts',(17.4099532468711,1.01803725495168,127.507638323144));
#54463=CARTESIAN_POINT('Ctrl Pts',(17.0854953400889,0.485568884820926,127.545467204649));
#54464=CARTESIAN_POINT('Ctrl Pts',(17.006625668042,-0.134612140505952,127.583398399533));
#54465=CARTESIAN_POINT('Ctrl Pts',(17.188418776128,-0.734467438014115,127.621422779654));
#54466=CARTESIAN_POINT('Ctrl Pts',(17.6003366822749,-1.20887205801102,127.65954828209));
#54467=CARTESIAN_POINT('Ctrl Pts',(18.1716172541843,-1.47441118975859,127.69775474856));
#54468=CARTESIAN_POINT('Ctrl Pts',(18.8027604208616,-1.4832332174758,127.736069375441));
#54469=CARTESIAN_POINT('Ctrl Pts',(19.3838788005284,-1.23337426230525,127.774432416617));
#54470=CARTESIAN_POINT('Ctrl Pts',(19.8136026224869,-0.766189668421221,
127.812941446107));
#54471=CARTESIAN_POINT('Ctrl Pts',(20.0138145362224,-0.163792158425567,
127.851457167091));
#54472=CARTESIAN_POINT('Ctrl Pts',(19.9641501694412,0.363252169813094,127.883623693518));
#54473=CARTESIAN_POINT('Ctrl Pts',(19.79432217284,0.747620422811712,127.909505070839));
#54474=CARTESIAN_POINT('Ctrl Pts',(19.608996542054,1.00226608921801,127.928824308732));
#54475=CARTESIAN_POINT('Ctrl Pts',(19.3768569389481,1.21253337912636,127.948129329567));
#54476=CARTESIAN_POINT('Ctrl Pts',(19.108950972945,1.36963666110103,127.967545832416));
#54477=CARTESIAN_POINT('Ctrl Pts',(18.813603063098,1.46669294355822,127.98706761261));
#54478=CARTESIAN_POINT('Ctrl Pts',(18.6035448089217,1.48910415722868,127.999941776888));
#54479=CARTESIAN_POINT('Ctrl Pts',(18.4960527730771,1.49000887282122,128.006304968607));
#54480=CARTESIAN_POINT('Ctrl Pts',(18.49651553697,1.50499871401635,112.870284331898));
#54481=CARTESIAN_POINT('Ctrl Pts',(18.3336126008743,1.50362762800833,112.87992767523));
#54482=CARTESIAN_POINT('Ctrl Pts',(18.1233704382878,1.47030778167341,112.893035123571));
#54483=CARTESIAN_POINT('Ctrl Pts',(17.8312017734791,1.35658915071029,112.91277539402));
#54484=CARTESIAN_POINT('Ctrl Pts',(17.6051956153995,1.22416527432542,112.929156901125));
#54485=CARTESIAN_POINT('Ctrl Pts',(17.3699687728766,1.01106353608856,112.948717313545));
#54486=CARTESIAN_POINT('Ctrl Pts',(17.1818898541377,0.752733756695092,112.968320038741));
#54487=CARTESIAN_POINT('Ctrl Pts',(17.0092492859105,0.36200183096875,112.99462963671));
#54488=CARTESIAN_POINT('Ctrl Pts',(16.9586044369231,-0.174255285116374,
113.027359456216));
#54489=CARTESIAN_POINT('Ctrl Pts',(17.1626159288063,-0.788555902752346,
113.066633020249));
#54490=CARTESIAN_POINT('Ctrl Pts',(17.6017111768839,-1.26616594937551,113.105992819481));
#54491=CARTESIAN_POINT('Ctrl Pts',(18.1967581723796,-1.52214677887222,113.14527795291));
#54492=CARTESIAN_POINT('Ctrl Pts',(18.844504423364,-1.51325397885606,113.184601044115));
#54493=CARTESIAN_POINT('Ctrl Pts',(19.4320735597648,-1.24028824537934,113.223892539239));
#54494=CARTESIAN_POINT('Ctrl Pts',(19.8566981334926,-0.751475885302668,
113.263184243726));
#54495=CARTESIAN_POINT('Ctrl Pts',(20.0445669595258,-0.132045477816717,
113.302451626346));
#54496=CARTESIAN_POINT('Ctrl Pts',(19.9630909675482,0.509755478278449,113.341704280326));
#54497=CARTESIAN_POINT('Ctrl Pts',(19.6267635243402,1.0619677779827,113.380930598247));
#54498=CARTESIAN_POINT('Ctrl Pts',(19.0945974730579,1.42839035694035,113.420131303187));
#54499=CARTESIAN_POINT('Ctrl Pts',(18.4596682384706,1.54539663475943,113.459300732061));
#54500=CARTESIAN_POINT('Ctrl Pts',(17.8328788987336,1.39299167988022,113.498436286584));
#54501=CARTESIAN_POINT('Ctrl Pts',(17.3234976520339,0.998246828811687,113.537533977322));
#54502=CARTESIAN_POINT('Ctrl Pts',(17.0201012712623,0.43047223212316,113.576590529082));
#54503=CARTESIAN_POINT('Ctrl Pts',(16.9751265156656,-0.210968557547024,
113.615602351298));
#54504=CARTESIAN_POINT('Ctrl Pts',(17.1958026171018,-0.814087468865364,
113.654566025983));
#54505=CARTESIAN_POINT('Ctrl Pts',(17.6429797818494,-1.27385693352479,113.693478165596));
#54506=CARTESIAN_POINT('Ctrl Pts',(18.2381149235038,-1.51053956043059,113.732335298242));
#54507=CARTESIAN_POINT('Ctrl Pts',(18.8770399010279,-1.48353546536932,113.77113426794));
#54508=CARTESIAN_POINT('Ctrl Pts',(19.4483164054444,-1.19836309525062,113.809871477796));
#54509=CARTESIAN_POINT('Ctrl Pts',(19.8525979010098,-0.705553496904467,
113.848543962768));
#54510=CARTESIAN_POINT('Ctrl Pts',(20.0200408180881,-0.0916935590501383,
113.887148305216));
#54511=CARTESIAN_POINT('Ctrl Pts',(19.9223241392787,0.535881741945536,113.925681414906));
#54512=CARTESIAN_POINT('Ctrl Pts',(19.5774635624247,1.06775101120009,113.96414018534));
#54513=CARTESIAN_POINT('Ctrl Pts',(19.0465046155246,1.41172133274227,114.002521454301));
#54514=CARTESIAN_POINT('Ctrl Pts',(18.526648067714,1.49238331075636,114.034438886814));
#54515=CARTESIAN_POINT('Ctrl Pts',(18.1188516957653,1.42559012849739,114.059931011469));
#54516=CARTESIAN_POINT('Ctrl Pts',(17.7340973408627,1.27603701185301,114.085394830966));
#54517=CARTESIAN_POINT('Ctrl Pts',(17.329286118754,0.94373241691892,114.117170806693));
#54518=CARTESIAN_POINT('Ctrl Pts',(17.049492258478,0.382568260031224,114.155212625842));
#54519=CARTESIAN_POINT('Ctrl Pts',(17.0233344994864,-0.242377855811677,
114.193162521077));
#54520=CARTESIAN_POINT('Ctrl Pts',(17.2541617793634,-0.822071654025293,
114.231017692788));
#54521=CARTESIAN_POINT('Ctrl Pts',(17.7004709588697,-1.25579236892624,114.268775475679));
#54522=CARTESIAN_POINT('Ctrl Pts',(18.2834652007333,-1.46882945434736,114.306433293321));
#54523=CARTESIAN_POINT('Ctrl Pts',(18.9009375287065,-1.42527515643007,114.343988609376));
#54524=CARTESIAN_POINT('Ctrl Pts',(19.4452400385389,-1.13413243348152,114.381438939098));
#54525=CARTESIAN_POINT('Ctrl Pts',(19.8220671838761,-0.647455723515675,
114.418781942662));
#54526=CARTESIAN_POINT('Ctrl Pts',(19.9668177841584,-0.0510774300832363,
114.456015241884));
#54527=CARTESIAN_POINT('Ctrl Pts',(19.855686038565,0.550611907288274,114.493136645638));
#54528=CARTESIAN_POINT('Ctrl Pts',(19.5095622696879,1.05286323816987,114.530143966639));
#54529=CARTESIAN_POINT('Ctrl Pts',(18.9901066793641,1.36894922551202,114.567035111385));
#54530=CARTESIAN_POINT('Ctrl Pts',(18.3887907442047,1.4450452249503,114.603808080057));
#54531=CARTESIAN_POINT('Ctrl Pts',(17.810731402714,1.26947343893433,114.640460935603));
#54532=CARTESIAN_POINT('Ctrl Pts',(17.3563198980319,0.874426270620376,114.676991833415));
#54533=CARTESIAN_POINT('Ctrl Pts',(17.1037586025035,0.330076715915367,114.713399007585));
#54534=CARTESIAN_POINT('Ctrl Pts',(17.0955891084954,-0.267878922353754,
114.74968077348));
#54535=CARTESIAN_POINT('Ctrl Pts',(17.3315462787181,-0.815111405623883,
114.785835540599));
#54536=CARTESIAN_POINT('Ctrl Pts',(17.7688643629591,-1.2167760559352,114.821861785405));
#54537=CARTESIAN_POINT('Ctrl Pts',(18.3300985159098,-1.40416354888984,114.857758110311));
#54538=CARTESIAN_POINT('Ctrl Pts',(18.8189384921563,-1.35575323505928,114.887562293732));
#54539=CARTESIAN_POINT('Ctrl Pts',(19.1716912067797,-1.20042508413519,114.911339401126));
#54540=CARTESIAN_POINT('Ctrl Pts',(19.4840903420183,-0.975859670364661,
114.935072168859));
#54541=CARTESIAN_POINT('Ctrl Pts',(19.7716878728692,-0.582133605641874,
114.964654504561));
#54542=CARTESIAN_POINT('Ctrl Pts',(19.8931529911131,-0.0120119416229624,
115.000018638428));
#54543=CARTESIAN_POINT('Ctrl Pts',(19.7716793443981,0.555774460771906,115.035247022951));
#54544=CARTESIAN_POINT('Ctrl Pts',(19.4301928094659,1.02262655518765,115.07033883131));
#54545=CARTESIAN_POINT('Ctrl Pts',(18.9297825002282,1.30814522073825,115.105293244196));
#54546=CARTESIAN_POINT('Ctrl Pts',(18.3586637335548,1.36416104789949,115.140109582566));
#54547=CARTESIAN_POINT('Ctrl Pts',(17.816632406542,1.18272719467699,115.17478723275));
#54548=CARTESIAN_POINT('Ctrl Pts',(17.3976999462254,0.797309431344444,115.209325696987));
#54549=CARTESIAN_POINT('Ctrl Pts',(17.1735784716011,0.276454513248407,115.243724548093));
#54550=CARTESIAN_POINT('Ctrl Pts',(17.1809199116676,-0.22536964366726,115.274176940408));
#54551=CARTESIAN_POINT('Ctrl Pts',(17.3354710467395,-0.629195288576481,
115.300731925094));
#54552=CARTESIAN_POINT('Ctrl Pts',(17.502022403867,-0.850655511550889,115.31775626652));
#54553=CARTESIAN_POINT('Ctrl Pts',(17.6358232956015,-0.975224668920173,
115.329086323583));
#54554=CARTESIAN_POINT('Ctrl Pts',(17.7067764065314,-1.03268658588934,115.334747457085));
#54555=CARTESIAN_POINT('Ctrl Pts',(17.7816008739847,-1.08494819346858,115.340404694511));
#54556=CARTESIAN_POINT('Ctrl Pts',(17.9380013948717,-1.17876364558541,115.351711369109));
#54557=CARTESIAN_POINT('Ctrl Pts',(18.1955706816015,-1.27700122758528,115.368642182192));
#54558=CARTESIAN_POINT('Ctrl Pts',(18.5607517830549,-1.30775052484681,115.391154193319));
#54559=CARTESIAN_POINT('Ctrl Pts',(18.9192839923125,-1.23635697638592,115.413603956782));
#54560=CARTESIAN_POINT('Ctrl Pts',(19.24295722527,-1.06902914440793,115.435991388812));
#54561=CARTESIAN_POINT('Ctrl Pts',(19.5072304818416,-0.819230463869382,
115.458316697458));
#54562=CARTESIAN_POINT('Ctrl Pts',(19.690959734946,-0.507076536075454,115.480579842894));
#54563=CARTESIAN_POINT('Ctrl Pts',(19.8121732723121,-0.0402072384437589,
115.51018141997));
#54564=CARTESIAN_POINT('Ctrl Pts',(19.7291627781261,0.446553891594026,115.53965926837));
#54565=CARTESIAN_POINT('Ctrl Pts',(19.4957563328109,0.793998696574734,115.565344565252));
#54566=CARTESIAN_POINT('Ctrl Pts',(19.3263627711921,0.959025218074687,115.579991285573));
#54567=CARTESIAN_POINT('Ctrl Pts',(19.1353328686529,1.09850403796305,115.594617483237));
#54568=CARTESIAN_POINT('Ctrl Pts',(18.9457036306386,1.18342968358787,115.607388621145));
#54569=CARTESIAN_POINT('Ctrl Pts',(18.7746135630278,1.22619954854511,115.618316371275));
#54570=CARTESIAN_POINT('Ctrl Pts',(18.6879200730088,1.24156918634862,115.623776397083));
#54571=CARTESIAN_POINT('Ctrl Pts',(18.6149671512159,1.24929495538121,115.628323271269));
#54572=CARTESIAN_POINT('Ctrl Pts',(18.5564232901343,1.25232080760023,115.631958822256));
#54573=CARTESIAN_POINT('Ctrl Pts',(18.3188555044749,1.25686234907179,115.646698035442));
#54574=CARTESIAN_POINT('Ctrl Pts',(17.8888715430467,1.14680181043036,115.673379735934));
#54575=CARTESIAN_POINT('Ctrl Pts',(17.5243082161196,0.808308860592351,115.703303215303));
#54576=CARTESIAN_POINT('Ctrl Pts',(17.3625257033883,0.50390079334422,115.72460706276));
#54577=CARTESIAN_POINT('Ctrl Pts',(17.3075338582628,0.340949365208199,115.735241634511));
#54578=CARTESIAN_POINT('Ctrl Pts',(17.2805316366918,0.206509233398448,115.743738908119));
#54579=CARTESIAN_POINT('Ctrl Pts',(17.2483095255158,-0.0656048243204948,
115.760719371947));
#54580=CARTESIAN_POINT('Ctrl Pts',(17.3281117828854,-0.516084464963803,
115.788234052639));
#54581=CARTESIAN_POINT('Ctrl Pts',(17.7215430539041,-1.00896792873564,115.826146275045));
#54582=CARTESIAN_POINT('Ctrl Pts',(18.2516949275413,-1.2318489526899,115.860731644079));
#54583=CARTESIAN_POINT('Ctrl Pts',(18.765074033174,-1.21206507972195,115.892041349858));
#54584=CARTESIAN_POINT('Ctrl Pts',(19.1871807387752,-1.02791702813592,115.9201196661));
#54585=CARTESIAN_POINT('Ctrl Pts',(19.5117099232347,-0.703109660480611,
115.94809877643));
#54586=CARTESIAN_POINT('Ctrl Pts',(19.6639431963501,-0.353759299179872,
115.971332775432));
#54587=CARTESIAN_POINT('Ctrl Pts',(19.7029577450344,-0.0560681711860727,
115.989871790982));
#54588=CARTESIAN_POINT('Ctrl Pts',(19.6903956065854,0.168277428115539,116.003751582154));
#54589=CARTESIAN_POINT('Ctrl Pts',(19.6453583039838,0.349777156774072,116.01529861874));
#54590=CARTESIAN_POINT('Ctrl Pts',(19.5896345786186,0.487827454310805,116.024524180344));
#54591=CARTESIAN_POINT('Ctrl Pts',(19.4873268530305,0.686149792199375,116.038350531065));
#54592=CARTESIAN_POINT('Ctrl Pts',(19.2657788090282,0.94342374801498,116.059046301773));
#54593=CARTESIAN_POINT('Ctrl Pts',(18.8668133161929,1.15412635411037,116.086547373941));
#54594=CARTESIAN_POINT('Ctrl Pts',(18.4199331148969,1.20433642524023,116.113957070661));
#54595=CARTESIAN_POINT('Ctrl Pts',(18.0952779029817,1.11723399930278,116.134446884645));
#54596=CARTESIAN_POINT('Ctrl Pts',(17.9017889644904,1.01249991695947,116.148079023699));
#54597=CARTESIAN_POINT('Ctrl Pts',(17.7799369999649,0.93110838138898,116.157159621741));
#54598=CARTESIAN_POINT('Ctrl Pts',(17.5882472578648,0.759856044959128,116.173032149632));
#54599=CARTESIAN_POINT('Ctrl Pts',(17.4598618042694,0.5557237355446,116.187734998419));
#54600=CARTESIAN_POINT('Ctrl Pts',(17.3974802528664,0.384644782920287,116.199025088643));
#54601=CARTESIAN_POINT('Ctrl Pts',(17.3811086459147,0.332571473631556,116.202410852429));
#54602=CARTESIAN_POINT('Ctrl Pts',(17.3672458383465,0.27977617854763,116.205795247183));
#54603=CARTESIAN_POINT('Ctrl Pts',(17.3558537656234,0.226430775875569,116.209178339773));
#54604=CARTESIAN_POINT('Ctrl Pts',(17.3469543264664,0.172623320191819,116.212560079634));
#54605=CARTESIAN_POINT('Ctrl Pts',(17.3385176348533,0.100437721270174,116.217067299795));
#54606=CARTESIAN_POINT('Ctrl Pts',(17.3290322213833,-0.0992654325487338,
116.229454683121));
#54607=CARTESIAN_POINT('Ctrl Pts',(17.3908483892394,-0.425368273174374,
116.249686405889));
#54608=CARTESIAN_POINT('Ctrl Pts',(17.6256909219847,-0.79889129542694,116.276579485812));
#54609=CARTESIAN_POINT('Ctrl Pts',(17.9796947676307,-1.06001015743842,116.303392710883));
#54610=CARTESIAN_POINT('Ctrl Pts',(18.4034077753438,-1.17341375372982,116.330127316022));
#54611=CARTESIAN_POINT('Ctrl Pts',(18.8379681316464,-1.12433617754085,116.356785513166));
#54612=CARTESIAN_POINT('Ctrl Pts',(19.2235542763837,-0.92044124263072,116.383368803318));
#54613=CARTESIAN_POINT('Ctrl Pts',(19.4440554391474,-0.663980494317338,
116.403988454749));
#54614=CARTESIAN_POINT('Ctrl Pts',(19.5497056653311,-0.451252453324442,
116.418690018913));
#54615=CARTESIAN_POINT('Ctrl Pts',(19.6122761625615,-0.272121955888386,
116.430441476114));
#54616=CARTESIAN_POINT('Ctrl Pts',(19.6624926907458,0.0578739594259051,
116.450978681812));
#54617=CARTESIAN_POINT('Ctrl Pts',(19.5541359914442,0.532226076482499,116.480242353973));
#54618=CARTESIAN_POINT('Ctrl Pts',(19.1686764482267,0.968561647204002,116.515242131433));
#54619=CARTESIAN_POINT('Ctrl Pts',(18.6234304609746,1.16678220457797,116.550130731072));
#54620=CARTESIAN_POINT('Ctrl Pts',(18.0513874432561,1.08037506712942,116.58491296496));
#54621=CARTESIAN_POINT('Ctrl Pts',(17.6588194184233,0.782699663211421,116.614536530482));
#54622=CARTESIAN_POINT('Ctrl Pts',(17.4566975083438,0.43862940460328,116.639049224404));
#54623=CARTESIAN_POINT('Ctrl Pts',(17.3504735057365,0.0302010042763518,
116.664964912131));
#54624=CARTESIAN_POINT('Ctrl Pts',(17.441318190632,-0.504074055082703,116.697288303009));
#54625=CARTESIAN_POINT('Ctrl Pts',(17.8738322445769,-0.98766591140209,116.735970603409));
#54626=CARTESIAN_POINT('Ctrl Pts',(18.4956494809416,-1.16653777136026,116.774554938272));
#54627=CARTESIAN_POINT('Ctrl Pts',(19.1158561890266,-0.987678591541207,
116.813049296759));
#54628=CARTESIAN_POINT('Ctrl Pts',(19.5451029837921,-0.507162506325275,
116.851462000512));
#54629=CARTESIAN_POINT('Ctrl Pts',(19.6344500864472,0.0209568317628616,
116.883411031743));
#54630=CARTESIAN_POINT('Ctrl Pts',(19.529835344982,0.423259543631477,116.908938003123));
#54631=CARTESIAN_POINT('Ctrl Pts',(19.3719778191083,0.69166285162635,116.928067552668));
#54632=CARTESIAN_POINT('Ctrl Pts',(19.1455454752817,0.905164315225213,116.947183404083));
#54633=CARTESIAN_POINT('Ctrl Pts',(18.7774209857398,1.09622260692838,116.972653115984));
#54634=CARTESIAN_POINT('Ctrl Pts',(18.2449951046063,1.12623059429594,117.004460418568));
#54635=CARTESIAN_POINT('Ctrl Pts',(17.6853267542694,0.816754701388943,117.042589105265));
#54636=CARTESIAN_POINT('Ctrl Pts',(17.3763805857206,0.25760776168484,117.080686636608));
#54637=CARTESIAN_POINT('Ctrl Pts',(17.4122036778926,-0.379923978041567,
117.118761454777));
#54638=CARTESIAN_POINT('Ctrl Pts',(17.7815850748894,-0.900446847787842,
117.156822292918));
#54639=CARTESIAN_POINT('Ctrl Pts',(18.3711855462016,-1.14467562030106,117.194877755412));
#54640=CARTESIAN_POINT('Ctrl Pts',(19.0004142784978,-1.03777979468232,117.232936530983));
#54641=CARTESIAN_POINT('Ctrl Pts',(19.4764865869262,-0.612388047726278,
117.271007271204));
#54642=CARTESIAN_POINT('Ctrl Pts',(19.6533828286409,0.0014177969022171,
117.309098626614));
#54643=CARTESIAN_POINT('Ctrl Pts',(19.4764842231535,0.615731147059621,117.347219206504));
#54644=CARTESIAN_POINT('Ctrl Pts',(18.9994059623802,1.04220793738651,117.385377605214));
#54645=CARTESIAN_POINT('Ctrl Pts',(18.3677905909605,1.14964530042269,117.423582363643));
#54646=CARTESIAN_POINT('Ctrl Pts',(17.7749675945259,0.904241094560212,117.461841957937));
#54647=CARTESIAN_POINT('Ctrl Pts',(17.4029459302078,0.380199033566501,117.500164805045));
#54648=CARTESIAN_POINT('Ctrl Pts',(17.3666607130067,-0.26264953413493,117.53855925612));
#54649=CARTESIAN_POINT('Ctrl Pts',(17.6785947502515,-0.827443121223426,
117.577033557529));
#54650=CARTESIAN_POINT('Ctrl Pts',(18.2444674988179,-1.14045467464445,117.615595868649));
#54651=CARTESIAN_POINT('Ctrl Pts',(18.8917850917382,-1.10432648074206,117.654254235677));
#54652=CARTESIAN_POINT('Ctrl Pts',(19.4220254974689,-0.728402023842326,
117.693016621745));
#54653=CARTESIAN_POINT('Ctrl Pts',(19.6718587015237,-0.126164954214387,
117.731890784944));
#54654=CARTESIAN_POINT('Ctrl Pts',(19.5806405630026,0.411019352712336,117.764385541049));
#54655=CARTESIAN_POINT('Ctrl Pts',(19.3441675709589,0.763295298332512,117.790444769066));
#54656=CARTESIAN_POINT('Ctrl Pts',(19.0201301369936,1.03823903341511,117.816547739909));
#54657=CARTESIAN_POINT('Ctrl Pts',(18.493178198775,1.19052995092288,117.849260188486));
#54658=CARTESIAN_POINT('Ctrl Pts',(17.8581591562469,1.00786619563251,117.888656951998));
#54659=CARTESIAN_POINT('Ctrl Pts',(17.4160248614217,0.51366844782423,117.928202267748));
#54660=CARTESIAN_POINT('Ctrl Pts',(17.3041141976344,-0.142668645446928,
117.967903170292));
#54661=CARTESIAN_POINT('Ctrl Pts',(17.5595850207467,-0.760412353891034,
118.007766241407));
#54662=CARTESIAN_POINT('Ctrl Pts',(18.1068550165682,-1.1492371242961,118.04779801726));
#54663=CARTESIAN_POINT('Ctrl Pts',(18.7800314200528,-1.18744473707504,118.088004749543));
#54664=CARTESIAN_POINT('Ctrl Pts',(19.3730344071082,-0.860233663725908,
118.128392532671));
#54665=CARTESIAN_POINT('Ctrl Pts',(19.7025519711489,-0.26486780951679,118.168967176754));
#54666=CARTESIAN_POINT('Ctrl Pts',(19.6647053513366,0.417645340336696,118.209734371169));
#54667=CARTESIAN_POINT('Ctrl Pts',(19.267503779961,0.978374259812269,118.250699402105));
#54668=CARTESIAN_POINT('Ctrl Pts',(18.7362494566518,1.19864104439097,118.285006242352));
#54669=CARTESIAN_POINT('Ctrl Pts',(18.2877057344592,1.18528122231896,118.312555556409));
#54670=CARTESIAN_POINT('Ctrl Pts',(17.9664308123881,1.08327575222911,118.333270290751));
#54671=CARTESIAN_POINT('Ctrl Pts',(17.6852323698027,0.895287772551696,118.354037962367));
#54672=CARTESIAN_POINT('Ctrl Pts',(17.4664950224042,0.636435219092414,118.374859570174));
#54673=CARTESIAN_POINT('Ctrl Pts',(17.3276081719734,0.326162075674822,118.39573521112));
#54674=CARTESIAN_POINT('Ctrl Pts',(17.2799229603302,-0.0111919817315693,
118.41666582645));
#54675=CARTESIAN_POINT('Ctrl Pts',(17.327598035555,-0.349579187274582,118.437651539655));
#54676=CARTESIAN_POINT('Ctrl Pts',(17.4441956547223,-0.610077653010874,
118.455186324647));
#54677=CARTESIAN_POINT('Ctrl Pts',(17.5782188017048,-0.793582078732169,
118.469242010708));
#54678=CARTESIAN_POINT('Ctrl Pts',(17.7368454389062,-0.956441180317881,
118.483316881728));
#54679=CARTESIAN_POINT('Ctrl Pts',(18.0705782583969,-1.18054323096259,118.507997048192));
#54680=CARTESIAN_POINT('Ctrl Pts',(18.6554412304203,-1.28059964969612,118.543397636231));
#54681=CARTESIAN_POINT('Ctrl Pts',(19.3177414533384,-1.00686280515393,118.586110181979));
#54682=CARTESIAN_POINT('Ctrl Pts',(19.6650536664888,-0.517774642787662,
118.621899795047));
#54683=CARTESIAN_POINT('Ctrl Pts',(19.7442788642631,-0.115645277500642,
118.6470566672));
#54684=CARTESIAN_POINT('Ctrl Pts',(19.7411794524541,0.116933901702342,118.661461743122));
#54685=CARTESIAN_POINT('Ctrl Pts',(19.7054157650643,0.347518370662662,118.675886972296));
#54686=CARTESIAN_POINT('Ctrl Pts',(19.6003745425333,0.622016252827566,118.693955916805));
#54687=CARTESIAN_POINT('Ctrl Pts',(19.317257629013,0.99995885328799,118.722946752854));
#54688=CARTESIAN_POINT('Ctrl Pts',(18.7836518879622,1.29558280479233,118.759336777127));
#54689=CARTESIAN_POINT('Ctrl Pts',(18.0482527405502,1.2548599580439,118.803249169655));
#54690=CARTESIAN_POINT('Ctrl Pts',(17.4439365823436,0.826778385158046,118.847407475872));
#54691=CARTESIAN_POINT('Ctrl Pts',(17.2061922029869,0.253734869760506,118.884412115397));
#54692=CARTESIAN_POINT('Ctrl Pts',(17.2206748920695,-0.230259004950036,
118.914139911465));
#54693=CARTESIAN_POINT('Ctrl Pts',(17.3122772963604,-0.519205211008821,
118.932771615628));
#54694=CARTESIAN_POINT('Ctrl Pts',(17.4173179411385,-0.702637921404735,
118.945841005029));
#54695=CARTESIAN_POINT('Ctrl Pts',(17.4876798042075,-0.800486720086772,
118.953317008868));
#54696=CARTESIAN_POINT('Ctrl Pts',(17.564941377458,-0.89325038450052,118.960798213382));
#54697=CARTESIAN_POINT('Ctrl Pts',(17.6733776392394,-0.998701561839941,
118.970159456938));
#54698=CARTESIAN_POINT('Ctrl Pts',(17.869064246506,-1.1417814231385,118.985158206556));
#54699=CARTESIAN_POINT('Ctrl Pts',(18.1482054520686,-1.26678297579892,119.003945578663));
#54700=CARTESIAN_POINT('Ctrl Pts',(18.512660466752,-1.31830065871435,119.026552828765));
#54701=CARTESIAN_POINT('Ctrl Pts',(18.8781159084707,-1.26677700093841,119.049222381195));
#54702=CARTESIAN_POINT('Ctrl Pts',(19.2159631951799,-1.11568341872246,119.07195433768));
#54703=CARTESIAN_POINT('Ctrl Pts',(19.4995484771516,-0.876304025124276,
119.094748533567));
#54704=CARTESIAN_POINT('Ctrl Pts',(19.7063441509456,-0.566943680968072,
119.11760507113));
#54705=CARTESIAN_POINT('Ctrl Pts',(19.8197309451019,-0.211442999295146,
119.140523685235));
#54706=CARTESIAN_POINT('Ctrl Pts',(19.8302792102411,0.162535549658454,119.163504530996));
#54707=CARTESIAN_POINT('Ctrl Pts',(19.7522781137547,0.465296426729761,119.182706741));
#54708=CARTESIAN_POINT('Ctrl Pts',(19.6410989464218,0.687817901944263,119.19809956578));
#54709=CARTESIAN_POINT('Ctrl Pts',(19.4647313674719,0.944433947569229,119.217366235714));
#54710=CARTESIAN_POINT('Ctrl Pts',(19.1203100782122,1.22737777491237,119.244411622083));
#54711=CARTESIAN_POINT('Ctrl Pts',(18.5652296939497,1.37913493579527,119.279322521792));
#54712=CARTESIAN_POINT('Ctrl Pts',(17.9943789266596,1.29059989009301,119.314371048622));
#54713=CARTESIAN_POINT('Ctrl Pts',(17.5075663391158,0.975396843352528,119.349556416458));
#54714=CARTESIAN_POINT('Ctrl Pts',(17.1907406802648,0.486956739770124,119.38487780746));
#54715=CARTESIAN_POINT('Ctrl Pts',(17.1007177860647,-0.0904629952018157,
119.420334217929));
#54716=CARTESIAN_POINT('Ctrl Pts',(17.2549451352662,-0.656474628556876,
119.455924718063));
#54717=CARTESIAN_POINT('Ctrl Pts',(17.5661243855808,-1.03583821018366,119.485694096377));
#54718=CARTESIAN_POINT('Ctrl Pts',(17.8926570460436,-1.24382698529492,119.509575590226));
#54719=CARTESIAN_POINT('Ctrl Pts',(18.2558106009391,-1.37997354885633,119.533500603368));
#54720=CARTESIAN_POINT('Ctrl Pts',(18.7496196816727,-1.40102252601465,119.563488460007));
#54721=CARTESIAN_POINT('Ctrl Pts',(19.302802351283,-1.1811288001459,119.599602804378));
#54722=CARTESIAN_POINT('Ctrl Pts',(19.7193843468129,-0.753024059784299,
119.635844665495));
#54723=CARTESIAN_POINT('Ctrl Pts',(19.9254897572766,-0.190124415181504,
119.672212430828));
#54724=CARTESIAN_POINT('Ctrl Pts',(19.8835551265898,0.409891451814051,119.708704471057));
#54725=CARTESIAN_POINT('Ctrl Pts',(19.5992582389472,0.942231735537137,119.745319028385));
#54726=CARTESIAN_POINT('Ctrl Pts',(19.120735909551,1.31324454186643,119.782054298589));
#54727=CARTESIAN_POINT('Ctrl Pts',(18.5305348998093,1.45689202451587,119.818908350599));
#54728=CARTESIAN_POINT('Ctrl Pts',(17.9311917661294,1.34662904570844,119.855879245505));
#54729=CARTESIAN_POINT('Ctrl Pts',(17.5116220005748,1.05780154061175,119.886783901806));
#54730=CARTESIAN_POINT('Ctrl Pts',(17.2681007112558,0.738313939272634,119.911563959347));
#54731=CARTESIAN_POINT('Ctrl Pts',(17.0957154156509,0.374823924233557,119.936381231006));
#54732=CARTESIAN_POINT('Ctrl Pts',(17.0309927941948,-0.133517822775856,
119.967471718131));
#54733=CARTESIAN_POINT('Ctrl Pts',(17.2098570169801,-0.723745817563428,
120.004888433649));
#54734=CARTESIAN_POINT('Ctrl Pts',(17.6153203269838,-1.19074555891921,120.042410870425));
#54735=CARTESIAN_POINT('Ctrl Pts',(18.1777197790016,-1.45213042815002,120.080036611004));
#54736=CARTESIAN_POINT('Ctrl Pts',(18.7994854721492,-1.46102141363347,120.11776312502));
#54737=CARTESIAN_POINT('Ctrl Pts',(19.3721419323586,-1.21453953940101,120.155587847869));
#54738=CARTESIAN_POINT('Ctrl Pts',(19.7952400432308,-0.754491980125082,
120.193508128623));
#54739=CARTESIAN_POINT('Ctrl Pts',(19.9940145933377,-0.160304321379954,
120.231521263177));
#54740=CARTESIAN_POINT('Ctrl Pts',(19.9326093252334,0.464726279580436,120.269624478708));
#54741=CARTESIAN_POINT('Ctrl Pts',(19.620552160879,1.01140912119698,120.307814943475));
#54742=CARTESIAN_POINT('Ctrl Pts',(19.1112964283598,1.38377060349613,120.34608976467));
#54743=CARTESIAN_POINT('Ctrl Pts',(18.493054159353,1.51592840621915,120.384445993232));
#54744=CARTESIAN_POINT('Ctrl Pts',(17.8734911230083,1.38376736011695,120.422880625353));
#54745=CARTESIAN_POINT('Ctrl Pts',(17.3609452757673,1.00933886152342,120.461390604502));
#54746=CARTESIAN_POINT('Ctrl Pts',(17.0454493832622,0.457183766611044,120.499972821949));
#54747=CARTESIAN_POINT('Ctrl Pts',(16.9828884983602,-0.176810342706842,
120.5386241196));
#54748=CARTESIAN_POINT('Ctrl Pts',(17.1850847559295,-0.782090219748437,
120.577341292721));
#54749=CARTESIAN_POINT('Ctrl Pts',(17.617571957069,-1.25274977112251,120.616121092604));
#54750=CARTESIAN_POINT('Ctrl Pts',(18.2054777306114,-1.50609466901128,120.654960228881));
#54751=CARTESIAN_POINT('Ctrl Pts',(18.8465084682623,-1.49719808014636,120.693855368907));
#54752=CARTESIAN_POINT('Ctrl Pts',(19.4287811906121,-1.2268814515038,120.732803143256));
#54753=CARTESIAN_POINT('Ctrl Pts',(19.850388348535,-0.741698347844994,120.771800144215));
#54754=CARTESIAN_POINT('Ctrl Pts',(20.0372674102143,-0.125904739992541,
120.810842936167));
#54755=CARTESIAN_POINT('Ctrl Pts',(19.9562362814235,0.513203014455754,120.849928044874));
#54756=CARTESIAN_POINT('Ctrl Pts',(19.6208945619106,1.0640151196956,120.889051981027));
#54757=CARTESIAN_POINT('Ctrl Pts',(19.0893414896838,1.43014628984235,120.928211200816));
#54758=CARTESIAN_POINT('Ctrl Pts',(18.4540890328838,1.54731880733756,120.967402188646));
#54759=CARTESIAN_POINT('Ctrl Pts',(17.8259326540409,1.39470008780894,121.006621310676));
#54760=CARTESIAN_POINT('Ctrl Pts',(17.3145823586523,0.998555219088929,121.045865097348));
#54761=CARTESIAN_POINT('Ctrl Pts',(17.0094747415844,0.427826827738151,121.085129718059));
#54762=CARTESIAN_POINT('Ctrl Pts',(16.9640777387006,-0.218091263932203,
121.124411982227));
#54763=CARTESIAN_POINT('Ctrl Pts',(17.130918600528,-0.674247594855583,121.153883510412));
#54764=CARTESIAN_POINT('Ctrl Pts',(17.3138014149502,-0.933512874257721,
121.173534979156));
#54765=CARTESIAN_POINT('Ctrl Pts',(17.4530421733364,-1.09265995262176,121.186636051418));
#54766=CARTESIAN_POINT('Ctrl Pts',(17.7385750620485,-1.33073917465461,121.209565675458));
#54767=CARTESIAN_POINT('Ctrl Pts',(18.2401816117862,-1.53044037240608,121.242325830746));
#54768=CARTESIAN_POINT('Ctrl Pts',(18.8876846243691,-1.50314303435984,121.281640996012));
#54769=CARTESIAN_POINT('Ctrl Pts',(19.4674781468588,-1.21384361944328,121.320955204458));
#54770=CARTESIAN_POINT('Ctrl Pts',(19.8785262374103,-0.712971704074119,
121.360264930557));
#54771=CARTESIAN_POINT('Ctrl Pts',(20.0490844123739,-0.0880460210185634,
121.399566456549));
#54772=CARTESIAN_POINT('Ctrl Pts',(19.9495540137019,0.551858347376732,121.438856173297));
#54773=CARTESIAN_POINT('Ctrl Pts',(19.5974666870083,1.09507568907155,121.478130424469));
#54774=CARTESIAN_POINT('Ctrl Pts',(19.0544768654203,1.44693457162279,121.517385592229));
#54775=CARTESIAN_POINT('Ctrl Pts',(18.4154972537208,1.54625877810524,121.556618056793));
#54776=CARTESIAN_POINT('Ctrl Pts',(17.7920996522822,1.37604183951388,121.595824221844));
#54777=CARTESIAN_POINT('Ctrl Pts',(17.2929810705988,0.966354646499578,121.635000506818));
#54778=CARTESIAN_POINT('Ctrl Pts',(17.004980218725,0.389027537158531,121.674143350793));
#54779=CARTESIAN_POINT('Ctrl Pts',(16.9779354617802,-0.254970506734332,
121.713249217133));
#54780=CARTESIAN_POINT('Ctrl Pts',(17.2160457097184,-0.853225362726958,
121.752314588298));
#54781=CARTESIAN_POINT('Ctrl Pts',(17.6772270736164,-1.30153725689535,121.791335987055));
#54782=CARTESIAN_POINT('Ctrl Pts',(18.280563801658,-1.522109234509,121.830309943406));
#54783=CARTESIAN_POINT('Ctrl Pts',(18.9205345174637,-1.47706436765061,121.869233063613));
#54784=CARTESIAN_POINT('Ctrl Pts',(19.4854989461127,-1.17497713175005,121.908101903289));
#54785=CARTESIAN_POINT('Ctrl Pts',(19.877218120182,-0.669217905916773,121.946913212876));
#54786=CARTESIAN_POINT('Ctrl Pts',(20.027954611204,-0.0485663563189042,
121.985663485908));
#54787=CARTESIAN_POINT('Ctrl Pts',(19.9122221117287,0.578502033445827,122.024349735476));
#54788=CARTESIAN_POINT('Ctrl Pts',(19.5510980447147,1.10267673035263,122.062968476763));
#54789=CARTESIAN_POINT('Ctrl Pts',(19.008358735754,1.4330323440933,122.101516650726));
#54790=CARTESIAN_POINT('Ctrl Pts',(18.3792313621179,1.51273490014566,122.139991110259));
#54791=CARTESIAN_POINT('Ctrl Pts',(17.7736319859323,1.3288869614174,122.178388737758));
#54792=CARTESIAN_POINT('Ctrl Pts',(17.2969403519651,0.914578061633921,122.216706534334));
#54793=CARTESIAN_POINT('Ctrl Pts',(17.0316254152085,0.342938327687217,122.254941518211));
#54794=CARTESIAN_POINT('Ctrl Pts',(17.0229584803841,-0.285798262575817,
122.293090735968));
#54795=CARTESIAN_POINT('Ctrl Pts',(17.2712780130928,-0.861895236579561,
122.331151377767));
#54796=CARTESIAN_POINT('Ctrl Pts',(17.7321373752124,-1.28529911750752,122.369120583684));
#54797=CARTESIAN_POINT('Ctrl Pts',(18.324268585886,-1.48304302933555,122.406995648865));
#54798=CARTESIAN_POINT('Ctrl Pts',(18.943934995372,-1.42184009998327,122.444773893392));
#54799=CARTESIAN_POINT('Ctrl Pts',(19.4831319671316,-1.11368417665321,122.482452674253));
#54800=CARTESIAN_POINT('Ctrl Pts',(19.8484430472875,-0.613528621914714,
122.520029499532));
#54801=CARTESIAN_POINT('Ctrl Pts',(19.9772418314858,-0.00946603320977227,
122.55750183048));
#54802=CARTESIAN_POINT('Ctrl Pts',(19.8484484572925,0.592790433281014,122.594867332922));
#54803=CARTESIAN_POINT('Ctrl Pts',(19.4859506986768,1.08847020229008,122.632123577563));
#54804=CARTESIAN_POINT('Ctrl Pts',(18.9542199651723,1.39193826091876,122.669268450296));
#54805=CARTESIAN_POINT('Ctrl Pts',(18.3467642170425,1.45156152895867,122.706299619877));
#54806=CARTESIAN_POINT('Ctrl Pts',(17.769753863205,1.25849341836473,122.743215077924));
#54807=CARTESIAN_POINT('Ctrl Pts',(17.3233542581996,0.847860663667533,122.78001275512));
#54808=CARTESIAN_POINT('Ctrl Pts',(17.0843926590814,0.292596511201441,122.816690711866));
#54809=CARTESIAN_POINT('Ctrl Pts',(17.092085167056,-0.243030263092677,122.849185287392));
#54810=CARTESIAN_POINT('Ctrl Pts',(17.257257453301,-0.673940750281189,122.87753804838));
#54811=CARTESIAN_POINT('Ctrl Pts',(17.57311479071,-1.09519924960301,122.909867480492));
#54812=CARTESIAN_POINT('Ctrl Pts',(18.164141477298,-1.4216002905349,122.950139633626));
#54813=CARTESIAN_POINT('Ctrl Pts',(18.9696230694653,-1.37578967503559,122.998239220247));
#54814=CARTESIAN_POINT('Ctrl Pts',(19.6239280630407,-0.910798341147612,
123.046108286732));
#54815=CARTESIAN_POINT('Ctrl Pts',(19.9291530020374,-0.172616375716822,
123.09374369598));
#54816=CARTESIAN_POINT('Ctrl Pts',(19.7954441463139,0.611082382716884,123.141142539284));
#54817=CARTESIAN_POINT('Ctrl Pts',(19.3559189355603,1.10190606845524,123.180442267812));
#54818=CARTESIAN_POINT('Ctrl Pts',(18.8899307018718,1.30920832624538,123.211761321333));
#54819=CARTESIAN_POINT('Ctrl Pts',(18.5263742070194,1.36095381325754,123.234322232426));
#54820=CARTESIAN_POINT('Ctrl Pts',(18.1775435791038,1.31674673854746,123.255962213161));
#54821=CARTESIAN_POINT('Ctrl Pts',(17.7593333092916,1.15328432565283,123.283597019229));
#54822=CARTESIAN_POINT('Ctrl Pts',(17.3398307943576,0.763703083387018,123.318019536972));
#54823=CARTESIAN_POINT('Ctrl Pts',(17.1587817619038,0.223479402479618,123.352279789599));
#54824=CARTESIAN_POINT('Ctrl Pts',(17.1817179901053,-0.21965108746767,123.379590264377));
#54825=CARTESIAN_POINT('Ctrl Pts',(17.3115269973765,-0.642795882173348,
123.406835412008));
#54826=CARTESIAN_POINT('Ctrl Pts',(17.6636164923134,-1.08399859950636,123.440769257244));
#54827=CARTESIAN_POINT('Ctrl Pts',(18.2330731955017,-1.32335926805016,123.477916162675));
#54828=CARTESIAN_POINT('Ctrl Pts',(18.7844078123242,-1.30212295801351,123.511542460656));
#54829=CARTESIAN_POINT('Ctrl Pts',(19.237729586223,-1.10435198427873,123.541695259909));
#54830=CARTESIAN_POINT('Ctrl Pts',(19.5861320260864,-0.755606676065294,
123.571737216082));
#54831=CARTESIAN_POINT('Ctrl Pts',(19.7823338166623,-0.305527423581674,
123.601668369117));
#54832=CARTESIAN_POINT('Ctrl Pts',(19.8004670543637,0.183419600739397,123.631488872885));
#54833=CARTESIAN_POINT('Ctrl Pts',(19.6393061251712,0.643384293867979,123.661198852101));
#54834=CARTESIAN_POINT('Ctrl Pts',(19.3752597155567,0.950094183277476,123.685865350904));
#54835=CARTESIAN_POINT('Ctrl Pts',(19.1084833026195,1.12428378128028,123.705543516584));
#54836=CARTESIAN_POINT('Ctrl Pts',(18.7659233778752,1.2668057521504,123.728458733859));
#54837=CARTESIAN_POINT('Ctrl Pts',(18.2510086222503,1.29223736298827,123.759451911037));
#54838=CARTESIAN_POINT('Ctrl Pts',(17.7649077298888,1.05761469451992,123.791914783735));
#54839=CARTESIAN_POINT('Ctrl Pts',(17.4792767223923,0.748967846692912,123.817788794064));
#54840=CARTESIAN_POINT('Ctrl Pts',(17.329077898565,0.47291654541466,123.837146270913));
#54841=CARTESIAN_POINT('Ctrl Pts',(17.2252669564987,0.0673940502346189,
123.862892562462));
#54842=CARTESIAN_POINT('Ctrl Pts',(17.2852604391398,-0.408471018364417,
123.89174995223));
#54843=CARTESIAN_POINT('Ctrl Pts',(17.5645778305311,-0.851824873362711,
123.923676060479));
#54844=CARTESIAN_POINT('Ctrl Pts',(17.9580568083485,-1.14230514083795,123.953496928898));
#54845=CARTESIAN_POINT('Ctrl Pts',(18.4529779621923,-1.26241680311112,123.984390222781));
#54846=CARTESIAN_POINT('Ctrl Pts',(18.9708103094374,-1.16668504108039,124.01634052165));
#54847=CARTESIAN_POINT('Ctrl Pts',(19.366630228591,-0.893819587524324,124.045509327258));
#54848=CARTESIAN_POINT('Ctrl Pts',(19.5610749691126,-0.608733295788248,
124.066648060783));
#54849=CARTESIAN_POINT('Ctrl Pts',(19.6687801575205,-0.346185382792283,
124.084228340358));
#54850=CARTESIAN_POINT('Ctrl Pts',(19.7217080738956,-0.0799700980385591,
124.100898985158));
#54851=CARTESIAN_POINT('Ctrl Pts',(19.6928905271332,0.260729788345592,124.121900560401));
#54852=CARTESIAN_POINT('Ctrl Pts',(19.5712258979927,0.579308030812463,124.142846849415));
#54853=CARTESIAN_POINT('Ctrl Pts',(19.3666436814044,0.851037647129537,124.16373812114));
#54854=CARTESIAN_POINT('Ctrl Pts',(19.0955647657873,1.05496769594385,124.184575019819));
#54855=CARTESIAN_POINT('Ctrl Pts',(18.8057448596413,1.16555851345604,124.203626193165));
#54856=CARTESIAN_POINT('Ctrl Pts',(18.5276285134945,1.19871213746157,124.220906472711));
#54857=CARTESIAN_POINT('Ctrl Pts',(18.1934516179046,1.16838186372108,124.241603159253));
#54858=CARTESIAN_POINT('Ctrl Pts',(17.8030055811293,1.00012280453531,124.267400343048));
#54859=CARTESIAN_POINT('Ctrl Pts',(17.4591443613634,0.625680307947734,124.298240874512));
#54860=CARTESIAN_POINT('Ctrl Pts',(17.298780306353,0.145317478363908,124.328967538828));
#54861=CARTESIAN_POINT('Ctrl Pts',(17.3484322588003,-0.356863082032555,
124.359582443048));
#54862=CARTESIAN_POINT('Ctrl Pts',(17.5979613332727,-0.793375340327835,
124.390087870071));
#54863=CARTESIAN_POINT('Ctrl Pts',(18.0025932240276,-1.08887194841174,124.420486124645));
#54864=CARTESIAN_POINT('Ctrl Pts',(18.4909367856316,-1.19296322240431,124.450779612303));
#54865=CARTESIAN_POINT('Ctrl Pts',(18.9775569396537,-1.08887495450386,124.480970793866));
#54866=CARTESIAN_POINT('Ctrl Pts',(19.3778957756401,-0.796079646301384,
124.511062207275));
#54867=CARTESIAN_POINT('Ctrl Pts',(19.6229378177282,-0.366699000956798,
124.541056454746));
#54868=CARTESIAN_POINT('Ctrl Pts',(19.6710819454008,0.123768576792137,124.570956206973));
#54869=CARTESIAN_POINT('Ctrl Pts',(19.5151825214616,0.589690167012718,124.6007641975));
#54870=CARTESIAN_POINT('Ctrl Pts',(19.1835730252442,0.950223228101631,124.63048322199));
#54871=CARTESIAN_POINT('Ctrl Pts',(18.7349333590939,1.14331075884206,124.660116135655));
#54872=CARTESIAN_POINT('Ctrl Pts',(18.2479281964886,1.13633797140025,124.689665853396));
#54873=CARTESIAN_POINT('Ctrl Pts',(17.8074430853533,0.931620578918509,124.719135346688));
#54874=CARTESIAN_POINT('Ctrl Pts',(17.4898217356975,0.565808383480578,124.748527641549));
#54875=CARTESIAN_POINT('Ctrl Pts',(17.3496657150365,0.103341142817895,124.777845815482));
#54876=CARTESIAN_POINT('Ctrl Pts',(17.4104730137507,-0.374876916066361,
124.807092995679));
#54877=CARTESIAN_POINT('Ctrl Pts',(17.6607161319537,-0.785598124605828,
124.836272358739));
#54878=CARTESIAN_POINT('Ctrl Pts',(18.0560104898594,-1.05768804968322,124.865387127451));
#54879=CARTESIAN_POINT('Ctrl Pts',(18.526967068725,-1.14441382762597,124.894440568606));
#54880=CARTESIAN_POINT('Ctrl Pts',(18.9913431026315,-1.0314475639091,124.923435989685));
#54881=CARTESIAN_POINT('Ctrl Pts',(19.3683685002177,-0.739218678075058,
124.952376736826));
#54882=CARTESIAN_POINT('Ctrl Pts',(19.5927584790688,-0.319231596033026,
124.981266194478));
#54883=CARTESIAN_POINT('Ctrl Pts',(19.6259873268813,0.154988889320898,125.010107782232));
#54884=CARTESIAN_POINT('Ctrl Pts',(19.4628825553958,0.60073609927402,125.038904952244));
#54885=CARTESIAN_POINT('Ctrl Pts',(19.1324150236228,0.940507944126239,125.067661186012));
#54886=CARTESIAN_POINT('Ctrl Pts',(18.6925674228159,1.11544599427495,125.09637999193));
#54887=CARTESIAN_POINT('Ctrl Pts',(18.220187394042,1.09550298745015,125.125064904932));
#54888=CARTESIAN_POINT('Ctrl Pts',(17.7975969993875,0.884587280323155,125.153719483493));
#54889=CARTESIAN_POINT('Ctrl Pts',(17.498285758871,0.519807155829135,125.182347306636));
#54890=CARTESIAN_POINT('Ctrl Pts',(17.3741663376746,0.0649598517818115,
125.210951970916));
#54891=CARTESIAN_POINT('Ctrl Pts',(17.4465962994511,-0.400595566794844,
125.239537087522));
#54892=CARTESIAN_POINT('Ctrl Pts',(17.702714511609,-0.795746326978485,125.268106281994));
#54893=CARTESIAN_POINT('Ctrl Pts',(18.0977185791255,-1.0517185595441,125.296663191365));
#54894=CARTESIAN_POINT('Ctrl Pts',(18.5626804301901,-1.12401300878258,125.325211460905));
#54895=CARTESIAN_POINT('Ctrl Pts',(19.0165404416634,-1.00011889006815,125.353754741278));
#54896=CARTESIAN_POINT('Ctrl Pts',(19.3801993580427,-0.701672757556588,
125.382296685284));
#54897=CARTESIAN_POINT('Ctrl Pts',(19.5902652601078,-0.280690435726507,
125.410840947633));
#54898=CARTESIAN_POINT('Ctrl Pts',(19.6100726418786,0.189473466106149,125.439391182285));
#54899=CARTESIAN_POINT('Ctrl Pts',(19.4360640155898,0.626871185373153,125.467951038996));
#54900=CARTESIAN_POINT('Ctrl Pts',(19.0984268547706,0.955204626959225,125.496524160671));
#54901=CARTESIAN_POINT('Ctrl Pts',(18.6558720003985,1.11709745415395,125.525114179851));
#54902=CARTESIAN_POINT('Ctrl Pts',(18.1854533778308,1.08409412045259,125.553724718471));
#54903=CARTESIAN_POINT('Ctrl Pts',(17.7691894439931,0.861647559159082,125.582359385548));
#54904=CARTESIAN_POINT('Ctrl Pts',(17.4798028826353,0.488224059886903,125.611021773455));
#54905=CARTESIAN_POINT('Ctrl Pts',(17.3680505492265,0.028671246726309,125.639715455637));
#54906=CARTESIAN_POINT('Ctrl Pts',(17.4538447442219,-0.437011366440344,
125.668443982813));
#54907=CARTESIAN_POINT('Ctrl Pts',(17.7227152954249,-0.827560849480737,
125.697210882868));
#54908=CARTESIAN_POINT('Ctrl Pts',(18.1282398436561,-1.07459346383945,125.726019658635));
#54909=CARTESIAN_POINT('Ctrl Pts',(18.6000357415897,-1.13454664475889,125.754873784372));
#54910=CARTESIAN_POINT('Ctrl Pts',(19.0559420543163,-0.996340771154775,
125.783776703428));
#54911=CARTESIAN_POINT('Ctrl Pts',(19.4162896725845,-0.683416566476759,
125.81273182463));
#54912=CARTESIAN_POINT('Ctrl Pts',(19.6177879629471,-0.249774365013851,
125.841742522047));
#54913=CARTESIAN_POINT('Ctrl Pts',(19.6246130111878,0.229318651775951,125.870812133036));
#54914=CARTESIAN_POINT('Ctrl Pts',(19.4347596171185,0.670358453751199,125.899943954864));
#54915=CARTESIAN_POINT('Ctrl Pts',(19.0805337627966,0.996122063548543,125.929141242478));
#54916=CARTESIAN_POINT('Ctrl Pts',(18.6230742316303,1.14915614382532,125.958407205093));
#54917=CARTESIAN_POINT('Ctrl Pts',(18.1418280742596,1.10188574238829,125.987745005866));
#54918=CARTESIAN_POINT('Ctrl Pts',(17.7207864948947,0.861567901278113,126.0171577601));
#54919=CARTESIAN_POINT('Ctrl Pts',(17.4338601270708,0.46920267105939,126.046648532321));
#54920=CARTESIAN_POINT('Ctrl Pts',(17.3319338973738,-0.00744028244417294,
126.076220333858));
#54921=CARTESIAN_POINT('Ctrl Pts',(17.4338635816607,-0.48549799831244,126.105876120044));
#54922=CARTESIAN_POINT('Ctrl Pts',(17.7230041681992,-0.881387583071317,
126.135618789578));
#54923=CARTESIAN_POINT('Ctrl Pts',(18.1499074077235,-1.12538888170401,126.16545118304));
#54924=CARTESIAN_POINT('Ctrl Pts',(18.6407553958162,-1.17389726511166,126.195376080285));
#54925=CARTESIAN_POINT('Ctrl Pts',(19.110096255813,-1.01719771547609,126.225396198108));
#54926=CARTESIAN_POINT('Ctrl Pts',(19.4756904241207,-0.681377009093858,
126.255514187869));
#54927=CARTESIAN_POINT('Ctrl Pts',(19.6728936838703,-0.224001716190088,
126.285732634629));
#54928=CARTESIAN_POINT('Ctrl Pts',(19.6660657931652,0.275726478226854,126.316054056017));
#54929=CARTESIAN_POINT('Ctrl Pts',(19.4549941835243,0.730659016820871,126.346480900112));
#54930=CARTESIAN_POINT('Ctrl Pts',(19.0751783442302,1.0608711604977,126.37701554289));
#54931=CARTESIAN_POINT('Ctrl Pts',(18.5918798815844,1.2076802849347,126.407660287092));
#54932=CARTESIAN_POINT('Ctrl Pts',(18.088932931197,1.14405521959446,126.438417359648));
#54933=CARTESIAN_POINT('Ctrl Pts',(17.6542245236157,0.879575635245244,126.469288913932));
#54934=CARTESIAN_POINT('Ctrl Pts',(17.3643636459841,0.459028112591109,126.5002770223));
#54935=CARTESIAN_POINT('Ctrl Pts',(17.2711939938056,-0.0451525818812408,
126.531383684238));
#54936=CARTESIAN_POINT('Ctrl Pts',(17.3925496972517,-0.545347189477102,
126.562610806295));
#54937=CARTESIAN_POINT('Ctrl Pts',(17.7088476742613,-0.953940800655802,
126.593960235512));
#54938=CARTESIAN_POINT('Ctrl Pts',(18.1662621639506,-1.19868197962896,126.625433694777));
#54939=CARTESIAN_POINT('Ctrl Pts',(18.6857870320997,-1.23538347152007,126.657032901379));
#54940=CARTESIAN_POINT('Ctrl Pts',(19.1770109198137,-1.05599536532106,126.688759339219));
#54941=CARTESIAN_POINT('Ctrl Pts',(19.4907918421248,-0.751068679762662,
126.715305466298));
#54942=CARTESIAN_POINT('Ctrl Pts',(19.6511793003569,-0.445245949338393,
126.73660731796));
#54943=CARTESIAN_POINT('Ctrl Pts',(19.7449908411919,-0.112183045382465,
126.757952973406));
#54944=CARTESIAN_POINT('Ctrl Pts',(19.7266891552073,0.328560035877289,126.784717043322));
#54945=CARTESIAN_POINT('Ctrl Pts',(19.4895319957358,0.804308800674381,126.816966807474));
#54946=CARTESIAN_POINT('Ctrl Pts',(19.077093245759,1.14310156338576,126.84935038456));
#54947=CARTESIAN_POINT('Ctrl Pts',(18.5600737160613,1.28447435350301,126.881868928107));
#54948=CARTESIAN_POINT('Ctrl Pts',(18.0282062679645,1.20200111344108,126.914523338728));
#54949=CARTESIAN_POINT('Ctrl Pts',(17.5745116558757,0.908257909117066,126.947314510873));
#54950=CARTESIAN_POINT('Ctrl Pts',(17.2791351203368,0.45292366127595,126.980243200589));
#54951=CARTESIAN_POINT('Ctrl Pts',(17.1951454991029,-0.0855934603369406,
127.013310094763));
#54952=CARTESIAN_POINT('Ctrl Pts',(17.3390382074035,-0.613655007911289,
127.046515773498));
#54953=CARTESIAN_POINT('Ctrl Pts',(17.6875198362081,-1.0386636260325,127.079860729247));
#54954=CARTESIAN_POINT('Ctrl Pts',(18.181260402214,-1.28529745768021,127.113345357394));
#54955=CARTESIAN_POINT('Ctrl Pts',(18.7349795771802,-1.30885272449037,127.146969959054));
#54956=CARTESIAN_POINT('Ctrl Pts',(19.2521732788533,-1.10333621731152,127.180734741782));
#54957=CARTESIAN_POINT('Ctrl Pts',(19.6419290401089,-0.702841603331218,
127.214639813623));
#54958=CARTESIAN_POINT('Ctrl Pts',(19.8349060622305,-0.175911321282134,
127.248685196296));
#54959=CARTESIAN_POINT('Ctrl Pts',(19.7956686304382,0.386187668303325,127.282870799533));
#54960=CARTESIAN_POINT('Ctrl Pts',(19.5291784681672,0.885271812874289,127.317196470363));
#54961=CARTESIAN_POINT('Ctrl Pts',(19.0802611718389,1.23339149582639,127.351661899081));
#54962=CARTESIAN_POINT('Ctrl Pts',(18.5260767506703,1.3683341345413,127.386266797367));
#54963=CARTESIAN_POINT('Ctrl Pts',(17.9628555970782,1.26473704354384,127.421010556494));
#54964=CARTESIAN_POINT('Ctrl Pts',(17.4891965904045,0.938837633413158,127.455892935242));
#54965=CARTESIAN_POINT('Ctrl Pts',(17.1887742378464,0.445956210839747,127.490912627166));
#54966=CARTESIAN_POINT('Ctrl Pts',(17.1155871988033,-0.128878759482379,
127.526070226388));
#54967=CARTESIAN_POINT('Ctrl Pts',(17.2842442567953,-0.6856327348833,127.561362414191));
#54968=CARTESIAN_POINT('Ctrl Pts',(17.6669802913474,-1.12658965503124,127.596792558688));
#54969=CARTESIAN_POINT('Ctrl Pts',(18.1986315984172,-1.37375997079926,127.632352264871));
#54970=CARTESIAN_POINT('Ctrl Pts',(18.7867735556596,-1.38213293233228,127.668054104116));
#54971=CARTESIAN_POINT('Ctrl Pts',(19.3292837483826,-1.1488895601724,127.7038701522));
#54972=CARTESIAN_POINT('Ctrl Pts',(19.7308757076997,-0.712514467722855,
127.739846925354));
#54973=CARTESIAN_POINT('Ctrl Pts',(19.918472262676,-0.148383127901019,127.775918194433));
#54974=CARTESIAN_POINT('Ctrl Pts',(19.8719539849658,0.345937981508172,127.806087591881));
#54975=CARTESIAN_POINT('Ctrl Pts',(19.7127708262951,0.70607801146938,127.830337982654));
#54976=CARTESIAN_POINT('Ctrl Pts',(19.5386023042488,0.945577081476424,127.848504632835));
#54977=CARTESIAN_POINT('Ctrl Pts',(19.3198906328131,1.14364161409795,127.866689814571));
#54978=CARTESIAN_POINT('Ctrl Pts',(19.0678313013017,1.2914197254424,127.884957912083));
#54979=CARTESIAN_POINT('Ctrl Pts',(18.7904620761009,1.38257654608712,127.903291001622));
#54980=CARTESIAN_POINT('Ctrl Pts',(18.5922400986655,1.40380723379247,127.915441694516));
#54981=CARTESIAN_POINT('Ctrl Pts',(18.4903128297246,1.40466511306502,127.92147546947));
#54982=CARTESIAN_POINT('Ctrl Pts',(18.4897811044666,1.46372061123931,112.750652102996));
#54983=CARTESIAN_POINT('Ctrl Pts',(18.3305659168598,1.46238056347085,112.760077143174));
#54984=CARTESIAN_POINT('Ctrl Pts',(18.125793406092,1.42986577729673,112.772844964474));
#54985=CARTESIAN_POINT('Ctrl Pts',(17.8412845056959,1.31915463921368,112.792067023561));
#54986=CARTESIAN_POINT('Ctrl Pts',(17.6209713973646,1.1900784659798,112.80803570717));
#54987=CARTESIAN_POINT('Ctrl Pts',(17.3911882883068,0.981968016985861,112.827140907135));
#54988=CARTESIAN_POINT('Ctrl Pts',(17.2073171982579,0.729393018088631,112.846306361443));
#54989=CARTESIAN_POINT('Ctrl Pts',(17.0384351507011,0.347283122277831,112.872036780446));
#54990=CARTESIAN_POINT('Ctrl Pts',(16.9886748804566,-0.178292311259029,
112.904115521818));
#54991=CARTESIAN_POINT('Ctrl Pts',(17.1889316142324,-0.781749189448536,
112.942692992335));
#54992=CARTESIAN_POINT('Ctrl Pts',(17.6209789196198,-1.25188558375487,112.981429235051));
#54993=CARTESIAN_POINT('Ctrl Pts',(18.2079353711238,-1.5045708835093,113.020185323627));
#54994=CARTESIAN_POINT('Ctrl Pts',(18.8482829043636,-1.49590845051623,113.05905837792));
#54995=CARTESIAN_POINT('Ctrl Pts',(19.4304958659054,-1.22560756348276,113.097987904393));
#54996=CARTESIAN_POINT('Ctrl Pts',(19.8522306332794,-0.740339244651456,
113.137001694574));
#54997=CARTESIAN_POINT('Ctrl Pts',(20.0393256416704,-0.123981173335954,
113.176077472417));
#54998=CARTESIAN_POINT('Ctrl Pts',(19.9582169960145,0.516105276266115,113.215223894842));
#54999=CARTESIAN_POINT('Ctrl Pts',(19.6221913410372,1.06810878123685,113.254429998878));
#55000=CARTESIAN_POINT('Ctrl Pts',(19.0892198662845,1.43526754494134,113.293696217054));
#55001=CARTESIAN_POINT('Ctrl Pts',(18.4518647573978,1.55287245970027,113.333016998286));
#55002=CARTESIAN_POINT('Ctrl Pts',(17.8212439746614,1.39968964394208,113.372389563759));
#55003=CARTESIAN_POINT('Ctrl Pts',(17.3075692374066,1.00180608691406,113.411809801272));
#55004=CARTESIAN_POINT('Ctrl Pts',(17.000873284185,0.42817270456625,113.451274197287));
#55005=CARTESIAN_POINT('Ctrl Pts',(16.9551821048933,-0.22136165817646,113.49077889699));
#55006=CARTESIAN_POINT('Ctrl Pts',(17.1789901136725,-0.833471727017209,
113.530320136614));
#55007=CARTESIAN_POINT('Ctrl Pts',(17.6336675842817,-1.30116454392376,113.569894150434));
#55008=CARTESIAN_POINT('Ctrl Pts',(18.2401696678772,-1.54252645140642,113.60949699668));
#55009=CARTESIAN_POINT('Ctrl Pts',(18.8927538416101,-1.51509157179902,113.64912505003));
#55010=CARTESIAN_POINT('Ctrl Pts',(19.4775429231303,-1.22333733766362,113.68877409611));
#55011=CARTESIAN_POINT('Ctrl Pts',(19.8923283686142,-0.717952641965618,
113.728440607448));
#55012=CARTESIAN_POINT('Ctrl Pts',(20.0645752690355,-0.0870289267892908,
113.768120453468));
#55013=CARTESIAN_POINT('Ctrl Pts',(19.9640685005371,0.559400324613147,113.807809828465));
#55014=CARTESIAN_POINT('Ctrl Pts',(19.6082418329362,1.10844386956989,113.847504852794));
#55015=CARTESIAN_POINT('Ctrl Pts',(19.0591636449125,1.46432165094386,113.887201491434));
#55016=CARTESIAN_POINT('Ctrl Pts',(18.5204080967549,1.54803402763228,113.920280307134));
#55017=CARTESIAN_POINT('Ctrl Pts',(18.0971213830127,1.47872672380361,113.946740145263));
#55018=CARTESIAN_POINT('Ctrl Pts',(17.6973555935897,1.32336298729138,113.973197285216));
#55019=CARTESIAN_POINT('Ctrl Pts',(17.2760459903937,0.977663903758167,114.006262645077));
#55020=CARTESIAN_POINT('Ctrl Pts',(16.9841963480954,0.392626824069597,114.045926931518));
#55021=CARTESIAN_POINT('Ctrl Pts',(16.9567342727123,-0.260253158742564,
114.085573459637));
#55022=CARTESIAN_POINT('Ctrl Pts',(17.1982278925264,-0.867095767455903,
114.125198265763));
#55023=CARTESIAN_POINT('Ctrl Pts',(17.6662113538874,-1.32206355425537,114.164797473269));
#55024=CARTESIAN_POINT('Ctrl Pts',(18.2787609337407,-1.54603968390748,114.20436727098));
#55025=CARTESIAN_POINT('Ctrl Pts',(18.9288172222856,-1.50031607897088,114.243903822103));
#55026=CARTESIAN_POINT('Ctrl Pts',(19.5029618017992,-1.19335509858773,114.283403282528));
#55027=CARTESIAN_POINT('Ctrl Pts',(19.901237024244,-0.679182233478761,114.322861954074));
#55028=CARTESIAN_POINT('Ctrl Pts',(20.0545852373889,-0.047903393129132,
114.362275981028));
#55029=CARTESIAN_POINT('Ctrl Pts',(19.9368537301759,0.590185965224506,114.40164173171));
#55030=CARTESIAN_POINT('Ctrl Pts',(19.5692562741686,1.12380691439424,114.440955473318));
#55031=CARTESIAN_POINT('Ctrl Pts',(19.0165331060083,1.46027294727139,114.480213553625));
#55032=CARTESIAN_POINT('Ctrl Pts',(18.375563704988,1.54150263789562,114.519412367348));
#55033=CARTESIAN_POINT('Ctrl Pts',(17.7583100289019,1.35414393426942,114.5585483306));
#55034=CARTESIAN_POINT('Ctrl Pts',(17.2722472743633,0.931726226959488,114.597617913046));
#55035=CARTESIAN_POINT('Ctrl Pts',(17.001603535348,0.348658869884238,114.636617630877));
#55036=CARTESIAN_POINT('Ctrl Pts',(16.9927335372165,-0.292881472094132,
114.675544031198));
#55037=CARTESIAN_POINT('Ctrl Pts',(17.2461846841767,-0.880944809491311,
114.714393746167));
#55038=CARTESIAN_POINT('Ctrl Pts',(17.7167374067633,-1.31327003087369,114.753163390647));
#55039=CARTESIAN_POINT('Ctrl Pts',(18.3215624607069,-1.51531409642752,114.791849768283));
#55040=CARTESIAN_POINT('Ctrl Pts',(18.8491562346418,-1.46314533152096,114.824016194578));
#55041=CARTESIAN_POINT('Ctrl Pts',(19.2302731192541,-1.29534293564721,114.849704556036));
#55042=CARTESIAN_POINT('Ctrl Pts',(19.5680201993842,-1.05257590633892,114.87536252632));
#55043=CARTESIAN_POINT('Ctrl Pts',(19.8793194019256,-0.626525224187843,
114.907376795667));
#55044=CARTESIAN_POINT('Ctrl Pts',(20.0110263896328,-0.00874579380907211,
114.945698209434));
#55045=CARTESIAN_POINT('Ctrl Pts',(19.8793086186887,0.607314790118817,114.983920680183));
#55046=CARTESIAN_POINT('Ctrl Pts',(19.5084111324286,1.11450997297525,115.022041429527));
#55047=CARTESIAN_POINT('Ctrl Pts',(18.964206619524,1.42510388242354,115.060057532941));
#55048=CARTESIAN_POINT('Ctrl Pts',(18.3423681279344,1.48616747636079,115.09796627472));
#55049=CARTESIAN_POINT('Ctrl Pts',(17.751531483489,1.28847084357424,115.135764893611));
#55050=CARTESIAN_POINT('Ctrl Pts',(17.2943774305468,0.86797834662618,115.173450851635));
#55051=CARTESIAN_POINT('Ctrl Pts',(17.0495318909918,0.299122922775257,115.211021448735));
#55052=CARTESIAN_POINT('Ctrl Pts',(17.0575062136741,-0.249489879927474,
115.244313053249));
#55053=CARTESIAN_POINT('Ctrl Pts',(17.2265723807848,-0.691296868335461,
115.273365038483));
#55054=CARTESIAN_POINT('Ctrl Pts',(17.4088824641546,-0.933730795312457,
115.292001216897));
#55055=CARTESIAN_POINT('Ctrl Pts',(17.5553960293834,-1.07013569528572,115.304407717233));
#55056=CARTESIAN_POINT('Ctrl Pts',(17.6331027617258,-1.1330673537071,115.310607741085));
#55057=CARTESIAN_POINT('Ctrl Pts',(17.7150593184202,-1.19031116283603,115.31680421033));
#55058=CARTESIAN_POINT('Ctrl Pts',(17.8863953605569,-1.29308480412215,115.329190651479));
#55059=CARTESIAN_POINT('Ctrl Pts',(18.1686370240243,-1.40074582057259,115.347743492983));
#55060=CARTESIAN_POINT('Ctrl Pts',(18.5690163480438,-1.43447133078092,115.372425439255));
#55061=CARTESIAN_POINT('Ctrl Pts',(18.9622857850623,-1.356175093929,115.397050104753));
#55062=CARTESIAN_POINT('Ctrl Pts',(19.3174893024164,-1.17255993098256,115.421618022958));
#55063=CARTESIAN_POINT('Ctrl Pts',(19.6076271996196,-0.898329980683078,
115.446127643009));
#55064=CARTESIAN_POINT('Ctrl Pts',(19.8094258000695,-0.55549666470966,115.470579183103));
#55065=CARTESIAN_POINT('Ctrl Pts',(19.9426156970628,-0.0425558216700198,
115.503102315118));
#55066=CARTESIAN_POINT('Ctrl Pts',(19.8514135668701,0.492534124086972,115.535506467039));
#55067=CARTESIAN_POINT('Ctrl Pts',(19.5947255019288,0.874650732212783,115.563754295808));
#55068=CARTESIAN_POINT('Ctrl Pts',(19.4083996970038,1.05617431733856,115.579865220324));
#55069=CARTESIAN_POINT('Ctrl Pts',(19.1982429433524,1.2096203916672,115.595955885261));
#55070=CARTESIAN_POINT('Ctrl Pts',(18.989589114405,1.30306979403804,115.610008424767));
#55071=CARTESIAN_POINT('Ctrl Pts',(18.8013128243347,1.3501360194407,115.622033854083));
#55072=CARTESIAN_POINT('Ctrl Pts',(18.7059043584766,1.3670507590569,115.628042775347));
#55073=CARTESIAN_POINT('Ctrl Pts',(18.6256141605857,1.37555385934589,115.633046937773));
#55074=CARTESIAN_POINT('Ctrl Pts',(18.561178149311,1.37888388996972,115.637048396594));
#55075=CARTESIAN_POINT('Ctrl Pts',(18.2997000866567,1.38388444692226,115.65327107495));
#55076=CARTESIAN_POINT('Ctrl Pts',(17.8263490130143,1.2627382748751,115.682643583081));
#55077=CARTESIAN_POINT('Ctrl Pts',(17.424914370665,0.890032416107338,115.715592608078));
#55078=CARTESIAN_POINT('Ctrl Pts',(17.2467539250202,0.554805958801192,115.739053158468));
#55079=CARTESIAN_POINT('Ctrl Pts',(17.1861924514361,0.375353183495959,115.750764696338));
#55080=CARTESIAN_POINT('Ctrl Pts',(17.1564555797285,0.227296192343728,115.760122604584));
#55081=CARTESIAN_POINT('Ctrl Pts',(17.120967866444,-0.0723899313699495,
115.778823626985));
#55082=CARTESIAN_POINT('Ctrl Pts',(17.2088578800484,-0.568527186055847,
115.809127002241));
#55083=CARTESIAN_POINT('Ctrl Pts',(17.6421591341182,-1.11134999926644,115.850880748309));
#55084=CARTESIAN_POINT('Ctrl Pts',(18.2259638545534,-1.35677182815753,115.888965856558));
#55085=CARTESIAN_POINT('Ctrl Pts',(18.7911845995156,-1.3349800129774,115.923437330073));
#55086=CARTESIAN_POINT('Ctrl Pts',(19.255812563341,-1.13226888716917,115.954344416483));
#55087=CARTESIAN_POINT('Ctrl Pts',(19.6129288887079,-0.774826552610854,
115.985133850421));
#55088=CARTESIAN_POINT('Ctrl Pts',(19.7803871051415,-0.390503239648824,
116.010693444063));
#55089=CARTESIAN_POINT('Ctrl Pts',(19.8232900466592,-0.0631136113716338,
116.031081930678));
#55090=CARTESIAN_POINT('Ctrl Pts',(19.8094753804474,0.18357055636264,116.046343784384));
#55091=CARTESIAN_POINT('Ctrl Pts',(19.759963513967,0.383089889208843,116.059037249292));
#55092=CARTESIAN_POINT('Ctrl Pts',(19.6987167583072,0.534822847653917,116.069177221446));
#55093=CARTESIAN_POINT('Ctrl Pts',(19.5862796684731,0.752779622550448,116.084372388956));
#55094=CARTESIAN_POINT('Ctrl Pts',(19.3428646912038,1.03541739212991,116.107109487966));
#55095=CARTESIAN_POINT('Ctrl Pts',(18.9047700381786,1.26675694584353,116.137306977485));
#55096=CARTESIAN_POINT('Ctrl Pts',(18.4143705145873,1.32182474021267,116.167385713619));
#55097=CARTESIAN_POINT('Ctrl Pts',(18.0583443434444,1.22628304283745,116.189855803588));
#55098=CARTESIAN_POINT('Ctrl Pts',(17.8462515090041,1.11147637938476,116.204798779312));
#55099=CARTESIAN_POINT('Ctrl Pts',(17.7127049673212,1.02227301661988,116.214750887188));
#55100=CARTESIAN_POINT('Ctrl Pts',(17.5026882046262,0.834640398251948,116.232141219153));
#55101=CARTESIAN_POINT('Ctrl Pts',(17.3621175549714,0.611099620430629,116.248241208803));
#55102=CARTESIAN_POINT('Ctrl Pts',(17.2938429805976,0.423855467682653,116.260598155883));
#55103=CARTESIAN_POINT('Ctrl Pts',(17.2759262214136,0.366868133270414,116.264303404854));
#55104=CARTESIAN_POINT('Ctrl Pts',(17.2607570337696,0.309096675662953,116.268006801496));
#55105=CARTESIAN_POINT('Ctrl Pts',(17.248292579062,0.250729697737948,116.271708356085));
#55106=CARTESIAN_POINT('Ctrl Pts',(17.2385564436958,0.191862855691203,116.275408062101));
#55107=CARTESIAN_POINT('Ctrl Pts',(17.2293276540802,0.112898847873108,116.280338540313));
#55108=CARTESIAN_POINT('Ctrl Pts',(17.2189539465842,-0.105526562397861,
116.293887185899));
#55109=CARTESIAN_POINT('Ctrl Pts',(17.2865569346428,-0.46198587121534,116.316002575039));
#55110=CARTESIAN_POINT('Ctrl Pts',(17.5430611832942,-0.869881342426196,
116.345372133543));
#55111=CARTESIAN_POINT('Ctrl Pts',(17.9292997327579,-1.15471831367284,116.374624691353));
#55112=CARTESIAN_POINT('Ctrl Pts',(18.3910824032975,-1.27825989559717,116.403760596127));
#55113=CARTESIAN_POINT('Ctrl Pts',(18.8641367580531,-1.22478453810117,116.432780512622));
#55114=CARTESIAN_POINT('Ctrl Pts',(19.2833643020942,-1.00303724998616,116.461684909985));
#55115=CARTESIAN_POINT('Ctrl Pts',(19.5227871655153,-0.724505149715909,
116.484076990982));
#55116=CARTESIAN_POINT('Ctrl Pts',(19.6374182547927,-0.493683341710843,
116.500028892448));
#55117=CARTESIAN_POINT('Ctrl Pts',(19.7052765909381,-0.299410071500717,
116.512773803769));
#55118=CARTESIAN_POINT('Ctrl Pts',(19.7596827729301,0.0582630911084101,
116.535032914344));
#55119=CARTESIAN_POINT('Ctrl Pts',(19.6422842103624,0.571651584928872,116.566706373337));
#55120=CARTESIAN_POINT('Ctrl Pts',(19.2257653211103,1.04290863492653,116.604515658408));
#55121=CARTESIAN_POINT('Ctrl Pts',(18.6378872911912,1.25645660057682,116.642128600935));
#55122=CARTESIAN_POINT('Ctrl Pts',(18.0225041260444,1.16333115570126,116.679547542631));
#55123=CARTESIAN_POINT('Ctrl Pts',(17.601202923633,0.843680448939181,116.71134621701));
#55124=CARTESIAN_POINT('Ctrl Pts',(17.3846691880087,0.474999085705099,116.737611476145));
#55125=CARTESIAN_POINT('Ctrl Pts',(17.2710407476065,0.0379276543343812,
116.765343094364));
#55126=CARTESIAN_POINT('Ctrl Pts',(17.3682734853946,-0.532588354634737,
116.799861144831));
#55127=CARTESIAN_POINT('Ctrl Pts',(17.8290624618527,-1.0473695001524,116.841053271886));
#55128=CARTESIAN_POINT('Ctrl Pts',(18.4893639542835,-1.23701137347387,116.88202069821));
#55129=CARTESIAN_POINT('Ctrl Pts',(19.1457977829931,-1.04739610347266,116.922768533721));
#55130=CARTESIAN_POINT('Ctrl Pts',(19.5985173054551,-0.540139679709388,
116.96330233943));
#55131=CARTESIAN_POINT('Ctrl Pts',(19.6922387328967,0.0153796368980274,
116.996906606869));
#55132=CARTESIAN_POINT('Ctrl Pts',(19.5824301046536,0.437440499685657,117.02368902324));
#55133=CARTESIAN_POINT('Ctrl Pts',(19.4170516191088,0.71855847802177,117.043725662408));
#55134=CARTESIAN_POINT('Ctrl Pts',(19.1802672799888,0.941766571567522,117.063713592448));
#55135=CARTESIAN_POINT('Ctrl Pts',(18.7959731089366,1.14115562743497,117.090299363394));
#55136=CARTESIAN_POINT('Ctrl Pts',(18.2416584714609,1.17212298152654,117.123413149607));
#55137=CARTESIAN_POINT('Ctrl Pts',(17.6612476425556,0.85078765321395,117.16296619688));
#55138=CARTESIAN_POINT('Ctrl Pts',(17.3422279633976,0.272702222384503,117.202342864818));
#55139=CARTESIAN_POINT('Ctrl Pts',(17.3794635084803,-0.383772473351894,
117.241550095212));
#55140=CARTESIAN_POINT('Ctrl Pts',(17.7586839982553,-0.91755328435359,117.280595232539));
#55141=CARTESIAN_POINT('Ctrl Pts',(18.3613572107628,-1.16681408332463,117.319485706597));
#55142=CARTESIAN_POINT('Ctrl Pts',(19.0018467679279,-1.05764318469179,117.358229192413));
#55143=CARTESIAN_POINT('Ctrl Pts',(19.4843526169941,-0.62602185554045,117.396833518546));
#55144=CARTESIAN_POINT('Ctrl Pts',(19.6626760875841,-0.00596355109428755,
117.435306690535));
#55145=CARTESIAN_POINT('Ctrl Pts',(19.4843653350139,0.611949745664865,117.473656858281));
#55146=CARTESIAN_POINT('Ctrl Pts',(19.006082836089,1.03901891538125,117.511892338249));
#55147=CARTESIAN_POINT('Ctrl Pts',(18.3756555473465,1.14588845941846,117.550021578917));
#55148=CARTESIAN_POINT('Ctrl Pts',(17.7865034506633,0.901614741639774,117.588053147374));
#55149=CARTESIAN_POINT('Ctrl Pts',(17.4184650221663,0.38256549210635,117.625995735236));
#55150=CARTESIAN_POINT('Ctrl Pts',(17.3830379091306,-0.251394920777476,
117.663858153122));
#55151=CARTESIAN_POINT('Ctrl Pts',(17.6897416212228,-0.805988837816665,
117.701649288551));
#55152=CARTESIAN_POINT('Ctrl Pts',(18.2435530961125,-1.11192915841498,117.739378125066));
#55153=CARTESIAN_POINT('Ctrl Pts',(18.8743941085538,-1.07637392924317,117.777053713013));
#55154=CARTESIAN_POINT('Ctrl Pts',(19.3889681580371,-0.711139819413866,
117.814685205125));
#55155=CARTESIAN_POINT('Ctrl Pts',(19.6302776223641,-0.128565949173179,
117.852281715748));
#55156=CARTESIAN_POINT('Ctrl Pts',(19.5421188945232,0.388966926266299,117.883590757787));
#55157=CARTESIAN_POINT('Ctrl Pts',(19.3148713652829,0.727405617431935,117.908629650839));
#55158=CARTESIAN_POINT('Ctrl Pts',(19.0040420734761,0.991073319636765,117.933664807893));
#55159=CARTESIAN_POINT('Ctrl Pts',(18.4999415631754,1.13648535076679,117.964953921654));
#55160=CARTESIAN_POINT('Ctrl Pts',(17.8947899695678,0.96208712009206,118.002503188243));
#55161=CARTESIAN_POINT('Ctrl Pts',(17.4750732454252,0.492492667183828,118.040063661805));
#55162=CARTESIAN_POINT('Ctrl Pts',(17.3694300523301,-0.128850031555598,
118.077644813751));
#55163=CARTESIAN_POINT('Ctrl Pts',(17.6107331136891,-0.711582450772628,
118.115255756409));
#55164=CARTESIAN_POINT('Ctrl Pts',(18.125603119214,-1.07704534040567,118.152905757722));
#55165=CARTESIAN_POINT('Ctrl Pts',(18.7567934833813,-1.1125997163517,118.190603932222));
#55166=CARTESIAN_POINT('Ctrl Pts',(19.3110204717537,-0.806486790888208,
118.228359414069));
#55167=CARTESIAN_POINT('Ctrl Pts',(19.6179609922649,-0.25139504372414,118.266181161867));
#55168=CARTESIAN_POINT('Ctrl Pts',(19.5825391926542,0.383053875326996,118.304078231522));
#55169=CARTESIAN_POINT('Ctrl Pts',(19.2140816405097,0.902802898927527,118.342059291419));
#55170=CARTESIAN_POINT('Ctrl Pts',(18.7226880201779,1.10634814765537,118.373787735995));
#55171=CARTESIAN_POINT('Ctrl Pts',(18.3086085930042,1.09397848195709,118.39922099189));
#55172=CARTESIAN_POINT('Ctrl Pts',(18.0123540634614,0.999893884623254,118.418322678652));
#55173=CARTESIAN_POINT('Ctrl Pts',(17.7533626515011,0.82671918127196,118.437451496774));
#55174=CARTESIAN_POINT('Ctrl Pts',(17.5521199768519,0.588537547192838,118.456609257602));
#55175=CARTESIAN_POINT('Ctrl Pts',(17.4244911269899,0.303352454653029,118.475796244556));
#55176=CARTESIAN_POINT('Ctrl Pts',(17.3807273267954,-0.00639979916192339,
118.495014194405));
#55177=CARTESIAN_POINT('Ctrl Pts',(17.4244813580664,-0.316785015260581,
118.514263485987));
#55178=CARTESIAN_POINT('Ctrl Pts',(17.5313433203722,-0.555495775472718,
118.530332161233));
#55179=CARTESIAN_POINT('Ctrl Pts',(17.6540773517199,-0.723534213278567,
118.543203421388));
#55180=CARTESIAN_POINT('Ctrl Pts',(17.7992754119155,-0.872605010499798,
118.556086803096));
#55181=CARTESIAN_POINT('Ctrl Pts',(18.1045650757977,-1.07757525544991,118.578662058107));
#55182=CARTESIAN_POINT('Ctrl Pts',(18.6388883319623,-1.16886260969525,118.611002224315));
#55183=CARTESIAN_POINT('Ctrl Pts',(19.2429199720252,-0.91905243268689,118.649960624054));
#55184=CARTESIAN_POINT('Ctrl Pts',(19.5591656207873,-0.47353880214557,118.682557494984));
#55185=CARTESIAN_POINT('Ctrl Pts',(19.6312341819153,-0.107637891392649,
118.705448035791));
#55186=CARTESIAN_POINT('Ctrl Pts',(19.6284150057505,0.103886268314961,118.718548975396));
#55187=CARTESIAN_POINT('Ctrl Pts',(19.5958932860597,0.313538506666422,118.731664743549));
#55188=CARTESIAN_POINT('Ctrl Pts',(19.5004242033217,0.563000832640334,118.748085947437));
#55189=CARTESIAN_POINT('Ctrl Pts',(19.2432455304437,0.90628492536278,118.774418879784));
#55190=CARTESIAN_POINT('Ctrl Pts',(18.7589006628383,1.17453438898742,118.807447049227));
#55191=CARTESIAN_POINT('Ctrl Pts',(18.0920378754068,1.13752775310542,118.847267321706));
#55192=CARTESIAN_POINT('Ctrl Pts',(17.5444894219634,0.749580520515216,118.887280294004));
#55193=CARTESIAN_POINT('Ctrl Pts',(17.3292362808046,0.230633636407774,118.920790576476));
#55194=CARTESIAN_POINT('Ctrl Pts',(17.3423520957121,-0.207489759410931,
118.94770109744));
#55195=CARTESIAN_POINT('Ctrl Pts',(17.4252619681566,-0.469003909932179,
118.96456394793));
#55196=CARTESIAN_POINT('Ctrl Pts',(17.5203149088613,-0.634993651085502,
118.976390606938));
#55197=CARTESIAN_POINT('Ctrl Pts',(17.583983658906,-0.723534404469764,118.983155440389));
#55198=CARTESIAN_POINT('Ctrl Pts',(17.6538927305433,-0.807470935982133,
118.98992472633));
#55199=CARTESIAN_POINT('Ctrl Pts',(17.7520083028492,-0.902883777274666,
118.998394938564));
#55200=CARTESIAN_POINT('Ctrl Pts',(17.9290489907581,-1.0323314088204,119.01196453638));
#55201=CARTESIAN_POINT('Ctrl Pts',(18.1815801842383,-1.14541285633602,119.028960890958));
#55202=CARTESIAN_POINT('Ctrl Pts',(18.5112600172864,-1.19201555623084,119.049410990679));
#55203=CARTESIAN_POINT('Ctrl Pts',(18.8418328477004,-1.14540690441618,119.06991680109));
#55204=CARTESIAN_POINT('Ctrl Pts',(19.1474267825692,-1.00874033585996,119.090478520413));
#55205=CARTESIAN_POINT('Ctrl Pts',(19.4039443073445,-0.79220717736026,119.111097145673));
#55206=CARTESIAN_POINT('Ctrl Pts',(19.5910119718638,-0.51236647902462,119.131772830806));
#55207=CARTESIAN_POINT('Ctrl Pts',(19.6935905299409,-0.190752836459021,
119.152506800925));
#55208=CARTESIAN_POINT('Ctrl Pts',(19.7031388477895,0.147604935192541,119.173298766399));
#55209=CARTESIAN_POINT('Ctrl Pts',(19.6325566841645,0.421577620165869,119.190675097676));
#55210=CARTESIAN_POINT('Ctrl Pts',(19.5319409006659,0.622959778725234,119.204605562775));
#55211=CARTESIAN_POINT('Ctrl Pts',(19.3723111918508,0.855222362722365,119.22204381589));
#55212=CARTESIAN_POINT('Ctrl Pts',(19.0605236648718,1.11137648097883,119.24652741901));
#55213=CARTESIAN_POINT('Ctrl Pts',(18.557841901936,1.24883064038303,119.278143157038));
#55214=CARTESIAN_POINT('Ctrl Pts',(18.0406440600076,1.16864301673205,119.309897324764));
#55215=CARTESIAN_POINT('Ctrl Pts',(17.5993534519754,0.882949483972891,119.341791378035));
#55216=CARTESIAN_POINT('Ctrl Pts',(17.3119750925068,0.439968778678807,119.373826695856));
#55217=CARTESIAN_POINT('Ctrl Pts',(17.2302408898466,-0.0840529947305273,
119.406004587621));
#55218=CARTESIAN_POINT('Ctrl Pts',(17.3702629976844,-0.598088729393078,
119.438326182762));
#55219=CARTESIAN_POINT('Ctrl Pts',(17.6530460544461,-0.942889577582773,
119.465381607609));
#55220=CARTESIAN_POINT('Ctrl Pts',(17.9499828766226,-1.13203718581272,119.487098771073));
#55221=CARTESIAN_POINT('Ctrl Pts',(18.2803607508843,-1.25590365191542,119.508864774012));
#55222=CARTESIAN_POINT('Ctrl Pts',(18.729892524166,-1.27510737942024,119.536163929142));
#55223=CARTESIAN_POINT('Ctrl Pts',(19.2339592933469,-1.07479600420633,119.569070444908));
#55224=CARTESIAN_POINT('Ctrl Pts',(19.6139473273938,-0.684379105992577,
119.602125158036));
#55225=CARTESIAN_POINT('Ctrl Pts',(19.8021770921533,-0.170476841564033,
119.635328673285));
#55226=CARTESIAN_POINT('Ctrl Pts',(19.7639134649815,0.377926935064038,119.668681477351));
#55227=CARTESIAN_POINT('Ctrl Pts',(19.503839851328,0.865051934686931,119.70218396231));
#55228=CARTESIAN_POINT('Ctrl Pts',(19.0655180465322,1.20498508477827,119.735836419624));
#55229=CARTESIAN_POINT('Ctrl Pts',(18.524202098875,1.33680965848674,119.76963902964));
#55230=CARTESIAN_POINT('Ctrl Pts',(17.973771139484,1.23562343421845,119.803591891955));
#55231=CARTESIAN_POINT('Ctrl Pts',(17.5879069760352,0.970077900984119,119.832011116879));
#55232=CARTESIAN_POINT('Ctrl Pts',(17.3637280416863,0.675990163767077,119.85482156895));
#55233=CARTESIAN_POINT('Ctrl Pts',(17.2049255398143,0.341169720857323,119.877682007301));
#55234=CARTESIAN_POINT('Ctrl Pts',(17.1451722184405,-0.127573629778547,
119.906351243673));
#55235=CARTESIAN_POINT('Ctrl Pts',(17.310261401612,-0.672648178521142,119.940903882702));
#55236=CARTESIAN_POINT('Ctrl Pts',(17.6851761255204,-1.10460181805881,119.975605671829));
#55237=CARTESIAN_POINT('Ctrl Pts',(18.2060526856434,-1.34679126014451,120.0104560752));
#55238=CARTESIAN_POINT('Ctrl Pts',(18.7828550078472,-1.35513556170808,120.045454472915));
#55239=CARTESIAN_POINT('Ctrl Pts',(19.3149902028912,-1.12620240023457,120.08060013599));
#55240=CARTESIAN_POINT('Ctrl Pts',(19.7088387709082,-0.69810855233221,120.115892239948));
#55241=CARTESIAN_POINT('Ctrl Pts',(19.8942441582493,-0.144212137261873,
120.151329858863));
#55242=CARTESIAN_POINT('Ctrl Pts',(19.8370075803674,0.439473461448282,120.186911969597));
#55243=CARTESIAN_POINT('Ctrl Pts',(19.5451864564148,0.950924687748161,120.22263744994));
#55244=CARTESIAN_POINT('Ctrl Pts',(19.0680246080906,1.29995703510414,120.258505080578));
#55245=CARTESIAN_POINT('Ctrl Pts',(18.4876484020761,1.42413625094397,120.294513545472));
#55246=CARTESIAN_POINT('Ctrl Pts',(17.9049235301147,1.29995128236404,120.330661433598));
#55247=CARTESIAN_POINT('Ctrl Pts',(17.4219109382343,0.94724316719828,120.36694723955));
#55248=CARTESIAN_POINT('Ctrl Pts',(17.1239748622548,0.42606089295562,120.40336936399));
#55249=CARTESIAN_POINT('Ctrl Pts',(17.0646832076731,-0.173564467661854,
120.43992611466));
#55250=CARTESIAN_POINT('Ctrl Pts',(17.2561734622077,-0.747185474824163,
120.476615708097));
#55251=CARTESIAN_POINT('Ctrl Pts',(17.6667181243669,-1.19415105882015,120.513436271009));
#55252=CARTESIAN_POINT('Ctrl Pts',(18.2259712361402,-1.43528718231683,120.55038584204));
#55253=CARTESIAN_POINT('Ctrl Pts',(18.8370311234314,-1.4269354433336,120.587462370911));
#55254=CARTESIAN_POINT('Ctrl Pts',(19.3932495447825,-1.16885830485679,120.62466372221));
#55255=CARTESIAN_POINT('Ctrl Pts',(19.7968685982965,-0.70457726902139,120.661987673534));
#55256=CARTESIAN_POINT('Ctrl Pts',(19.9762240695575,-0.11403519053951,120.699431923752));
#55257=CARTESIAN_POINT('Ctrl Pts',(19.8984843651625,0.500186680137618,120.736994083826));
#55258=CARTESIAN_POINT('Ctrl Pts',(19.575656077446,1.03070741260493,120.774671696405));
#55259=CARTESIAN_POINT('Ctrl Pts',(19.0627604327755,1.38415482585726,120.812462202125));
#55260=CARTESIAN_POINT('Ctrl Pts',(18.4484458920318,1.49760672327847,120.850363008698));
#55261=CARTESIAN_POINT('Ctrl Pts',(17.8396489580402,1.34983590931418,120.888371367717));
#55262=CARTESIAN_POINT('Ctrl Pts',(17.3429428706895,0.96521497337526,120.926484611833));
#55263=CARTESIAN_POINT('Ctrl Pts',(17.045865677827,0.409809093734156,120.964699713595));
#55264=CARTESIAN_POINT('Ctrl Pts',(17.0014431624987,-0.220184717467978,
121.003014125745));
#55265=CARTESIAN_POINT('Ctrl Pts',(17.164424612689,-0.666099995461193,121.031821615483));
#55266=CARTESIAN_POINT('Ctrl Pts',(17.3434257995041,-0.919871476980275,
121.05105622202));
#55267=CARTESIAN_POINT('Ctrl Pts',(17.4797859795515,-1.07572928897003,121.063886410082));
#55268=CARTESIAN_POINT('Ctrl Pts',(17.7596234065678,-1.30908834442737,121.086360066906));
#55269=CARTESIAN_POINT('Ctrl Pts',(18.2520106540773,-1.50524820617466,121.118521093473));
#55270=CARTESIAN_POINT('Ctrl Pts',(18.8890624165871,-1.47853930079608,121.157201286479));
#55271=CARTESIAN_POINT('Ctrl Pts',(19.4608024223474,-1.19342203771302,121.19596496386));
#55272=CARTESIAN_POINT('Ctrl Pts',(19.8670946705987,-0.698578328455279,
121.234808961374));
#55273=CARTESIAN_POINT('Ctrl Pts',(20.0361439976898,-0.0797433644516521,
121.273729883387));
#55274=CARTESIAN_POINT('Ctrl Pts',(19.9375081708051,0.555375415482859,121.312724375624));
#55275=CARTESIAN_POINT('Ctrl Pts',(19.5874251537738,1.09577408462559,121.351788983929));
#55276=CARTESIAN_POINT('Ctrl Pts',(19.0462304801139,1.44664725684484,121.390920231817));
#55277=CARTESIAN_POINT('Ctrl Pts',(18.4078945414795,1.54602243253516,121.430114584083));
#55278=CARTESIAN_POINT('Ctrl Pts',(17.7836988323502,1.37574232630369,121.46936846982));
#55279=CARTESIAN_POINT('Ctrl Pts',(17.282784413028,0.964774261392473,121.508678276351));
#55280=CARTESIAN_POINT('Ctrl Pts',(16.9930369427572,0.384280279752719,121.548040351931));
#55281=CARTESIAN_POINT('Ctrl Pts',(16.965632387849,-0.264730861667821,121.587451011704));
#55282=CARTESIAN_POINT('Ctrl Pts',(17.2059822704094,-0.869015615574065,
121.62690653034));
#55283=CARTESIAN_POINT('Ctrl Pts',(17.6726767135541,-1.32289404488312,121.666403167446));
#55284=CARTESIAN_POINT('Ctrl Pts',(18.2846316707479,-1.54677468466741,121.705937127496));
#55285=CARTESIAN_POINT('Ctrl Pts',(18.9352078852143,-1.50113156051487,121.745504642789));
#55286=CARTESIAN_POINT('Ctrl Pts',(19.5108283377225,-1.19351370721864,121.785101820707));
#55287=CARTESIAN_POINT('Ctrl Pts',(19.9108571524216,-0.677265469818324,
121.824724937988));
#55288=CARTESIAN_POINT('Ctrl Pts',(20.0652157840296,-0.0423184316138819,
121.864369898394));
#55289=CARTESIAN_POINT('Ctrl Pts',(19.9467037274954,0.600613015659342,121.904033165255));
#55290=CARTESIAN_POINT('Ctrl Pts',(19.5757992709283,1.13923860750134,121.94371053936));
#55291=CARTESIAN_POINT('Ctrl Pts',(19.0170903691283,1.47948299020874,121.98339826705));
#55292=CARTESIAN_POINT('Ctrl Pts',(18.3680365032212,1.56185385513211,122.023092428396));
#55293=CARTESIAN_POINT('Ctrl Pts',(17.7419081841277,1.37192185757288,122.062789067507));
#55294=CARTESIAN_POINT('Ctrl Pts',(17.2479880852714,0.942825489960859,122.102484313511));
#55295=CARTESIAN_POINT('Ctrl Pts',(16.9724506261291,0.349491856500285,122.142174250389));
#55296=CARTESIAN_POINT('Ctrl Pts',(16.9632975544238,-0.304482856222713,
122.181854925629));
#55297=CARTESIAN_POINT('Ctrl Pts',(17.2219756104425,-0.90495722201614,122.221522510184));
#55298=CARTESIAN_POINT('Ctrl Pts',(17.703150736639,-1.34720967711664,122.261173032983));
#55299=CARTESIAN_POINT('Ctrl Pts',(18.32267005537,-1.55424124071767,122.300802661018));
#55300=CARTESIAN_POINT('Ctrl Pts',(18.9723111111196,-1.49021086379301,122.340407526305));
#55301=CARTESIAN_POINT('Ctrl Pts',(19.5387259317724,-1.16665041070326,122.379983728909));
#55302=CARTESIAN_POINT('Ctrl Pts',(19.9232635108214,-0.640390240190918,
122.41952751821));
#55303=CARTESIAN_POINT('Ctrl Pts',(20.0591820384592,-0.00354720571782957,
122.459034985586));
#55304=CARTESIAN_POINT('Ctrl Pts',(19.9232660830292,0.632615020340979,122.498502456349));
#55305=CARTESIAN_POINT('Ctrl Pts',(19.5397804872933,1.15720317221413,122.537926016389));
#55306=CARTESIAN_POINT('Ctrl Pts',(18.976169061755,1.47900616711341,122.57730217062));
#55307=CARTESIAN_POINT('Ctrl Pts',(18.3311000990434,1.54244114772495,122.616626980227));
#55308=CARTESIAN_POINT('Ctrl Pts',(17.7172503357923,1.33717049420449,122.65589694091));
#55309=CARTESIAN_POINT('Ctrl Pts',(17.2414907601859,0.899686660583994,122.695108360465));
#55310=CARTESIAN_POINT('Ctrl Pts',(16.9863250205813,0.307053962090209,122.734257662629));
#55311=CARTESIAN_POINT('Ctrl Pts',(16.9944497248883,-0.265604990902867,
122.768998723032));
#55312=CARTESIAN_POINT('Ctrl Pts',(17.1712479141773,-0.726942161622184,
122.799352272066));
#55313=CARTESIAN_POINT('Ctrl Pts',(17.5097094866836,-1.1784234221635,122.833999798576));
#55314=CARTESIAN_POINT('Ctrl Pts',(18.1440046231468,-1.52895577946613,122.877227151694));
#55315=CARTESIAN_POINT('Ctrl Pts',(19.0103596682388,-1.47993008996887,122.928960969768));
#55316=CARTESIAN_POINT('Ctrl Pts',(19.7156188499506,-0.979014184639401,
122.980547803872));
#55317=CARTESIAN_POINT('Ctrl Pts',(20.0453801510908,-0.182081354440587,
123.03198007533));
#55318=CARTESIAN_POINT('Ctrl Pts',(19.9009658784246,0.665665387675089,123.083250264192));
#55319=CARTESIAN_POINT('Ctrl Pts',(19.4248338794238,1.19762189380074,123.125834318843));
#55320=CARTESIAN_POINT('Ctrl Pts',(18.9192728107669,1.42256593967437,123.159813367155));
#55321=CARTESIAN_POINT('Ctrl Pts',(18.5245231164848,1.4787721179211,123.184310457398));
#55322=CARTESIAN_POINT('Ctrl Pts',(18.1454638254786,1.43075212555668,123.207825338745));
#55323=CARTESIAN_POINT('Ctrl Pts',(17.6907015228179,1.25302600903987,123.237875289869));
#55324=CARTESIAN_POINT('Ctrl Pts',(17.2340011183052,0.829040578783695,123.275344392595));
#55325=CARTESIAN_POINT('Ctrl Pts',(17.036580919693,0.240275284929825,123.3126849899));
#55326=CARTESIAN_POINT('Ctrl Pts',(17.0615849896374,-0.243150591543408,
123.342478462658));
#55327=CARTESIAN_POINT('Ctrl Pts',(17.2032609087076,-0.705038732123995,
123.372218231113));
#55328=CARTESIAN_POINT('Ctrl Pts',(17.5878551543339,-1.18711482918302,123.409291524378));
#55329=CARTESIAN_POINT('Ctrl Pts',(18.2106400712898,-1.44898576843933,123.44991921019));
#55330=CARTESIAN_POINT('Ctrl Pts',(18.8141776698684,-1.42578153316616,123.486729147975));
#55331=CARTESIAN_POINT('Ctrl Pts',(19.3107890371302,-1.20916212882085,123.519760499083));
#55332=CARTESIAN_POINT('Ctrl Pts',(19.6927353972249,-0.826888177330121,
123.552692753465));
#55333=CARTESIAN_POINT('Ctrl Pts',(19.9079783510014,-0.333205350440447,
123.58552446981));
#55334=CARTESIAN_POINT('Ctrl Pts',(19.927910114824,0.203440614612126,123.618254093443));
#55335=CARTESIAN_POINT('Ctrl Pts',(19.7509532260585,0.708563531543187,123.650880447743));
#55336=CARTESIAN_POINT('Ctrl Pts',(19.4608602251756,1.04556155423777,123.677981648566));
#55337=CARTESIAN_POINT('Ctrl Pts',(19.1676482101075,1.23701496091332,123.699609780472));
#55338=CARTESIAN_POINT('Ctrl Pts',(18.7910679570069,1.39369644218677,123.724801049022));
#55339=CARTESIAN_POINT('Ctrl Pts',(18.2247967647374,1.42170073442178,123.758885465202));
#55340=CARTESIAN_POINT('Ctrl Pts',(17.6899503199116,1.1635842287656,123.794602768893));
#55341=CARTESIAN_POINT('Ctrl Pts',(17.3755915425233,0.823902495683255,123.823078658873));
#55342=CARTESIAN_POINT('Ctrl Pts',(17.2102573337398,0.520040275543171,123.844386427488));
#55343=CARTESIAN_POINT('Ctrl Pts',(17.095967357383,0.0736009166210867,123.872730605635));
#55344=CARTESIAN_POINT('Ctrl Pts',(17.1620133383056,-0.450381505464488,
123.904505832421));
#55345=CARTESIAN_POINT('Ctrl Pts',(17.4696117223982,-0.938632889638676,
123.939664796233));
#55346=CARTESIAN_POINT('Ctrl Pts',(17.9029622950757,-1.25855076196019,123.972507589326));
#55347=CARTESIAN_POINT('Ctrl Pts',(18.4480459034613,-1.39083552515014,124.006531983721));
#55348=CARTESIAN_POINT('Ctrl Pts',(19.0183329635533,-1.28540085920782,124.041718831028));
#55349=CARTESIAN_POINT('Ctrl Pts',(19.4541943928961,-0.984922969711832,
124.073838648615));
#55350=CARTESIAN_POINT('Ctrl Pts',(19.6682715737307,-0.67104133868322,124.097112291097));
#55351=CARTESIAN_POINT('Ctrl Pts',(19.7868416138341,-0.382011184973219,
124.116465835797));
#55352=CARTESIAN_POINT('Ctrl Pts',(19.845095426036,-0.0889792271213038,
124.134815712575));
#55353=CARTESIAN_POINT('Ctrl Pts',(19.8133776059636,0.285969865030816,124.157928489657));
#55354=CARTESIAN_POINT('Ctrl Pts',(19.6795064045911,0.636485482650236,124.180974858546));
#55355=CARTESIAN_POINT('Ctrl Pts',(19.4544658023414,0.935380714529392,124.203954899115));
#55356=CARTESIAN_POINT('Ctrl Pts',(19.1563653681889,1.15962510660347,124.226868327498));
#55357=CARTESIAN_POINT('Ctrl Pts',(18.8377643876985,1.28119223747043,124.247811293649));
#55358=CARTESIAN_POINT('Ctrl Pts',(18.5321242045092,1.31762067856076,124.266801681851));
#55359=CARTESIAN_POINT('Ctrl Pts',(18.1649796321115,1.28429399639958,124.289540148812));
#55360=CARTESIAN_POINT('Ctrl Pts',(17.7362231944242,1.09949023306847,124.317869313244));
#55361=CARTESIAN_POINT('Ctrl Pts',(17.3588965090123,0.688544810591405,124.351714091216));
#55362=CARTESIAN_POINT('Ctrl Pts',(17.1830862730632,0.161768183835377,124.385408663042));
#55363=CARTESIAN_POINT('Ctrl Pts',(17.2375391699697,-0.388462801364577,
124.418953209553));
#55364=CARTESIAN_POINT('Ctrl Pts',(17.510749604725,-0.866293220470127,124.452347979479));
#55365=CARTESIAN_POINT('Ctrl Pts',(17.953313706052,-1.18941945391201,124.485593341375));
#55366=CARTESIAN_POINT('Ctrl Pts',(18.4868547743004,-1.30308143479277,124.51868975568));
#55367=CARTESIAN_POINT('Ctrl Pts',(19.0178962204122,-1.18942424606218,124.551637788857));
#55368=CARTESIAN_POINT('Ctrl Pts',(19.4542337078503,-0.8702144890527,124.584438104991));
#55369=CARTESIAN_POINT('Ctrl Pts',(19.7209361731848,-0.402730819941738,
124.617091470052));
#55370=CARTESIAN_POINT('Ctrl Pts',(19.7732021435748,0.130517736745286,124.649598749166));
#55371=CARTESIAN_POINT('Ctrl Pts',(19.6038673633271,0.636337480625157,124.681960907071));
#55372=CARTESIAN_POINT('Ctrl Pts',(19.244310467946,1.0271307853851,124.714179006478));
#55373=CARTESIAN_POINT('Ctrl Pts',(18.7586597506273,1.23605144177733,124.746254207572));
#55374=CARTESIAN_POINT('Ctrl Pts',(18.2323678346202,1.22842456764535,124.778187767811));
#55375=CARTESIAN_POINT('Ctrl Pts',(17.7571886611326,1.00747814552238,124.809981041022));
#55376=CARTESIAN_POINT('Ctrl Pts',(17.4151961591713,0.613446990910202,124.841635476325));
#55377=CARTESIAN_POINT('Ctrl Pts',(17.2646251988404,0.11626338066299,124.873152616656));
#55378=CARTESIAN_POINT('Ctrl Pts',(17.3299739672999,-0.396839428590113,
124.904534097586));
#55379=CARTESIAN_POINT('Ctrl Pts',(17.5980462947708,-0.836615880994796,
124.935781647363));
#55380=CARTESIAN_POINT('Ctrl Pts',(18.0205671134112,-1.12731152415149,124.966897085264));
#55381=CARTESIAN_POINT('Ctrl Pts',(18.5228589289931,-1.21969167859972,124.997882320446));
#55382=CARTESIAN_POINT('Ctrl Pts',(19.0170220921567,-1.09935899300576,125.028739349874));
#55383=CARTESIAN_POINT('Ctrl Pts',(19.4172956623671,-0.788959348815974,
125.059470256914));
#55384=CARTESIAN_POINT('Ctrl Pts',(19.6549180267179,-0.343945996706955,
125.090077211201));
#55385=CARTESIAN_POINT('Ctrl Pts',(19.6899160842551,0.157308971986261,125.120562466777));
#55386=CARTESIAN_POINT('Ctrl Pts',(19.5178066612108,0.627294647194249,125.150928360418));
#55387=CARTESIAN_POINT('Ctrl Pts',(19.1700918544773,0.984613592532787,125.181177309389));
#55388=CARTESIAN_POINT('Ctrl Pts',(18.7085131498763,1.16805288175899,125.211311809549));
#55389=CARTESIAN_POINT('Ctrl Pts',(18.2141093210495,1.14704615240416,125.241334435139));
#55390=CARTESIAN_POINT('Ctrl Pts',(17.7730146416868,0.926743182603541,125.271247836795));
#55391=CARTESIAN_POINT('Ctrl Pts',(17.4614821276217,0.546851681684302,125.301054739329));
#55392=CARTESIAN_POINT('Ctrl Pts',(17.3327303667907,0.0744996228417085,
125.330757939393));
#55393=CARTESIAN_POINT('Ctrl Pts',(17.4078770669085,-0.407601769713727,
125.360360303038));
#55394=CARTESIAN_POINT('Ctrl Pts',(17.6724992810162,-0.815611229448775,
125.389864765497));
#55395=CARTESIAN_POINT('Ctrl Pts',(18.0793755906884,-1.0791058017612,125.419274329063));
#55396=CARTESIAN_POINT('Ctrl Pts',(18.5568918796206,-1.15320571445106,125.448592060433));
#55397=CARTESIAN_POINT('Ctrl Pts',(19.0216174451001,-1.02619433748491,125.47782108828));
#55398=CARTESIAN_POINT('Ctrl Pts',(19.3928480017872,-0.721344483540626,
125.506964600284));
#55399=CARTESIAN_POINT('Ctrl Pts',(19.6065865223145,-0.29267161003856,125.536025842907));
#55400=CARTESIAN_POINT('Ctrl Pts',(19.6265455959889,0.184613405993531,125.565008119228));
#55401=CARTESIAN_POINT('Ctrl Pts',(19.4502857848642,0.627267625324512,125.593914785862));
#55402=CARTESIAN_POINT('Ctrl Pts',(19.1094565344714,0.958497326481144,125.622749250498));
#55403=CARTESIAN_POINT('Ctrl Pts',(18.6641306988289,1.12124490215563,125.65151496845));
#55404=CARTESIAN_POINT('Ctrl Pts',(18.1922438001048,1.08798886479353,125.680215442352));
#55405=CARTESIAN_POINT('Ctrl Pts',(17.7759904730407,0.865378727907893,125.70885422014));
#55406=CARTESIAN_POINT('Ctrl Pts',(17.4875467958782,0.492928571561681,125.737434891433));
#55407=CARTESIAN_POINT('Ctrl Pts',(17.3765912962239,0.0360231116649436,
125.765961085237));
#55408=CARTESIAN_POINT('Ctrl Pts',(17.4617752953106,-0.425529155060106,
125.794436465925));
#55409=CARTESIAN_POINT('Ctrl Pts',(17.7276023914822,-0.811397469264803,
125.822864733026));
#55410=CARTESIAN_POINT('Ctrl Pts',(18.1272364572306,-1.05466977543198,125.851249619116));
#55411=CARTESIAN_POINT('Ctrl Pts',(18.5907303019158,-1.11342078422065,125.879594886123));
#55412=CARTESIAN_POINT('Ctrl Pts',(19.0372330501214,-0.977914032009643,
125.9079043228));
#55413=CARTESIAN_POINT('Ctrl Pts',(19.3890522206571,-0.672205338262385,
125.93618174058));
#55414=CARTESIAN_POINT('Ctrl Pts',(19.5851322651224,-0.249885254342319,
125.964430973193));
#55415=CARTESIAN_POINT('Ctrl Pts',(19.5916177912335,0.215288095109658,125.992655874655));
#55416=CARTESIAN_POINT('Ctrl Pts',(19.4076799277922,0.642232516558101,126.02086031546));
#55417=CARTESIAN_POINT('Ctrl Pts',(19.0656071912909,0.956631975295786,126.049048179947));
#55418=CARTESIAN_POINT('Ctrl Pts',(18.6251546527486,1.1038329828714,126.07722336208));
#55419=CARTESIAN_POINT('Ctrl Pts',(18.1631369444732,1.05831622648696,126.105389764899));
#55420=CARTESIAN_POINT('Ctrl Pts',(17.7600722808915,0.828106591669271,126.133551298519));
#55421=CARTESIAN_POINT('Ctrl Pts',(17.4861931301989,0.453362374694559,126.161711876545));
#55422=CARTESIAN_POINT('Ctrl Pts',(17.3892461185869,-0.000608579703322207,
126.189875413034));
#55423=CARTESIAN_POINT('Ctrl Pts',(17.4861934126935,-0.45469525474382,126.218045818642));
#55424=CARTESIAN_POINT('Ctrl Pts',(17.7602536761873,-0.829727747487646,
126.246226999653));
#55425=CARTESIAN_POINT('Ctrl Pts',(18.1637977951782,-1.06023867129499,126.274422856165));
#55426=CARTESIAN_POINT('Ctrl Pts',(18.6266008887622,-1.10585668977637,126.302637278628));
#55427=CARTESIAN_POINT('Ctrl Pts',(19.0680252619495,-0.958355862859884,
126.33087414464));
#55428=CARTESIAN_POINT('Ctrl Pts',(19.4110278768796,-0.643133784314882,
126.359137315337));
#55429=CARTESIAN_POINT('Ctrl Pts',(19.5955669183692,-0.214853191351468,
126.387430634005));
#55430=CARTESIAN_POINT('Ctrl Pts',(19.5890811732739,0.252008008583668,126.415757924456));
#55431=CARTESIAN_POINT('Ctrl Pts',(19.3922180527628,0.676069561741979,126.444122988192));
#55432=CARTESIAN_POINT('Ctrl Pts',(19.038806518154,0.983192293191261,126.47252960012));
#55433=CARTESIAN_POINT('Ctrl Pts',(18.5900631360178,1.11940281866746,126.50098150721));
#55434=CARTESIAN_POINT('Ctrl Pts',(18.1240214367007,1.06035134340115,126.529482422973));
#55435=CARTESIAN_POINT('Ctrl Pts',(17.7219999728875,0.815652189115242,126.558036033249));
#55436=CARTESIAN_POINT('Ctrl Pts',(17.4544565122385,0.42732974030796,126.586645980413));
#55437=CARTESIAN_POINT('Ctrl Pts',(17.3686682099376,-0.0373706799791392,
126.615315883455));
#55438=CARTESIAN_POINT('Ctrl Pts',(17.4804111341263,-0.497601968494626,
126.644049291652));
#55439=CARTESIAN_POINT('Ctrl Pts',(17.7710524624981,-0.872926042665041,
126.672849763267));
#55440=CARTESIAN_POINT('Ctrl Pts',(18.1906784128292,-1.09736508436974,126.701720713779));
#55441=CARTESIAN_POINT('Ctrl Pts',(18.6665693810468,-1.13091363907518,126.73066569576));
#55442=CARTESIAN_POINT('Ctrl Pts',(19.115900304304,-0.966754134360276,126.759687863605));
#55443=CARTESIAN_POINT('Ctrl Pts',(19.4025342696002,-0.688135191455954,
126.783940470337));
#55444=CARTESIAN_POINT('Ctrl Pts',(19.548921654941,-0.40898722136763,126.803384174727));
#55445=CARTESIAN_POINT('Ctrl Pts',(19.634493180543,-0.10514408540288,126.822856841586));
#55446=CARTESIAN_POINT('Ctrl Pts',(19.6177649185308,0.296581417751861,126.847251669214));
#55447=CARTESIAN_POINT('Ctrl Pts',(19.4017808130667,0.729742583298161,126.876616113372));
#55448=CARTESIAN_POINT('Ctrl Pts',(19.0265757427209,1.03788810065477,126.906073797672));
#55449=CARTESIAN_POINT('Ctrl Pts',(18.5566758014723,1.16633154684977,126.935628014866));
#55450=CARTESIAN_POINT('Ctrl Pts',(18.0736913341831,1.09139777528755,126.965281594702));
#55451=CARTESIAN_POINT('Ctrl Pts',(17.6620120612613,0.824814395466043,126.995037511174));
#55452=CARTESIAN_POINT('Ctrl Pts',(17.3941799549046,0.411881837949739,127.024898556795));
#55453=CARTESIAN_POINT('Ctrl Pts',(17.3180870575981,-0.076187288283962,
127.05486751266));
#55454=CARTESIAN_POINT('Ctrl Pts',(17.4484565420247,-0.554528037140921,
127.084947054201));
#55455=CARTESIAN_POINT('Ctrl Pts',(17.764010774281,-0.939345893009087,127.115139797876));
#55456=CARTESIAN_POINT('Ctrl Pts',(18.2109253092811,-1.16257046672283,127.145448275684));
#55457=CARTESIAN_POINT('Ctrl Pts',(18.7119822511381,-1.18387264939932,127.175874945546));
#55458=CARTESIAN_POINT('Ctrl Pts',(19.1798875199966,-0.997932182564281,
127.206422183755));
#55459=CARTESIAN_POINT('Ctrl Pts',(19.5324518600497,-0.635646414421749,
127.237092283841));
#55460=CARTESIAN_POINT('Ctrl Pts',(19.7070045821325,-0.15902031214536,127.267887456223));
#55461=CARTESIAN_POINT('Ctrl Pts',(19.6715152795569,0.349422683108497,127.298809830743));
#55462=CARTESIAN_POINT('Ctrl Pts',(19.4304489650515,0.800905801272552,127.329861432512));
#55463=CARTESIAN_POINT('Ctrl Pts',(19.0242953873212,1.11587711326151,127.361044250206));
#55464=CARTESIAN_POINT('Ctrl Pts',(18.5227859928513,1.23800718975454,127.392360076625));
#55465=CARTESIAN_POINT('Ctrl Pts',(18.0129472939614,1.14424745798179,127.423810814418));
#55466=CARTESIAN_POINT('Ctrl Pts',(17.5840172876535,0.849149894711047,127.455397873974));
#55467=CARTESIAN_POINT('Ctrl Pts',(17.3118406201315,0.402652849536599,127.487123453883));
#55468=CARTESIAN_POINT('Ctrl Pts',(17.2454720166539,-0.118349922486156,
127.518987753904));
#55469=CARTESIAN_POINT('Ctrl Pts',(17.3984032330202,-0.623252153014087,
127.550994556485));
#55470=CARTESIAN_POINT('Ctrl Pts',(17.7456488662068,-1.02342067777811,127.58314143777));
#55471=CARTESIAN_POINT('Ctrl Pts',(18.2284245791308,-1.2478499399624,127.615434837012));
#55472=CARTESIAN_POINT('Ctrl Pts',(18.7627797364581,-1.25558862553399,127.647868301601));
#55473=CARTESIAN_POINT('Ctrl Pts',(19.2563109695001,-1.04333545914346,127.680455449859));
#55474=CARTESIAN_POINT('Ctrl Pts',(19.6216681619718,-0.646528379290638,
127.713175673656));
#55475=CARTESIAN_POINT('Ctrl Pts',(19.7927328538191,-0.132281528567945,
127.746058739306));
#55476=CARTESIAN_POINT('Ctrl Pts',(19.7503141195651,0.318711829041913,127.773584129304));
#55477=CARTESIAN_POINT('Ctrl Pts',(19.6053572776214,0.646435247116302,127.795653000386));
#55478=CARTESIAN_POINT('Ctrl Pts',(19.4462354220477,0.865492620926237,127.812264237419));
#55479=CARTESIAN_POINT('Ctrl Pts',(19.2457948002735,1.04692682939879,127.828924915749));
#55480=CARTESIAN_POINT('Ctrl Pts',(19.0155264002248,1.18188573320303,127.845613783594));
#55481=CARTESIAN_POINT('Ctrl Pts',(18.7628986552341,1.26490607478793,127.862310718442));
#55482=CARTESIAN_POINT('Ctrl Pts',(18.5810921207593,1.28450653733517,127.873458175477));
#55483=CARTESIAN_POINT('Ctrl Pts',(18.4867961500699,1.28530018715607,127.879040201486));
#55484=CARTESIAN_POINT('Ctrl Pts',(18.4876785229654,1.35973827479612,112.700349483895));
#55485=CARTESIAN_POINT('Ctrl Pts',(18.338278791091,1.35848083962102,112.709193479852));
#55486=CARTESIAN_POINT('Ctrl Pts',(18.1480053653849,1.32809629852819,112.721061171528));
#55487=CARTESIAN_POINT('Ctrl Pts',(17.8839969407007,1.22542744763376,112.73889627186));
#55488=CARTESIAN_POINT('Ctrl Pts',(17.6791187447654,1.10539854696858,112.753746837641));
#55489=CARTESIAN_POINT('Ctrl Pts',(17.4646853083375,0.911300230451853,112.771570316604));
#55490=CARTESIAN_POINT('Ctrl Pts',(17.2932741920643,0.675669450544188,112.789446398643));
#55491=CARTESIAN_POINT('Ctrl Pts',(17.1360309787953,0.320121093800881,112.813390160947));
#55492=CARTESIAN_POINT('Ctrl Pts',(17.0894953340232,-0.170507827027364,
112.843336784654));
#55493=CARTESIAN_POINT('Ctrl Pts',(17.2766257739384,-0.734670630418044,
112.879400942648));
#55494=CARTESIAN_POINT('Ctrl Pts',(17.6806702631371,-1.17437363669764,112.915626922413));
#55495=CARTESIAN_POINT('Ctrl Pts',(18.2307083272979,-1.41134855642679,112.951951982645));
#55496=CARTESIAN_POINT('Ctrl Pts',(18.8314790313439,-1.40324601833503,112.988419852557));
#55497=CARTESIAN_POINT('Ctrl Pts',(19.3786171248065,-1.14937703929912,113.025002743964));
#55498=CARTESIAN_POINT('Ctrl Pts',(19.7755321622389,-0.69277837996112,113.06171356028));
#55499=CARTESIAN_POINT('Ctrl Pts',(19.9519587360096,-0.111935044059312,
113.098541071133));
#55500=CARTESIAN_POINT('Ctrl Pts',(19.8754964114079,0.492238686716583,113.135489585637));
#55501=CARTESIAN_POINT('Ctrl Pts',(19.5579256638734,1.01412235273271,113.172553147416));
#55502=CARTESIAN_POINT('Ctrl Pts',(19.0533449396798,1.36184827886875,113.209731746827));
#55503=CARTESIAN_POINT('Ctrl Pts',(18.4489214934587,1.47348302587511,113.247022170108));
#55504=CARTESIAN_POINT('Ctrl Pts',(17.8498617671385,1.328077180479,113.284422590151));
#55505=CARTESIAN_POINT('Ctrl Pts',(17.3610409118715,0.949582216371434,113.32193043636));
#55506=CARTESIAN_POINT('Ctrl Pts',(17.0686356732366,0.402912605142576,113.359543389231));
#55507=CARTESIAN_POINT('Ctrl Pts',(17.0249018837744,-0.217196012200376,
113.397258901394));
#55508=CARTESIAN_POINT('Ctrl Pts',(17.2388349234317,-0.802630231903418,
113.435074404672));
#55509=CARTESIAN_POINT('Ctrl Pts',(17.6743443357727,-1.25077220769488,113.47298729979));
#55510=CARTESIAN_POINT('Ctrl Pts',(18.2563708833245,-1.48251999814763,113.510994797665));
#55511=CARTESIAN_POINT('Ctrl Pts',(18.883788180464,-1.45626180229461,113.54909429881));
#55512=CARTESIAN_POINT('Ctrl Pts',(19.4470878187195,-1.17536327214856,113.587282715003));
#55513=CARTESIAN_POINT('Ctrl Pts',(19.8474132957324,-0.687788270612358,
113.625557419335));
#55514=CARTESIAN_POINT('Ctrl Pts',(20.0140399050535,-0.0779171052049972,
113.663915285566));
#55515=CARTESIAN_POINT('Ctrl Pts',(19.9168245873902,0.548151296346475,113.702353379261));
#55516=CARTESIAN_POINT('Ctrl Pts',(19.5716780905909,1.08094531644977,113.740868668601));
#55517=CARTESIAN_POINT('Ctrl Pts',(19.0379862034942,1.42700170662234,113.779457936887));
#55518=CARTESIAN_POINT('Ctrl Pts',(18.5132840325881,1.5086380779085,113.811674845049));
#55519=CARTESIAN_POINT('Ctrl Pts',(18.1004282686362,1.44105976086287,113.837482080291));
#55520=CARTESIAN_POINT('Ctrl Pts',(17.7101473882012,1.28940494040579,113.863311335357));
#55521=CARTESIAN_POINT('Ctrl Pts',(17.2981783514831,0.951509020667204,113.895638332265));
#55522=CARTESIAN_POINT('Ctrl Pts',(17.0121782076903,0.378491346568276,113.934491682164));
#55523=CARTESIAN_POINT('Ctrl Pts',(16.9850947717721,-0.262273826574141,
113.973402866311));
#55524=CARTESIAN_POINT('Ctrl Pts',(17.2224477564689,-0.859069243423921,
114.012368441823));
#55525=CARTESIAN_POINT('Ctrl Pts',(17.6834527470367,-1.30743766470174,114.051384974311));
#55526=CARTESIAN_POINT('Ctrl Pts',(18.2881276456927,-1.52867649004814,114.090449046825));
#55527=CARTESIAN_POINT('Ctrl Pts',(18.9311491263506,-1.48358202333768,114.129557166494));
#55528=CARTESIAN_POINT('Ctrl Pts',(19.5002573154791,-1.17946619024642,114.168705781698));
#55529=CARTESIAN_POINT('Ctrl Pts',(19.895883518136,-0.668933671693989,114.207891428952));
#55530=CARTESIAN_POINT('Ctrl Pts',(20.0486043834432,-0.0408103026870864,
114.247110440653));
#55531=CARTESIAN_POINT('Ctrl Pts',(19.9313560547634,0.595409226935658,114.286359317187));
#55532=CARTESIAN_POINT('Ctrl Pts',(19.5642318343119,1.12858247956978,114.325634401683));
#55533=CARTESIAN_POINT('Ctrl Pts',(19.0110221780777,1.46550417236436,114.364932073146));
#55534=CARTESIAN_POINT('Ctrl Pts',(18.3681434811919,1.54711317103822,114.404248695611));
#55535=CARTESIAN_POINT('Ctrl Pts',(17.7477597391124,1.35894684363908,114.443580607611));
#55536=CARTESIAN_POINT('Ctrl Pts',(17.2581993100081,0.93367008885888,114.482924143866));
#55537=CARTESIAN_POINT('Ctrl Pts',(16.9849907759577,0.345400833559539,114.522275637151));
#55538=CARTESIAN_POINT('Ctrl Pts',(16.9758869025945,-0.303213715649527,
114.561631392287));
#55539=CARTESIAN_POINT('Ctrl Pts',(17.2325184431462,-0.899000003070434,
114.600987756475));
#55540=CARTESIAN_POINT('Ctrl Pts',(17.7100628186082,-1.3379326372978,114.640340988896));
#55541=CARTESIAN_POINT('Ctrl Pts',(18.3251652493023,-1.54355290685385,114.679687519473));
#55542=CARTESIAN_POINT('Ctrl Pts',(18.8628342525488,-1.49050064839209,114.712467468208));
#55543=CARTESIAN_POINT('Ctrl Pts',(19.2518081213493,-1.319262658196,114.738684473466));
#55544=CARTESIAN_POINT('Ctrl Pts',(19.5968527931672,-1.07127762690712,114.764896190921));
#55545=CARTESIAN_POINT('Ctrl Pts',(19.9154275427713,-0.63545754250494,114.797649532843));
#55546=CARTESIAN_POINT('Ctrl Pts',(20.0505695810008,-0.00220756764337195,
114.836932305889));
#55547=CARTESIAN_POINT('Ctrl Pts',(19.9154136835604,0.630564901895597,114.876189922281));
#55548=CARTESIAN_POINT('Ctrl Pts',(19.5338400364215,1.15258304952519,114.91541892072));
#55549=CARTESIAN_POINT('Ctrl Pts',(18.9727998510443,1.47293614770067,114.954615610741));
#55550=CARTESIAN_POINT('Ctrl Pts',(18.3304348019443,1.53614587402187,114.99377648997));
#55551=CARTESIAN_POINT('Ctrl Pts',(17.7188795785189,1.33165301578999,115.032897926425));
#55552=CARTESIAN_POINT('Ctrl Pts',(17.2447460413749,0.895715527281768,115.071976520637));
#55553=CARTESIAN_POINT('Ctrl Pts',(16.9902588839041,0.304783064849235,115.111008561568));
#55554=CARTESIAN_POINT('Ctrl Pts',(16.998448612415,-0.266235065591532,115.145659623941));
#55555=CARTESIAN_POINT('Ctrl Pts',(17.1746492311271,-0.726807957150069,
115.175944304194));
#55556=CARTESIAN_POINT('Ctrl Pts',(17.3649071445344,-0.979853975065223,
115.195395177983));
#55557=CARTESIAN_POINT('Ctrl Pts',(17.5179391530716,-1.12232983850705,115.208353638872));
#55558=CARTESIAN_POINT('Ctrl Pts',(17.5991280987468,-1.18808194474613,115.214831558541));
#55559=CARTESIAN_POINT('Ctrl Pts',(17.6847833163635,-1.2479102131603,115.221307669249));
#55560=CARTESIAN_POINT('Ctrl Pts',(17.8639071380312,-1.35535581298678,115.234257210543));
#55561=CARTESIAN_POINT('Ctrl Pts',(18.1591868534977,-1.4680197646283,115.253667690937));
#55562=CARTESIAN_POINT('Ctrl Pts',(18.5785806683425,-1.50338131849235,115.27952203358));
#55563=CARTESIAN_POINT('Ctrl Pts',(18.9910229601307,-1.42130509597836,115.305346731328));
#55564=CARTESIAN_POINT('Ctrl Pts',(19.3639961781648,-1.22854103830715,115.331142672617));
#55565=CARTESIAN_POINT('Ctrl Pts',(19.6690154415896,-0.940296747232436,
115.356907307457));
#55566=CARTESIAN_POINT('Ctrl Pts',(19.8814233359884,-0.579498862185678,
115.382641004355));
#55567=CARTESIAN_POINT('Ctrl Pts',(20.0218052305324,-0.039065010395108,
115.416908850278));
#55568=CARTESIAN_POINT('Ctrl Pts',(19.9257175915022,0.525726425592309,115.45110998076));
#55569=CARTESIAN_POINT('Ctrl Pts',(19.6543672323539,0.929749490353506,115.480974606343));
#55570=CARTESIAN_POINT('Ctrl Pts',(19.4572181758747,1.12181982433915,115.498021674344));
#55571=CARTESIAN_POINT('Ctrl Pts',(19.2347288283088,1.28428049014307,115.515056878813));
#55572=CARTESIAN_POINT('Ctrl Pts',(19.013651074864,1.3833118822926,115.529946665983));
#55573=CARTESIAN_POINT('Ctrl Pts',(18.8140247733603,1.43321755407129,115.542697012047));
#55574=CARTESIAN_POINT('Ctrl Pts',(18.7128363519114,1.45115700732122,115.54906996985));
#55575=CARTESIAN_POINT('Ctrl Pts',(18.6276598573334,1.46017834311691,115.554378697797));
#55576=CARTESIAN_POINT('Ctrl Pts',(18.5592862695786,1.46371178414657,115.558624633332));
#55577=CARTESIAN_POINT('Ctrl Pts',(18.281804518493,1.46901920455917,115.575840541739));
#55578=CARTESIAN_POINT('Ctrl Pts',(17.7789208622668,1.34044114145594,115.607043467896));
#55579=CARTESIAN_POINT('Ctrl Pts',(17.3515825252313,0.943867467580674,115.642111302339));
#55580=CARTESIAN_POINT('Ctrl Pts',(17.161718430748,0.586643344943619,115.667111195049));
#55581=CARTESIAN_POINT('Ctrl Pts',(17.0971415218615,0.395305592897811,115.679598666197));
#55582=CARTESIAN_POINT('Ctrl Pts',(17.0654186859172,0.237367172497665,115.689581011609));
#55583=CARTESIAN_POINT('Ctrl Pts',(17.0275491270296,-0.0824119897447905,
115.709536206168));
#55584=CARTESIAN_POINT('Ctrl Pts',(17.1213154380764,-0.612393720202946,
115.741905478085));
#55585=CARTESIAN_POINT('Ctrl Pts',(17.5848400159856,-1.19334019842358,115.786583882468));
#55586=CARTESIAN_POINT('Ctrl Pts',(18.2105492300219,-1.45653032695076,115.827406065294));
#55587=CARTESIAN_POINT('Ctrl Pts',(18.8172754847527,-1.43320988743828,115.864408413174));
#55588=CARTESIAN_POINT('Ctrl Pts',(19.3166435273073,-1.21540635448681,115.897624944836));
#55589=CARTESIAN_POINT('Ctrl Pts',(19.7009419977361,-0.830844298663376,
115.930754148081));
#55590=CARTESIAN_POINT('Ctrl Pts',(19.8813782039901,-0.416853424760839,
115.958288014972));
#55591=CARTESIAN_POINT('Ctrl Pts',(19.9276431736338,-0.0638821576866821,
115.980269583929));
#55592=CARTESIAN_POINT('Ctrl Pts',(19.9127472486195,0.20223062639115,115.996733473868));
#55593=CARTESIAN_POINT('Ctrl Pts',(19.8593136020091,0.41757635134816,116.010433712158));
#55594=CARTESIAN_POINT('Ctrl Pts',(19.7931822001391,0.581413531785223,116.021382537624));
#55595=CARTESIAN_POINT('Ctrl Pts',(19.6717448900476,0.81682145173997,116.037794354297));
#55596=CARTESIAN_POINT('Ctrl Pts',(19.4086990851244,1.12231198394179,116.06236784433));
#55597=CARTESIAN_POINT('Ctrl Pts',(18.9347537982859,1.37264233511827,116.095038203222));
#55598=CARTESIAN_POINT('Ctrl Pts',(18.4036743708657,1.43232551015976,116.12761233323));
#55599=CARTESIAN_POINT('Ctrl Pts',(18.017732623987,1.32879363369123,116.15196992527));
#55600=CARTESIAN_POINT('Ctrl Pts',(17.7876887319677,1.20427083424148,116.168177533439));
#55601=CARTESIAN_POINT('Ctrl Pts',(17.6428048499461,1.1074956958902,116.178974506447));
#55602=CARTESIAN_POINT('Ctrl Pts',(17.4148844793436,0.903876845597534,116.197846985979));
#55603=CARTESIAN_POINT('Ctrl Pts',(17.2622074736554,0.661128460586399,116.215331339299));
#55604=CARTESIAN_POINT('Ctrl Pts',(17.188027229338,0.457688297602254,116.228757052948));
#55605=CARTESIAN_POINT('Ctrl Pts',(17.168559043819,0.395766595906644,116.23278314266));
#55606=CARTESIAN_POINT('Ctrl Pts',(17.1520743242299,0.332985467597782,116.236807679468));
#55607=CARTESIAN_POINT('Ctrl Pts',(17.138527639409,0.26955084397591,116.240830617286));
#55608=CARTESIAN_POINT('Ctrl Pts',(17.1279448550524,0.205565981972609,116.244851992867));
#55609=CARTESIAN_POINT('Ctrl Pts',(17.1179125927233,0.119727148367452,116.250211712015));
#55610=CARTESIAN_POINT('Ctrl Pts',(17.10663249924,-0.117752725314212,116.264942373433));
#55611=CARTESIAN_POINT('Ctrl Pts',(17.1801410722104,-0.505505163832453,
116.288998851246));
#55612=CARTESIAN_POINT('Ctrl Pts',(17.4593468605389,-0.949572639259783,
116.320971494261));
#55613=CARTESIAN_POINT('Ctrl Pts',(17.8801051002652,-1.2599094895317,116.352839941182));
#55614=CARTESIAN_POINT('Ctrl Pts',(18.3835262236398,-1.39462467271549,116.384603580865));
#55615=CARTESIAN_POINT('Ctrl Pts',(18.8995848502807,-1.33631990116552,116.416261382716));
#55616=CARTESIAN_POINT('Ctrl Pts',(19.3572158707464,-1.09429062186641,116.447812674778));
#55617=CARTESIAN_POINT('Ctrl Pts',(19.6187260169908,-0.790095912733049,
116.472268975216));
#55618=CARTESIAN_POINT('Ctrl Pts',(19.7439727930601,-0.537901365985853,
116.489697925247));
#55619=CARTESIAN_POINT('Ctrl Pts',(19.8181256978155,-0.325610218012137,
116.503624869793));
#55620=CARTESIAN_POINT('Ctrl Pts',(19.8776026319941,0.0653392500041546,
116.527955084156));
#55621=CARTESIAN_POINT('Ctrl Pts',(19.7492623583921,0.626762380276667,116.562591461326));
#55622=CARTESIAN_POINT('Ctrl Pts',(19.2935621397076,1.14241638930198,116.603960385172));
#55623=CARTESIAN_POINT('Ctrl Pts',(18.6500528451987,1.37621044955443,116.64513338571));
#55624=CARTESIAN_POINT('Ctrl Pts',(17.9761635526829,1.2742602408342,116.686109582385));
#55625=CARTESIAN_POINT('Ctrl Pts',(17.5146651224903,0.924134010931,116.720941344535));
#55626=CARTESIAN_POINT('Ctrl Pts',(17.2774362791059,0.520220428704234,116.749716614797));
#55627=CARTESIAN_POINT('Ctrl Pts',(17.1529354063379,0.0413427657848591,
116.780100883198));
#55628=CARTESIAN_POINT('Ctrl Pts',(17.2594728905108,-0.583805099635299,
116.817924242688));
#55629=CARTESIAN_POINT('Ctrl Pts',(17.7643920189576,-1.14787815539454,116.863060893889));
#55630=CARTESIAN_POINT('Ctrl Pts',(18.4878485549571,-1.355639848724,116.907946311528));
#55631=CARTESIAN_POINT('Ctrl Pts',(19.2068886828874,-1.1479083033055,116.952580891862));
#55632=CARTESIAN_POINT('Ctrl Pts',(19.7025859315818,-0.59243259627754,116.996965410243));
#55633=CARTESIAN_POINT('Ctrl Pts',(19.805116781009,0.0155843273252081,117.033744906381));
#55634=CARTESIAN_POINT('Ctrl Pts',(19.6849763257637,0.477310867630742,117.063044708738));
#55635=CARTESIAN_POINT('Ctrl Pts',(19.5041028285569,0.784752423535641,117.084957745122));
#55636=CARTESIAN_POINT('Ctrl Pts',(19.2452349298756,1.02876411530207,117.106809363928));
#55637=CARTESIAN_POINT('Ctrl Pts',(18.8252583549806,1.24665288186946,117.135863022342));
#55638=CARTESIAN_POINT('Ctrl Pts',(18.2198687746404,1.28039646177613,117.172027569721));
#55639=CARTESIAN_POINT('Ctrl Pts',(17.5866457772006,0.929702296368013,117.21518301736));
#55640=CARTESIAN_POINT('Ctrl Pts',(17.2390532742044,0.299598173471757,117.258099043471));
#55641=CARTESIAN_POINT('Ctrl Pts',(17.2797153311823,-0.415006662101263,
117.3007784115));
#55642=CARTESIAN_POINT('Ctrl Pts',(17.6920802994576,-0.995196786608285,
117.343224228662));
#55643=CARTESIAN_POINT('Ctrl Pts',(18.3463415258393,-1.26562861592044,117.385439850698));
#55644=CARTESIAN_POINT('Ctrl Pts',(19.0404591281284,-1.14715003431039,117.427428928389));
#55645=CARTESIAN_POINT('Ctrl Pts',(19.5623711434035,-0.680042513891968,
117.469195380227));
#55646=CARTESIAN_POINT('Ctrl Pts',(19.7547673292631,-0.0103754829418355,
117.510743394758));
#55647=CARTESIAN_POINT('Ctrl Pts',(19.5623929190238,0.655560976653802,117.552077418062));
#55648=CARTESIAN_POINT('Ctrl Pts',(19.0478297506675,1.11474704186936,117.593202163305));
#55649=CARTESIAN_POINT('Ctrl Pts',(18.3712156490552,1.22922475979801,117.63412259366));
#55650=CARTESIAN_POINT('Ctrl Pts',(17.7404829013797,0.967463930769031,117.674843912414));
#55651=CARTESIAN_POINT('Ctrl Pts',(17.3475629596244,0.412913264252416,117.715371566815));
#55652=CARTESIAN_POINT('Ctrl Pts',(17.310064375504,-0.262540500826519,117.755711245779));
#55653=CARTESIAN_POINT('Ctrl Pts',(17.636197520999,-0.85173985968551,117.795868851832));
#55654=CARTESIAN_POINT('Ctrl Pts',(18.2232061575254,-1.17571779828974,117.83585051381));
#55655=CARTESIAN_POINT('Ctrl Pts',(18.8898049415706,-1.13787460741934,117.875662566524));
#55656=CARTESIAN_POINT('Ctrl Pts',(19.4318065563587,-0.752832224962471,
117.915311577176));
#55657=CARTESIAN_POINT('Ctrl Pts',(19.6850206338496,-0.140764865189098,
117.954804243761));
#55658=CARTESIAN_POINT('Ctrl Pts',(19.5924643948714,0.401139914316672,117.987590349654));
#55659=CARTESIAN_POINT('Ctrl Pts',(19.3550318497187,0.754660044567889,118.01374802109));
#55660=CARTESIAN_POINT('Ctrl Pts',(19.0307937520553,1.02963893852138,118.039859642854));
#55661=CARTESIAN_POINT('Ctrl Pts',(18.50622690624,1.18069309462962,118.072414545105));
#55662=CARTESIAN_POINT('Ctrl Pts',(17.8787720595626,0.999543022593704,118.111353082998));
#55663=CARTESIAN_POINT('Ctrl Pts',(17.4452307248378,0.514012685374898,118.15017156465));
#55664=CARTESIAN_POINT('Ctrl Pts',(17.3367378446691,-0.125987357398448,
118.188877898695));
#55665=CARTESIAN_POINT('Ctrl Pts',(17.5846953995656,-0.723951514978575,
118.227479865732));
#55666=CARTESIAN_POINT('Ctrl Pts',(18.1114543571691,-1.0974563568826,118.265985524989));
#55667=CARTESIAN_POINT('Ctrl Pts',(18.7547058180995,-1.13336389519741,118.304402965018));
#55668=CARTESIAN_POINT('Ctrl Pts',(19.3173182988927,-0.822244782737743,
118.342740449353));
#55669=CARTESIAN_POINT('Ctrl Pts',(19.6275738333935,-0.26047787608183,118.381006236972));
#55670=CARTESIAN_POINT('Ctrl Pts',(19.5915390368011,0.379069408536245,118.419208846237));
#55671=CARTESIAN_POINT('Ctrl Pts',(19.2211927231264,0.900906054925335,118.45735657839));
#55672=CARTESIAN_POINT('Ctrl Pts',(18.7293427115169,1.10434931242854,118.489108025697));
#55673=CARTESIAN_POINT('Ctrl Pts',(18.3161133166046,1.09194722489886,118.514490132623));
#55674=CARTESIAN_POINT('Ctrl Pts',(18.0209984782359,0.998187264691806,118.533518695961));
#55675=CARTESIAN_POINT('Ctrl Pts',(17.7634928966558,0.82595466122776,118.552539656177));
#55676=CARTESIAN_POINT('Ctrl Pts',(17.563775870497,0.589521138450256,118.571554845456));
#55677=CARTESIAN_POINT('Ctrl Pts',(17.437363222974,0.306953574752756,118.590564605243));
#55678=CARTESIAN_POINT('Ctrl Pts',(17.3941193006543,0.000610802263239836,
118.609570707512));
#55679=CARTESIAN_POINT('Ctrl Pts',(17.4373534640508,-0.305796483992987,
118.628573614322));
#55680=CARTESIAN_POINT('Ctrl Pts',(17.5426862832814,-0.541016627132415,
118.644408242671));
#55681=CARTESIAN_POINT('Ctrl Pts',(17.6634779226648,-0.706381682981929,
118.657075049229));
#55682=CARTESIAN_POINT('Ctrl Pts',(17.806243697093,-0.852950163395337,118.66974258048));
#55683=CARTESIAN_POINT('Ctrl Pts',(18.106057194281,-1.05418422554283,118.691910013046));
#55684=CARTESIAN_POINT('Ctrl Pts',(18.6293906886623,-1.14333393643523,118.72358214913));
#55685=CARTESIAN_POINT('Ctrl Pts',(19.2187652101556,-0.899240835761239,
118.761603122514));
#55686=CARTESIAN_POINT('Ctrl Pts',(19.5261380986293,-0.46579781924761,118.793306539549));
#55687=CARTESIAN_POINT('Ctrl Pts',(19.5960047419514,-0.110829187609168,
118.815513403398));
#55688=CARTESIAN_POINT('Ctrl Pts',(19.5932711946567,0.0941203340922264,
118.828206979085));
#55689=CARTESIAN_POINT('Ctrl Pts',(19.561775887923,0.297086240693117,118.840904501667));
#55690=CARTESIAN_POINT('Ctrl Pts',(19.4694460545618,0.538278919044113,118.856782163855));
#55691=CARTESIAN_POINT('Ctrl Pts',(19.2211350815969,0.869636695096682,118.882201823917));
#55692=CARTESIAN_POINT('Ctrl Pts',(18.7546109285557,1.12774604749691,118.914006897353));
#55693=CARTESIAN_POINT('Ctrl Pts',(18.1144942029186,1.09193664690372,118.952230982635));
#55694=CARTESIAN_POINT('Ctrl Pts',(17.5906842728557,0.720468306166889,118.990521107805));
#55695=CARTESIAN_POINT('Ctrl Pts',(17.3855246482535,0.225277058832011,119.022491989366));
#55696=CARTESIAN_POINT('Ctrl Pts',(17.3980555839542,-0.191783272636398,
119.048109713078));
#55697=CARTESIAN_POINT('Ctrl Pts',(17.4768927747722,-0.44037660910954,119.06413951312));
#55698=CARTESIAN_POINT('Ctrl Pts',(17.5671568068215,-0.597988874584677,
119.075369732831));
#55699=CARTESIAN_POINT('Ctrl Pts',(17.627583349682,-0.682021820729704,119.08179007171));
#55700=CARTESIAN_POINT('Ctrl Pts',(17.6939097716351,-0.761655148296046,
119.088212380741));
#55701=CARTESIAN_POINT('Ctrl Pts',(17.7869510861829,-0.852129061282766,
119.096244363201));
#55702=CARTESIAN_POINT('Ctrl Pts',(17.9547144167929,-0.974787629722701,
119.109102616347));
#55703=CARTESIAN_POINT('Ctrl Pts',(18.1937763612775,-1.0818094293345,119.125191738617));
#55704=CARTESIAN_POINT('Ctrl Pts',(18.5054383431021,-1.1258363795764,119.144523919164));
#55705=CARTESIAN_POINT('Ctrl Pts',(18.8175251592586,-1.08180363622223,119.163883306933));
#55706=CARTESIAN_POINT('Ctrl Pts',(19.1056462869439,-0.952921422339809,
119.183270109433));
#55707=CARTESIAN_POINT('Ctrl Pts',(19.3471812503215,-0.748996843631803,
119.202685994533));
#55708=CARTESIAN_POINT('Ctrl Pts',(19.5230935936411,-0.485797243267148,
119.222131101893));
#55709=CARTESIAN_POINT('Ctrl Pts',(19.6194235398893,-0.183681159155142,
119.241607538908));
#55710=CARTESIAN_POINT('Ctrl Pts',(19.6283568615701,0.133769359585175,119.261114722082));
#55711=CARTESIAN_POINT('Ctrl Pts',(19.5621898852985,0.39051406225891,119.277398730761));
#55712=CARTESIAN_POINT('Ctrl Pts',(19.467979719698,0.579067452723987,119.290441977098));
#55713=CARTESIAN_POINT('Ctrl Pts',(19.3185921773537,0.796417004314266,119.306760645479));
#55714=CARTESIAN_POINT('Ctrl Pts',(19.0271066040016,1.03580841985484,119.329646794098));
#55715=CARTESIAN_POINT('Ctrl Pts',(18.5579560526582,1.16400930978687,119.359152271126));
#55716=CARTESIAN_POINT('Ctrl Pts',(18.0760367110303,1.08921289338611,119.388741208946));
#55717=CARTESIAN_POINT('Ctrl Pts',(17.6654854616247,0.823330943755025,119.418416546625));
#55718=CARTESIAN_POINT('Ctrl Pts',(17.3985369873615,0.411710794457526,119.448181135551));
#55719=CARTESIAN_POINT('Ctrl Pts',(17.3227666115826,-0.0745209629554153,
119.478037892946));
#55720=CARTESIAN_POINT('Ctrl Pts',(17.4525835817918,-0.550846602669221,
119.507989394093));
#55721=CARTESIAN_POINT('Ctrl Pts',(17.7143528381942,-0.869942542802271,
119.533030493605));
#55722=CARTESIAN_POINT('Ctrl Pts',(17.9889445791141,-1.04484589484823,119.553113195196));
#55723=CARTESIAN_POINT('Ctrl Pts',(18.2942955374926,-1.15931837182444,119.573229991214));
#55724=CARTESIAN_POINT('Ctrl Pts',(18.7094283500856,-1.17700658256433,119.598440038838));
#55725=CARTESIAN_POINT('Ctrl Pts',(19.1744277236937,-0.992164148776086,
119.628797431618));
#55726=CARTESIAN_POINT('Ctrl Pts',(19.5246105085742,-0.632300664711906,
119.659262467001));
#55727=CARTESIAN_POINT('Ctrl Pts',(19.6978971318757,-0.159064142767438,
119.689837552661));
#55728=CARTESIAN_POINT('Ctrl Pts',(19.6626494698746,0.345510270040854,119.720524932272));
#55729=CARTESIAN_POINT('Ctrl Pts',(19.4235062092649,0.793350318368254,119.751326824166));
#55730=CARTESIAN_POINT('Ctrl Pts',(19.0207724226401,1.10563928405634,119.782245336604));
#55731=CARTESIAN_POINT('Ctrl Pts',(18.5237348992026,1.22664815333434,119.813282525917));
#55732=CARTESIAN_POINT('Ctrl Pts',(18.0186212112409,1.13376405338814,119.844440332931));
#55733=CARTESIAN_POINT('Ctrl Pts',(17.6647078195633,0.890180692604903,119.870507283873));
#55734=CARTESIAN_POINT('Ctrl Pts',(17.459152794792,0.620520297905578,119.891422999201));
#55735=CARTESIAN_POINT('Ctrl Pts',(17.3135738426375,0.313569874486673,119.912380371528));
#55736=CARTESIAN_POINT('Ctrl Pts',(17.2588234924652,-0.116038476650668,
119.938655950413));
#55737=CARTESIAN_POINT('Ctrl Pts',(17.4100983478659,-0.615449946450397,
119.970314243228));
#55738=CARTESIAN_POINT('Ctrl Pts',(17.7535352748928,-1.01112010205256,120.002101741838));
#55739=CARTESIAN_POINT('Ctrl Pts',(18.2305891354705,-1.23292472309362,120.034019862503));
#55740=CARTESIAN_POINT('Ctrl Pts',(18.7588013590758,-1.24056168734763,120.066069997976));
#55741=CARTESIAN_POINT('Ctrl Pts',(19.2460849895487,-1.03092328241255,120.098253406646));
#55742=CARTESIAN_POINT('Ctrl Pts',(19.6067436569891,-0.638908623644245,
120.130571281471));
#55743=CARTESIAN_POINT('Ctrl Pts',(19.7765414423687,-0.131657613778088,
120.16302471018));
#55744=CARTESIAN_POINT('Ctrl Pts',(19.7241268936388,0.402946109902079,120.195614696143));
#55745=CARTESIAN_POINT('Ctrl Pts',(19.4568058001641,0.871483019948602,120.228342146454));
#55746=CARTESIAN_POINT('Ctrl Pts',(19.0195888769497,1.19131601339264,120.261207876936));
#55747=CARTESIAN_POINT('Ctrl Pts',(18.4876303130866,1.30515498304331,120.29421260826));
#55748=CARTESIAN_POINT('Ctrl Pts',(17.9533196433611,1.19131025373105,120.327356967205));
#55749=CARTESIAN_POINT('Ctrl Pts',(17.5102434085246,0.867796104159015,120.360641485681));
#55750=CARTESIAN_POINT('Ctrl Pts',(17.2367984070158,0.389513905763427,120.394066601003));
#55751=CARTESIAN_POINT('Ctrl Pts',(17.1823257731603,-0.161052944534343,
120.427632654705));
#55752=CARTESIAN_POINT('Ctrl Pts',(17.3582173349526,-0.688057393908344,
120.461339892745));
#55753=CARTESIAN_POINT('Ctrl Pts',(17.7355965521711,-1.09897149996487,120.495188465041));
#55754=CARTESIAN_POINT('Ctrl Pts',(18.2500378061209,-1.32083060054573,120.529178426105));
#55755=CARTESIAN_POINT('Ctrl Pts',(18.8125577781375,-1.31318644286814,120.563309734203));
#55756=CARTESIAN_POINT('Ctrl Pts',(19.3250052395169,-1.07547039577926,120.597582252196));
#55757=CARTESIAN_POINT('Ctrl Pts',(19.697188512651,-0.647426242261582,120.631995745907));
#55758=CARTESIAN_POINT('Ctrl Pts',(19.8627512839161,-0.102480320396054,
120.666549887297));
#55759=CARTESIAN_POINT('Ctrl Pts',(19.7910024142767,0.464853743541633,120.70124425028));
#55760=CARTESIAN_POINT('Ctrl Pts',(19.4925884258856,0.955366343499383,120.73607831879));
#55761=CARTESIAN_POINT('Ctrl Pts',(19.017965346801,1.28251422077536,120.771051472002));
#55762=CARTESIAN_POINT('Ctrl Pts',(18.448872236062,1.38768021419735,120.806163012952));
#55763=CARTESIAN_POINT('Ctrl Pts',(17.8842561866098,1.25070220238676,120.841412116456));
#55764=CARTESIAN_POINT('Ctrl Pts',(17.4230517533873,0.893660617828872,120.876797928954));
#55765=CARTESIAN_POINT('Ctrl Pts',(17.1468515279311,0.377437762693973,120.912319382562));
#55766=CARTESIAN_POINT('Ctrl Pts',(17.1054347892236,-0.208842011271403,
120.947975548869));
#55767=CARTESIAN_POINT('Ctrl Pts',(17.257242942961,-0.624353404722209,120.974817587713));
#55768=CARTESIAN_POINT('Ctrl Pts',(17.4241596596904,-0.860998050927015,
120.992753814121));
#55769=CARTESIAN_POINT('Ctrl Pts',(17.5513580669707,-1.00638554422223,121.004722033497));
#55770=CARTESIAN_POINT('Ctrl Pts',(17.8125062676019,-1.22417547142694,121.025695549015));
#55771=CARTESIAN_POINT('Ctrl Pts',(18.2724517094306,-1.40748417284606,121.055739282651));
#55772=CARTESIAN_POINT('Ctrl Pts',(18.8683616599553,-1.38258592298105,121.091921232995));
#55773=CARTESIAN_POINT('Ctrl Pts',(19.4039469371452,-1.11559596226272,121.128230999328));
#55774=CARTESIAN_POINT('Ctrl Pts',(19.7851220860264,-0.651485254357956,
121.164667024263));
#55775=CARTESIAN_POINT('Ctrl Pts',(19.9440082322412,-0.0702040346042679,
121.201227575976));
#55776=CARTESIAN_POINT('Ctrl Pts',(19.8513116568888,0.527285905129969,121.237910885291));
#55777=CARTESIAN_POINT('Ctrl Pts',(19.5215667915217,1.03646753264763,121.274715074731));
#55778=CARTESIAN_POINT('Ctrl Pts',(19.0109647654682,1.3676240556558,121.31163819733));
#55779=CARTESIAN_POINT('Ctrl Pts',(18.4077307987017,1.46163653233743,121.348678218649));
#55780=CARTESIAN_POINT('Ctrl Pts',(17.8168866182968,1.30056114436624,121.385833028301));
#55781=CARTESIAN_POINT('Ctrl Pts',(17.3419316367841,0.911026491110346,121.42310043786));
#55782=CARTESIAN_POINT('Ctrl Pts',(17.0666957019877,0.359844238279606,121.460478181363));
#55783=CARTESIAN_POINT('Ctrl Pts',(17.0405213308045,-0.257462790858785,
121.49796392011));
#55784=CARTESIAN_POINT('Ctrl Pts',(17.2694126324673,-0.833236802289572,
121.535555236205));
#55785=CARTESIAN_POINT('Ctrl Pts',(17.7147338114203,-1.26648509350842,121.57324965169));
#55786=CARTESIAN_POINT('Ctrl Pts',(18.2997310041706,-1.48062436312049,121.611044598073));
#55787=CARTESIAN_POINT('Ctrl Pts',(18.9227806176326,-1.43702806539659,121.648937478815));
#55788=CARTESIAN_POINT('Ctrl Pts',(19.475064541157,-1.14201388349045,121.686925554159));
#55789=CARTESIAN_POINT('Ctrl Pts',(19.8596141628965,-0.645935586892937,
121.725006162078));
#55790=CARTESIAN_POINT('Ctrl Pts',(20.008346706193,-0.0346372378620192,
121.763176310523));
#55791=CARTESIAN_POINT('Ctrl Pts',(19.8941556704044,0.585521991047194,121.80143337875));
#55792=CARTESIAN_POINT('Ctrl Pts',(19.5358462733169,1.10607313572164,121.839774198206));
#55793=CARTESIAN_POINT('Ctrl Pts',(18.995024727083,1.43556935990143,121.878195884757));
#55794=CARTESIAN_POINT('Ctrl Pts',(18.3655210390793,1.51558521854799,121.916695382839));
#55795=CARTESIAN_POINT('Ctrl Pts',(17.7570606450874,1.33114453962665,121.95526955489));
#55796=CARTESIAN_POINT('Ctrl Pts',(17.2761160603867,0.913489361496773,121.993915283113));
#55797=CARTESIAN_POINT('Ctrl Pts',(17.0072368483796,0.334798105910418,122.032629365255));
#55798=CARTESIAN_POINT('Ctrl Pts',(16.9981624241316,-0.304316767733318,
122.071408517403));
#55799=CARTESIAN_POINT('Ctrl Pts',(17.251330532035,-0.892329965491541,122.11024951087));
#55800=CARTESIAN_POINT('Ctrl Pts',(17.7233021624858,-1.3263014609352,122.149148947241));
#55801=CARTESIAN_POINT('Ctrl Pts',(18.3322262968092,-1.5299313411392,122.188103494914));
#55802=CARTESIAN_POINT('Ctrl Pts',(18.9720612013498,-1.46700073882079,122.227109746095));
#55803=CARTESIAN_POINT('Ctrl Pts',(19.5310749635394,-1.14782155829681,122.266164210345));
#55804=CARTESIAN_POINT('Ctrl Pts',(19.9113979815986,-0.627556137759355,
122.305263484811));
#55805=CARTESIAN_POINT('Ctrl Pts',(20.0461854224048,0.00334322599405469,
122.344403969626));
#55806=CARTESIAN_POINT('Ctrl Pts',(19.9113972671777,0.63487192224289,122.383582231813));
#55807=CARTESIAN_POINT('Ctrl Pts',(19.5300757175112,1.15672922617075,122.422794562142));
#55808=CARTESIAN_POINT('Ctrl Pts',(18.9684369249769,1.47756196833367,122.462037597625));
#55809=CARTESIAN_POINT('Ctrl Pts',(18.3242818697673,1.54104364912502,122.501307500968));
#55810=CARTESIAN_POINT('Ctrl Pts',(17.7100244133753,1.33578019286523,122.540600797604));
#55811=CARTESIAN_POINT('Ctrl Pts',(17.2329398048057,0.897263318486983,122.579913783485));
#55812=CARTESIAN_POINT('Ctrl Pts',(16.9764784072532,0.301964176637347,122.619242811121));
#55813=CARTESIAN_POINT('Ctrl Pts',(16.9845337828457,-0.274473648200087,
122.654212995416));
#55814=CARTESIAN_POINT('Ctrl Pts',(17.1627555053455,-0.739648570522611,
122.684817494633));
#55815=CARTESIAN_POINT('Ctrl Pts',(17.5044140404774,-1.19548846578833,122.719797873699));
#55816=CARTESIAN_POINT('Ctrl Pts',(18.1459455530736,-1.55032796429415,122.763527455907));
#55817=CARTESIAN_POINT('Ctrl Pts',(19.0247080539113,-1.50093222138397,122.81600109576));
#55818=CARTESIAN_POINT('Ctrl Pts',(19.7421346852786,-0.991773946961065,
122.868463997585));
#55819=CARTESIAN_POINT('Ctrl Pts',(20.078678890067,-0.179297852006348,122.920907533627));
#55820=CARTESIAN_POINT('Ctrl Pts',(19.931361285469,0.687441108918969,122.97332295464));
#55821=CARTESIAN_POINT('Ctrl Pts',(19.4435177864377,1.2328776932785,123.016971870743));
#55822=CARTESIAN_POINT('Ctrl Pts',(18.9243150922261,1.46395147514551,123.051868326394));
#55823=CARTESIAN_POINT('Ctrl Pts',(18.5183951569639,1.52178329193078,123.077059337171));
#55824=CARTESIAN_POINT('Ctrl Pts',(18.1281145921538,1.47237094917012,123.101269725337));
#55825=CARTESIAN_POINT('Ctrl Pts',(17.6593637564239,1.28921713675561,123.132243778228));
#55826=CARTESIAN_POINT('Ctrl Pts',(17.1876918207849,0.851581019041659,123.170931091307));
#55827=CARTESIAN_POINT('Ctrl Pts',(16.9832215152354,0.242357233593553,123.209572770744));
#55828=CARTESIAN_POINT('Ctrl Pts',(17.0091058149915,-0.258767597083051,
123.240456182328));
#55829=CARTESIAN_POINT('Ctrl Pts',(17.1560922813407,-0.738084296272097,
123.271318228827));
#55830=CARTESIAN_POINT('Ctrl Pts',(17.5557244048119,-1.23929750545205,123.309854723166));
#55831=CARTESIAN_POINT('Ctrl Pts',(18.2044422297094,-1.51227958537405,123.352178753354));
#55832=CARTESIAN_POINT('Ctrl Pts',(18.8343869808506,-1.48815787538939,123.390598660515));
#55833=CARTESIAN_POINT('Ctrl Pts',(19.353588737119,-1.2617754559261,123.425130511472));
#55834=CARTESIAN_POINT('Ctrl Pts',(19.7535878185842,-0.861555544152392,
123.459613986599));
#55835=CARTESIAN_POINT('Ctrl Pts',(19.9794032819064,-0.343829749696201,
123.494046857608));
#55836=CARTESIAN_POINT('Ctrl Pts',(20.000423736225,0.219869657394578,123.528426618707));
#55837=CARTESIAN_POINT('Ctrl Pts',(19.8143309546131,0.751313711751814,123.562751365816));
#55838=CARTESIAN_POINT('Ctrl Pts',(19.5087207298247,1.10644312189301,123.591307129293));
#55839=CARTESIAN_POINT('Ctrl Pts',(19.1994192267151,1.30841669722232,123.614122206283));
#55840=CARTESIAN_POINT('Ctrl Pts',(18.8018880211566,1.47383184469139,123.640715972828));
#55841=CARTESIAN_POINT('Ctrl Pts',(18.203271795634,1.50358610427353,123.676747659749));
#55842=CARTESIAN_POINT('Ctrl Pts',(17.636687751151,1.23032070130387,123.714579983589));
#55843=CARTESIAN_POINT('Ctrl Pts',(17.30320303094,0.870020035335568,123.744785773105));
#55844=CARTESIAN_POINT('Ctrl Pts',(17.1276403635631,0.547396546141828,123.767409714068));
#55845=CARTESIAN_POINT('Ctrl Pts',(17.0061453562421,0.0729490378705759,
123.79753311268));
#55846=CARTESIAN_POINT('Ctrl Pts',(17.076311597054,-0.484727721015513,123.831350608742));
#55847=CARTESIAN_POINT('Ctrl Pts',(17.4041389802875,-1.00524236044422,123.868829379186));
#55848=CARTESIAN_POINT('Ctrl Pts',(17.8666645324534,-1.34678546980139,123.903886582043));
#55849=CARTESIAN_POINT('Ctrl Pts',(18.4492984685224,-1.48828068205571,123.940256330297));
#55850=CARTESIAN_POINT('Ctrl Pts',(19.0598066985192,-1.37550604828877,123.977923741201));
#55851=CARTESIAN_POINT('Ctrl Pts',(19.5271103794071,-1.05345495711953,124.012357050828));
#55852=CARTESIAN_POINT('Ctrl Pts',(19.7569163431838,-0.716570316510549,
124.037337521724));
#55853=CARTESIAN_POINT('Ctrl Pts',(19.8842721919957,-0.406132863032926,
124.058124610392));
#55854=CARTESIAN_POINT('Ctrl Pts',(19.9468983857731,-0.0912051795872804,
124.077845882252));
#55855=CARTESIAN_POINT('Ctrl Pts',(19.9128060685492,0.312131110791157,124.102708347526));
#55856=CARTESIAN_POINT('Ctrl Pts',(19.7686968044805,0.689516156019462,124.12752086565));
#55857=CARTESIAN_POINT('Ctrl Pts',(19.5262222384832,1.01161051681084,124.152283309869));
#55858=CARTESIAN_POINT('Ctrl Pts',(19.2047436092611,1.25346719763061,124.176994654029));
#55859=CARTESIAN_POINT('Ctrl Pts',(18.8608700518071,1.38470264636897,124.199599471414));
#55860=CARTESIAN_POINT('Ctrl Pts',(18.5307429560582,1.42405810218505,124.220111266288));
#55861=CARTESIAN_POINT('Ctrl Pts',(18.1339511090329,1.38805442878169,124.244685991001));
#55862=CARTESIAN_POINT('Ctrl Pts',(17.6701428523837,1.1882073001127,124.275329590867));
#55863=CARTESIAN_POINT('Ctrl Pts',(17.2614772001437,0.743236175006286,124.311980647433));
#55864=CARTESIAN_POINT('Ctrl Pts',(17.0708207279897,0.172186327797883,124.348508410227));
#55865=CARTESIAN_POINT('Ctrl Pts',(17.1298493738262,-0.424934717672883,
124.384911209635));
#55866=CARTESIAN_POINT('Ctrl Pts',(17.4265801116394,-0.944023464590011,
124.421187316989));
#55867=CARTESIAN_POINT('Ctrl Pts',(17.9077483098367,-1.29540685305693,124.457335165658));
#55868=CARTESIAN_POINT('Ctrl Pts',(18.4883777457567,-1.41915590235369,124.493353235692));
#55869=CARTESIAN_POINT('Ctrl Pts',(19.0667970754498,-1.29541084050984,124.529240117323));
#55870=CARTESIAN_POINT('Ctrl Pts',(19.5424601631271,-0.947491030561093,
124.564994478041));
#55871=CARTESIAN_POINT('Ctrl Pts',(19.8334367279826,-0.437548507507534,
124.600615080923));
#55872=CARTESIAN_POINT('Ctrl Pts',(19.890532162967,0.144554159051283,124.636100776618));
#55873=CARTESIAN_POINT('Ctrl Pts',(19.7056002759952,0.697081689981892,124.671450509215));
#55874=CARTESIAN_POINT('Ctrl Pts',(19.31264694973,1.1242227099732,124.706663314447));
#55875=CARTESIAN_POINT('Ctrl Pts',(18.7815879028084,1.35271038509035,124.741738321289));
#55876=CARTESIAN_POINT('Ctrl Pts',(18.2058055231885,1.34439292496962,124.776674751525));
#55877=CARTESIAN_POINT('Ctrl Pts',(17.6857205110023,1.10259169434594,124.81147192126));
#55878=CARTESIAN_POINT('Ctrl Pts',(17.3112703623074,0.671193369840806,124.84612924114));
#55879=CARTESIAN_POINT('Ctrl Pts',(17.1463529681068,0.126691569128493,124.880646216948));
#55880=CARTESIAN_POINT('Ctrl Pts',(17.2179263446672,-0.435378650074446,
124.915022449439));
#55881=CARTESIAN_POINT('Ctrl Pts',(17.51162287668,-0.917207316201509,124.949257634716));
#55882=CARTESIAN_POINT('Ctrl Pts',(17.9745869037968,-1.23573305878125,124.983351564605));
#55883=CARTESIAN_POINT('Ctrl Pts',(18.5249812919712,-1.33696044526901,125.017304127033));
#55884=CARTESIAN_POINT('Ctrl Pts',(19.0664533911177,-1.20510407231254,125.05111530585));
#55885=CARTESIAN_POINT('Ctrl Pts',(19.5050030607281,-0.865013250071704,
125.08478518061));
#55886=CARTESIAN_POINT('Ctrl Pts',(19.7652995061654,-0.377512664504211,
125.118313926678));
#55887=CARTESIAN_POINT('Ctrl Pts',(19.8036148445623,0.171470264339861,125.151701815308));
#55888=CARTESIAN_POINT('Ctrl Pts',(19.6151555861472,0.68604789282707,125.184949213517));
#55889=CARTESIAN_POINT('Ctrl Pts',(19.2345664267479,1.0771164944424,125.218056583602));
#55890=CARTESIAN_POINT('Ctrl Pts',(18.7295776788037,1.2777789898754,125.251024482545));
#55891=CARTESIAN_POINT('Ctrl Pts',(18.1889590277654,1.25477807637706,125.283853562006));
#55892=CARTESIAN_POINT('Ctrl Pts',(17.7069217162722,1.01398801261303,125.316544568073));
#55893=CARTESIAN_POINT('Ctrl Pts',(17.3667091947938,0.599062987557933,125.349098340655));
#55894=CARTESIAN_POINT('Ctrl Pts',(17.2262326256709,0.0835362323822979,
125.381515812706));
#55895=CARTESIAN_POINT('Ctrl Pts',(17.3082274780863,-0.442201849037498,
125.413798009192));
#55896=CARTESIAN_POINT('Ctrl Pts',(17.5966013589314,-0.886741847862278,
125.445946047028));
#55897=CARTESIAN_POINT('Ctrl Pts',(18.0395538508959,-1.17353593875436,125.477961134467));
#55898=CARTESIAN_POINT('Ctrl Pts',(18.5588683493257,-1.25406427559042,125.509844570104));
#55899=CARTESIAN_POINT('Ctrl Pts',(19.0637106321298,-1.11602592841314,125.541597741769));
#55900=CARTESIAN_POINT('Ctrl Pts',(19.4665019523936,-0.785175599263413,
125.573222125044));
#55901=CARTESIAN_POINT('Ctrl Pts',(19.6980954335397,-0.320540839004115,
125.604719283131));
#55902=CARTESIAN_POINT('Ctrl Pts',(19.7196286151713,0.196094904948042,125.636090865987));
#55903=CARTESIAN_POINT('Ctrl Pts',(19.5290243381413,0.674571056739599,125.667338608869));
#55904=CARTESIAN_POINT('Ctrl Pts',(19.161057269751,1.03206511272243,125.698464330996));
#55905=CARTESIAN_POINT('Ctrl Pts',(18.6810272845914,1.20740872383971,125.729469933572));
#55906=CARTESIAN_POINT('Ctrl Pts',(18.1731880784998,1.17153389999086,125.760357399525));
#55907=CARTESIAN_POINT('Ctrl Pts',(17.7259793640479,0.932269103252213,125.791128792605));
#55908=CARTESIAN_POINT('Ctrl Pts',(17.4166481460682,0.532699142812196,125.821786255271));
#55909=CARTESIAN_POINT('Ctrl Pts',(17.2979289089794,0.0434238889981436,
125.852332007358));
#55910=CARTESIAN_POINT('Ctrl Pts',(17.3890747127762,-0.449895700330302,
125.882768343437));
#55911=CARTESIAN_POINT('Ctrl Pts',(17.6727604197615,-0.861510746724262,
125.913097632608));
#55912=CARTESIAN_POINT('Ctrl Pts',(18.0983508923542,-1.12046324618725,125.943322317335));
#55913=CARTESIAN_POINT('Ctrl Pts',(18.5909205460674,-1.18279337377893,125.973444911086));
#55914=CARTESIAN_POINT('Ctrl Pts',(19.064420089077,-1.03898045127023,126.003467996632));
#55915=CARTESIAN_POINT('Ctrl Pts',(19.4366807791309,-0.715362751697529,
126.033394223096));
#55916=CARTESIAN_POINT('Ctrl Pts',(19.6436450174629,-0.269331625013446,
126.063226305569));
#55917=CARTESIAN_POINT('Ctrl Pts',(19.6503634796231,0.220825607772631,126.092967023883));
#55918=CARTESIAN_POINT('Ctrl Pts',(19.4568759059551,0.669639021035746,126.122619219901));
#55919=CARTESIAN_POINT('Ctrl Pts',(19.0979908142443,0.999328230901447,126.152185795611));
#55920=CARTESIAN_POINT('Ctrl Pts',(18.6370406771027,1.15325141249116,126.181669709829));
#55921=CARTESIAN_POINT('Ctrl Pts',(18.1547300638473,1.10561141161178,126.211073977686));
#55922=CARTESIAN_POINT('Ctrl Pts',(17.7350366382869,0.865760124565423,126.240401669216));
#55923=CARTESIAN_POINT('Ctrl Pts',(17.4506232868768,0.476387237297481,126.269655906651));
#55924=CARTESIAN_POINT('Ctrl Pts',(17.3502891400616,0.00594117354873083,
126.298839861967));
#55925=CARTESIAN_POINT('Ctrl Pts',(17.4506205281827,-0.463375181533064,
126.327956753676));
#55926=CARTESIAN_POINT('Ctrl Pts',(17.7332657943092,-0.849933821163535,
126.3570098459));
#55927=CARTESIAN_POINT('Ctrl Pts',(18.1482785980622,-1.08684381320572,126.386002446982));
#55928=CARTESIAN_POINT('Ctrl Pts',(18.6229220125094,-1.13349526950984,126.414937906657));
#55929=CARTESIAN_POINT('Ctrl Pts',(19.0743847326823,-0.982499015596272,
126.4438196133));
#55930=CARTESIAN_POINT('Ctrl Pts',(19.424192069326,-0.660840549056361,126.472650990649));
#55931=CARTESIAN_POINT('Ctrl Pts',(19.6118106557014,-0.225071250741804,
126.501435496495));
#55932=CARTESIAN_POINT('Ctrl Pts',(19.6050944907734,0.248608474895961,126.530176621242));
#55933=CARTESIAN_POINT('Ctrl Pts',(19.4057746373271,0.677638998879331,126.558877885567));
#55934=CARTESIAN_POINT('Ctrl Pts',(19.0490596952358,0.987451960857726,126.587542836246));
#55935=CARTESIAN_POINT('Ctrl Pts',(18.597433005056,1.12439519713685,126.616175045175));
#55936=CARTESIAN_POINT('Ctrl Pts',(18.1297382366635,1.06499687702138,126.644778103328));
#55937=CARTESIAN_POINT('Ctrl Pts',(17.7274508894903,0.819976494804396,126.673355627513));
#55938=CARTESIAN_POINT('Ctrl Pts',(17.46052738614,0.432314452937021,126.701911243189));
#55939=CARTESIAN_POINT('Ctrl Pts',(17.3752688798186,-0.0302622593028861,
126.730448607546));
#55940=CARTESIAN_POINT('Ctrl Pts',(17.4863236298534,-0.4870874654627,126.758971357521));
#55941=CARTESIAN_POINT('Ctrl Pts',(17.7741583266334,-0.858567970464191,
126.787483198642));
#55942=CARTESIAN_POINT('Ctrl Pts',(18.1885215296499,-1.08004071358368,126.815987733931));
#55943=CARTESIAN_POINT('Ctrl Pts',(18.6571227528184,-1.11294273911574,126.84448878));
#55944=CARTESIAN_POINT('Ctrl Pts',(19.0983396321036,-0.951607216982945,
126.87298976346));
#55945=CARTESIAN_POINT('Ctrl Pts',(19.3790073574672,-0.678636495961043,
126.896744018428));
#55946=CARTESIAN_POINT('Ctrl Pts',(19.5220836903997,-0.405756943585032,
126.915750760586));
#55947=CARTESIAN_POINT('Ctrl Pts',(19.6056047918582,-0.109116596200933,
126.934761112833));
#55948=CARTESIAN_POINT('Ctrl Pts',(19.5891990596196,0.282305480414591,126.958530471191));
#55949=CARTESIAN_POINT('Ctrl Pts',(19.3791775936598,0.703224821732214,126.987068898185));
#55950=CARTESIAN_POINT('Ctrl Pts',(19.0153693298559,1.00184926778107,127.015625598023));
#55951=CARTESIAN_POINT('Ctrl Pts',(18.5609439856181,1.12593517559301,127.044204512567));
#55952=CARTESIAN_POINT('Ctrl Pts',(18.0950635602875,1.05353232660813,127.072809113128));
#55953=CARTESIAN_POINT('Ctrl Pts',(17.6989714968607,0.796900190380831,127.101443096007));
#55954=CARTESIAN_POINT('Ctrl Pts',(17.4419485246998,0.400416874555999,127.13011000932));
#55955=CARTESIAN_POINT('Ctrl Pts',(17.3691828511564,-0.0670598713129301,
127.158813447632));
#55956=CARTESIAN_POINT('Ctrl Pts',(17.4938709051282,-0.524124201025331,
127.18755694342));
#55957=CARTESIAN_POINT('Ctrl Pts',(17.7948197733865,-0.890955803526526,
127.216344020369));
#55958=CARTESIAN_POINT('Ctrl Pts',(18.2200428622329,-1.10322448511446,127.245178163347));
#55959=CARTESIAN_POINT('Ctrl Pts',(18.6957109311462,-1.12334093168554,127.274062831572));
#55960=CARTESIAN_POINT('Ctrl Pts',(19.1389377379455,-0.947095772661866,
127.303001446521));
#55961=CARTESIAN_POINT('Ctrl Pts',(19.4721844503801,-0.604515201648737,
127.331997395638));
#55962=CARTESIAN_POINT('Ctrl Pts',(19.6367900836946,-0.154763370218899,
127.361054019705));
#55963=CARTESIAN_POINT('Ctrl Pts',(19.6032731046921,0.324047256434558,127.390174640306));
#55964=CARTESIAN_POINT('Ctrl Pts',(19.3765936226467,0.748387713713813,127.419362477709));
#55965=CARTESIAN_POINT('Ctrl Pts',(18.99545138893,1.04384901099861,127.448620841323));
#55966=CARTESIAN_POINT('Ctrl Pts',(18.5256921328986,1.15815663876935,127.477952723227));
#55967=CARTESIAN_POINT('Ctrl Pts',(18.0489718439953,1.07040199940171,127.507361577771));
#55968=CARTESIAN_POINT('Ctrl Pts',(17.6485849520916,0.794842800013771,127.536849772547));
#55969=CARTESIAN_POINT('Ctrl Pts',(17.3949567046523,0.378620118062738,127.566421855019));
#55970=CARTESIAN_POINT('Ctrl Pts',(17.3332559961865,-0.106295560388526,
127.596077582544));
#55971=CARTESIAN_POINT('Ctrl Pts',(17.4754687696325,-0.575519789631179,
127.6258257653));
#55972=CARTESIAN_POINT('Ctrl Pts',(17.7977855400058,-0.9468941024104,127.655659616253));
#55973=CARTESIAN_POINT('Ctrl Pts',(18.2453408438712,-1.15482413737233,127.685596661067));
#55974=CARTESIAN_POINT('Ctrl Pts',(18.7399637910724,-1.16200183707374,127.715615510269));
#55975=CARTESIAN_POINT('Ctrl Pts',(19.1964401094813,-0.965517772876336,
127.745762596965));
#55976=CARTESIAN_POINT('Ctrl Pts',(19.5336962630831,-0.599252394510159,
127.775963740483));
#55977=CARTESIAN_POINT('Ctrl Pts',(19.6915929912239,-0.124428463739348,
127.806325164134));
#55978=CARTESIAN_POINT('Ctrl Pts',(19.6524076589129,0.291505836798268,127.831711772845));
#55979=CARTESIAN_POINT('Ctrl Pts',(19.5191279816085,0.592593656833114,127.851988567495));
#55980=CARTESIAN_POINT('Ctrl Pts',(19.3724951349617,0.794645357387739,127.867306889191));
#55981=CARTESIAN_POINT('Ctrl Pts',(19.1874613302448,0.962053453799274,127.882681906434));
#55982=CARTESIAN_POINT('Ctrl Pts',(18.9757369246924,1.08607203149486,127.89802598822));
#55983=CARTESIAN_POINT('Ctrl Pts',(18.7443752728392,1.16211632557479,127.913317040423));
#55984=CARTESIAN_POINT('Ctrl Pts',(18.5765564222551,1.18031848976882,127.923609419278));
#55985=CARTESIAN_POINT('Ctrl Pts',(18.4888644293293,1.18105655666575,127.928800510495));
#55986=CARTESIAN_POINT('Ctrl Pts',(18.488182152249,1.29990053410893,112.700349483895));
#55987=CARTESIAN_POINT('Ctrl Pts',(18.3444976430382,1.29869120157713,112.70885515658));
#55988=CARTESIAN_POINT('Ctrl Pts',(18.1626414086569,1.26954424100949,112.72020028386));
#55989=CARTESIAN_POINT('Ctrl Pts',(17.9105741471188,1.1715572059241,112.7372275449));
#55990=CARTESIAN_POINT('Ctrl Pts',(17.7147016928909,1.05680544825268,112.75142581384));
#55991=CARTESIAN_POINT('Ctrl Pts',(17.5092914781924,0.870936460786282,112.768496063499));
#55992=CARTESIAN_POINT('Ctrl Pts',(17.3452643787265,0.645338607702756,112.785608543142));
#55993=CARTESIAN_POINT('Ctrl Pts',(17.1949694671818,0.305633664533222,112.808486356608));
#55994=CARTESIAN_POINT('Ctrl Pts',(17.1504041586296,-0.163958059400556,
112.8371493128));
#55995=CARTESIAN_POINT('Ctrl Pts',(17.3295581344551,-0.704127606930189,
112.871679546659));
#55996=CARTESIAN_POINT('Ctrl Pts',(17.7163063911852,-1.12497913550319,112.906352649458));
#55997=CARTESIAN_POINT('Ctrl Pts',(18.2431925961433,-1.35205912276461,112.941152109412));
#55998=CARTESIAN_POINT('Ctrl Pts',(18.8187741112765,-1.34427642838518,112.976089285723));
#55999=CARTESIAN_POINT('Ctrl Pts',(19.3432395618757,-1.10098396627254,113.011156346434));
#56000=CARTESIAN_POINT('Ctrl Pts',(19.7238494382154,-0.663159822701633,
113.046357078694));
#56001=CARTESIAN_POINT('Ctrl Pts',(19.8931314314799,-0.105956319615994,
113.08168722595));
#56002=CARTESIAN_POINT('Ctrl Pts',(19.8197719071333,0.473908286429459,113.117148366555));
#56003=CARTESIAN_POINT('Ctrl Pts',(19.514861434432,0.975046989864885,113.152737815001));
#56004=CARTESIAN_POINT('Ctrl Pts',(19.0301258646803,1.30913564752012,113.188455340763));
#56005=CARTESIAN_POINT('Ctrl Pts',(18.4491549165285,1.416472562517,113.224299311997));
#56006=CARTESIAN_POINT('Ctrl Pts',(17.8730091730699,1.27666467315962,113.260268611474));
#56007=CARTESIAN_POINT('Ctrl Pts',(17.4026034483492,0.912474225359778,113.296361769111));
#56008=CARTESIAN_POINT('Ctrl Pts',(17.1210280345443,0.386131812194797,113.332577359437));
#56009=CARTESIAN_POINT('Ctrl Pts',(17.0788544181136,-0.211299879373549,
113.368913814958));
#56010=CARTESIAN_POINT('Ctrl Pts',(17.2850565553758,-0.775695991436841,
113.405369493798));
#56011=CARTESIAN_POINT('Ctrl Pts',(17.705146965038,-1.20803167965084,113.441942712263));
#56012=CARTESIAN_POINT('Ctrl Pts',(18.2669652505624,-1.43177932086286,113.478631613973));
#56013=CARTESIAN_POINT('Ctrl Pts',(18.8730309513044,-1.40645905314605,113.51543444437));
#56014=CARTESIAN_POINT('Ctrl Pts',(19.4175618056869,-1.13497091574588,113.55234907248));
#56015=CARTESIAN_POINT('Ctrl Pts',(19.8048480383929,-0.663350581086933,
113.589373656825));
#56016=CARTESIAN_POINT('Ctrl Pts',(19.966197057422,-0.0729778537808475,
113.626505971993));
#56017=CARTESIAN_POINT('Ctrl Pts',(19.8720657245217,0.533549954628291,113.663743893195));
#56018=CARTESIAN_POINT('Ctrl Pts',(19.5374817640394,1.0501311842453,113.701085198819));
#56019=CARTESIAN_POINT('Ctrl Pts',(19.0196808505253,1.38594482959087,113.738527490934));
#56020=CARTESIAN_POINT('Ctrl Pts',(18.5101754020758,1.46526119175664,113.769811704289));
#56021=CARTESIAN_POINT('Ctrl Pts',(18.1090240872925,1.39960741569811,113.794887075397));
#56022=CARTESIAN_POINT('Ctrl Pts',(17.729655069815,1.25220225914757,113.819994103033));
#56023=CARTESIAN_POINT('Ctrl Pts',(17.3289300722954,0.923586877948104,113.851436567131));
#56024=CARTESIAN_POINT('Ctrl Pts',(17.0504721252432,0.365805609893722,113.889258509496));
#56025=CARTESIAN_POINT('Ctrl Pts',(17.0240290762783,-0.258477757917008,
113.927168961164));
#56026=CARTESIAN_POINT('Ctrl Pts',(17.2554238425403,-0.840447617959809,
113.965165177094));
#56027=CARTESIAN_POINT('Ctrl Pts',(17.7053131011304,-1.27808626113464,114.003244380208));
#56028=CARTESIAN_POINT('Ctrl Pts',(18.2959641544648,-1.49425702735341,114.041403784502));
#56029=CARTESIAN_POINT('Ctrl Pts',(18.9246622805112,-1.4502272181577,114.079640512388));
#56030=CARTESIAN_POINT('Ctrl Pts',(19.4816239236303,-1.15267110135651,114.117951609114));
#56031=CARTESIAN_POINT('Ctrl Pts',(19.8691907107327,-0.652639427392253,
114.156334167846));
#56032=CARTESIAN_POINT('Ctrl Pts',(20.0189810591327,-0.03683256961316,114.194785080069));
#56033=CARTESIAN_POINT('Ctrl Pts',(19.9039833865991,0.587522999416328,114.2333013558));
#56034=CARTESIAN_POINT('Ctrl Pts',(19.5434230734537,1.11127572106957,114.271879839515));
#56035=CARTESIAN_POINT('Ctrl Pts',(18.9995399107886,1.44259279852258,114.310517384521));
#56036=CARTESIAN_POINT('Ctrl Pts',(18.3668596633944,1.52297273199859,114.349210799966));
#56037=CARTESIAN_POINT('Ctrl Pts',(17.7556977562459,1.33767203016567,114.387956849117));
#56038=CARTESIAN_POINT('Ctrl Pts',(17.272914349715,0.918370107647551,114.426752263094));
#56039=CARTESIAN_POINT('Ctrl Pts',(17.0031861863323,0.337753138207008,114.46559374694));
#56040=CARTESIAN_POINT('Ctrl Pts',(16.9941242219495,-0.303088855509916,
114.504477951706));
#56041=CARTESIAN_POINT('Ctrl Pts',(17.2478715429229,-0.892350566926149,
114.543401543985));
#56042=CARTESIAN_POINT('Ctrl Pts',(17.720592505509,-1.32694200600498,114.582361077963));
#56043=CARTESIAN_POINT('Ctrl Pts',(18.3301332049521,-1.53077558802408,114.621353247865));
#56044=CARTESIAN_POINT('Ctrl Pts',(18.8635057740616,-1.47820468577621,114.653870882415));
#56045=CARTESIAN_POINT('Ctrl Pts',(19.2496685905278,-1.30821665552171,114.679897931973));
#56046=CARTESIAN_POINT('Ctrl Pts',(19.5923918636366,-1.06191387672613,114.705932982827));
#56047=CARTESIAN_POINT('Ctrl Pts',(19.9091081456583,-0.628734129737697,
114.738490494062));
#56048=CARTESIAN_POINT('Ctrl Pts',(20.0436482399265,0.00136013336455928,
114.777578396996));
#56049=CARTESIAN_POINT('Ctrl Pts',(19.9090928165798,0.631655323772199,114.816681421648));
#56050=CARTESIAN_POINT('Ctrl Pts',(19.5286868815429,1.1521949790643,114.855796201813));
#56051=CARTESIAN_POINT('Ctrl Pts',(18.9687372623033,1.47200625927751,114.894919129408));
#56052=CARTESIAN_POINT('Ctrl Pts',(18.3269247722238,1.53523233022917,114.934046750203));
#56053=CARTESIAN_POINT('Ctrl Pts',(17.7152334288248,1.33076841613399,114.973175454517));
#56054=CARTESIAN_POINT('Ctrl Pts',(17.2404725580255,0.894349558877001,115.012301840373));
#56055=CARTESIAN_POINT('Ctrl Pts',(16.9853446354984,0.302108848816737,115.051422158546));
#56056=CARTESIAN_POINT('Ctrl Pts',(16.9934993376988,-0.27079628228924,115.086187634404));
#56057=CARTESIAN_POINT('Ctrl Pts',(17.1704122775008,-0.733300276011371,
115.116598560424));
#56058=CARTESIAN_POINT('Ctrl Pts',(17.3615831320585,-0.98758491633179,115.136144037193));
#56059=CARTESIAN_POINT('Ctrl Pts',(17.5154254407977,-1.13081668225498,115.149171118788));
#56060=CARTESIAN_POINT('Ctrl Pts',(17.5970581795022,-1.19692836165928,115.155684477762));
#56061=CARTESIAN_POINT('Ctrl Pts',(17.6831967780099,-1.25709479715135,115.162197134421));
#56062=CARTESIAN_POINT('Ctrl Pts',(17.8633620834074,-1.36516570458449,115.175222025971));
#56063=CARTESIAN_POINT('Ctrl Pts',(18.1604819038664,-1.47854845945174,115.194753812955));
#56064=CARTESIAN_POINT('Ctrl Pts',(18.582786890695,-1.51417568969967,115.220787745291));
#56065=CARTESIAN_POINT('Ctrl Pts',(18.9983836416472,-1.43149328105734,115.246809679889));
#56066=CARTESIAN_POINT('Ctrl Pts',(19.374473528925,-1.23714016652633,115.27282057109));
#56067=CARTESIAN_POINT('Ctrl Pts',(19.6822598946567,-0.946311359030486,
115.298817689622));
#56068=CARTESIAN_POINT('Ctrl Pts',(19.8967480474023,-0.582015055171165,
115.324801432878));
#56069=CARTESIAN_POINT('Ctrl Pts',(20.0386193688326,-0.0359715504243672,
115.359425895719));
#56070=CARTESIAN_POINT('Ctrl Pts',(19.941536265269,0.535299448860012,115.394018366274));
#56071=CARTESIAN_POINT('Ctrl Pts',(19.6668198938765,0.944384240575756,115.424255526598));
#56072=CARTESIAN_POINT('Ctrl Pts',(19.4671125145751,1.13894829771433,115.44152396901));
#56073=CARTESIAN_POINT('Ctrl Pts',(19.2416596715355,1.3035791132569,115.458786271138));
#56074=CARTESIAN_POINT('Ctrl Pts',(19.0175256336374,1.40399060754221,115.473882214218));
#56075=CARTESIAN_POINT('Ctrl Pts',(18.8150509122225,1.45460978349152,115.486814484407));
#56076=CARTESIAN_POINT('Ctrl Pts',(18.7124011810244,1.4728082953005,115.493279478184));
#56077=CARTESIAN_POINT('Ctrl Pts',(18.6259805295674,1.48196183269604,115.498665769091));
#56078=CARTESIAN_POINT('Ctrl Pts',(18.5565983881251,1.48554743331276,115.502974301951));
#56079=CARTESIAN_POINT('Ctrl Pts',(18.275006635137,1.49093350233563,115.520445423601));
#56080=CARTESIAN_POINT('Ctrl Pts',(17.7643189677256,1.36044159259875,115.552131188091));
#56081=CARTESIAN_POINT('Ctrl Pts',(17.3297966145357,0.957318076594017,115.587783846009));
#56082=CARTESIAN_POINT('Ctrl Pts',(17.1366050542202,0.593850002954031,115.613220643608));
#56083=CARTESIAN_POINT('Ctrl Pts',(17.0708721336454,0.399095376421441,115.625931295202));
#56084=CARTESIAN_POINT('Ctrl Pts',(17.0385717481457,0.238286256682236,115.636095006768));
#56085=CARTESIAN_POINT('Ctrl Pts',(17.0000053948983,-0.0873641069959773,
115.656416799589));
#56086=CARTESIAN_POINT('Ctrl Pts',(17.0954817402936,-0.627463061463085,
115.689403138097));
#56087=CARTESIAN_POINT('Ctrl Pts',(17.5683032047114,-1.2202390337612,115.734986014693));
#56088=CARTESIAN_POINT('Ctrl Pts',(18.2073749791171,-1.48915585063008,115.776682365231));
#56089=CARTESIAN_POINT('Ctrl Pts',(18.827714255502,-1.46536270236631,115.81451460932));
#56090=CARTESIAN_POINT('Ctrl Pts',(19.3387291215206,-1.24252555435953,115.848504801486));
#56091=CARTESIAN_POINT('Ctrl Pts',(19.7323390465761,-0.84870905484788,115.882433969696));
#56092=CARTESIAN_POINT('Ctrl Pts',(19.917317868452,-0.424382854990528,115.910656120296));
#56093=CARTESIAN_POINT('Ctrl Pts',(19.9647758151583,-0.0623666971425709,
115.933200950891));
#56094=CARTESIAN_POINT('Ctrl Pts',(19.9494967945027,0.210678396553568,115.950093741532));
#56095=CARTESIAN_POINT('Ctrl Pts',(19.8946537689314,0.431722595099945,115.964156440341));
#56096=CARTESIAN_POINT('Ctrl Pts',(19.8267524040723,0.599946781165768,115.975398400255));
#56097=CARTESIAN_POINT('Ctrl Pts',(19.7020401592803,0.841706463647344,115.992253058882));
#56098=CARTESIAN_POINT('Ctrl Pts',(19.4317853790293,1.15561589179994,116.017502153899));
#56099=CARTESIAN_POINT('Ctrl Pts',(18.9444409086331,1.41307035879397,116.051097502054));
#56100=CARTESIAN_POINT('Ctrl Pts',(18.3979015457458,1.47453073660614,116.084620132269));
#56101=CARTESIAN_POINT('Ctrl Pts',(18.0004069582635,1.36793073631313,116.1097063674));
#56102=CARTESIAN_POINT('Ctrl Pts',(17.763366663899,1.23962198295239,116.126406802779));
#56103=CARTESIAN_POINT('Ctrl Pts',(17.6140480708204,1.1398854968943,116.137534246267));
#56104=CARTESIAN_POINT('Ctrl Pts',(17.3790836560323,0.929981622126309,116.156989690435));
#56105=CARTESIAN_POINT('Ctrl Pts',(17.2215832331742,0.679602546844773,116.175024509631));
#56106=CARTESIAN_POINT('Ctrl Pts',(17.1450352066694,0.469669982396278,116.188878617737));
#56107=CARTESIAN_POINT('Ctrl Pts',(17.1249441446997,0.405767087289566,116.193033537477));
#56108=CARTESIAN_POINT('Ctrl Pts',(17.1079301441042,0.340970796669862,116.197187251518));
#56109=CARTESIAN_POINT('Ctrl Pts',(17.0939473695056,0.275494153967272,116.201339691278));
#56110=CARTESIAN_POINT('Ctrl Pts',(17.0830227708597,0.209443458520346,116.205490910608));
#56111=CARTESIAN_POINT('Ctrl Pts',(17.0726655652121,0.120824547382831,116.211024197657));
#56112=CARTESIAN_POINT('Ctrl Pts',(17.0610173800014,-0.124379540531134,
116.226234061721));
#56113=CARTESIAN_POINT('Ctrl Pts',(17.1369245229291,-0.5249310381429,116.251084258337));
#56114=CARTESIAN_POINT('Ctrl Pts',(17.4255200195769,-0.984001270082908,
116.284135719174));
#56115=CARTESIAN_POINT('Ctrl Pts',(17.8607605682645,-1.30506353431624,116.317102617813));
#56116=CARTESIAN_POINT('Ctrl Pts',(18.3818866043649,-1.44455243472689,116.349983938512));
#56117=CARTESIAN_POINT('Ctrl Pts',(18.916470350186,-1.38418902476214,116.382777928971));
#56118=CARTESIAN_POINT('Ctrl Pts',(19.3908578736671,-1.13333494037052,116.415483428707));
#56119=CARTESIAN_POINT('Ctrl Pts',(19.662129258784,-0.817824110576332,116.440850810503));
#56120=CARTESIAN_POINT('Ctrl Pts',(19.7921004518703,-0.556121431420674,
116.458936888485));
#56121=CARTESIAN_POINT('Ctrl Pts',(19.8690655500124,-0.335782443963777,
116.473391787428));
#56122=CARTESIAN_POINT('Ctrl Pts',(19.9308282800101,0.0701141608640084,
116.498652513443));
#56123=CARTESIAN_POINT('Ctrl Pts',(19.7975561020439,0.653379656102897,116.534635638022));
#56124=CARTESIAN_POINT('Ctrl Pts',(19.3238121146665,1.18955843336623,116.577647401962));
#56125=CARTESIAN_POINT('Ctrl Pts',(18.6542573597491,1.43288587092525,116.620488268205));
#56126=CARTESIAN_POINT('Ctrl Pts',(17.9525424324882,1.32679118729713,116.663155847902));
#56127=CARTESIAN_POINT('Ctrl Pts',(17.4716228570456,0.961996366384522,116.699450989897));
#56128=CARTESIAN_POINT('Ctrl Pts',(17.2242845453766,0.540894020126181,116.729451046567));
#56129=CARTESIAN_POINT('Ctrl Pts',(17.0944240343639,0.041457592091441,116.761140226464));
#56130=CARTESIAN_POINT('Ctrl Pts',(17.2055334687691,-0.610901669378824,
116.8006093271));
#56131=CARTESIAN_POINT('Ctrl Pts',(17.7327235525077,-1.19996474577183,116.847741724244));
#56132=CARTESIAN_POINT('Ctrl Pts',(18.4886274023919,-1.41711476065944,116.894641370113));
#56133=CARTESIAN_POINT('Ctrl Pts',(19.2403913761961,-1.19999329817096,116.941306241231));
#56134=CARTESIAN_POINT('Ctrl Pts',(19.7589583230562,-0.618976305235332,
116.987734609023));
#56135=CARTESIAN_POINT('Ctrl Pts',(19.866303857657,0.0173456111094613,117.026226666982));
#56136=CARTESIAN_POINT('Ctrl Pts',(19.7405351404932,0.500732911611066,117.05690073817));
#56137=CARTESIAN_POINT('Ctrl Pts',(19.5511427517233,0.822664799957136,117.079846452937));
#56138=CARTESIAN_POINT('Ctrl Pts',(19.2800271222083,1.07822752115069,117.102732140544));
#56139=CARTESIAN_POINT('Ctrl Pts',(18.840099008821,1.30647550082486,117.13316636068));
#56140=CARTESIAN_POINT('Ctrl Pts',(18.2057864265544,1.34185814168128,117.171058787474));
#56141=CARTESIAN_POINT('Ctrl Pts',(17.5421074842011,0.974328602971076,117.216288928054));
#56142=CARTESIAN_POINT('Ctrl Pts',(17.1777038347398,0.313792671011465,117.261278280207));
#56143=CARTESIAN_POINT('Ctrl Pts',(17.2203225463522,-0.435464225919962,
117.306027156934));
#56144=CARTESIAN_POINT('Ctrl Pts',(17.652724667813,-1.04386133116569,117.350536141848));
#56145=CARTESIAN_POINT('Ctrl Pts',(18.3388239098277,-1.32745573236693,117.39480611765));
#56146=CARTESIAN_POINT('Ctrl Pts',(19.0667149711576,-1.20320856043253,117.438838249758));
#56147=CARTESIAN_POINT('Ctrl Pts',(19.6139786084161,-0.713397943859653,
117.482633994782));
#56148=CARTESIAN_POINT('Ctrl Pts',(19.8156811381899,-0.0112791664943189,
117.526195091984));
#56149=CARTESIAN_POINT('Ctrl Pts',(19.6140022601783,0.686784214414896,117.569523562413));
#56150=CARTESIAN_POINT('Ctrl Pts',(19.0747275941947,1.16798331893147,117.612621710931));
#56151=CARTESIAN_POINT('Ctrl Pts',(18.3658643708616,1.28788138840837,117.655492120034));
#56152=CARTESIAN_POINT('Ctrl Pts',(17.7053431257873,1.01371279747136,117.69813764302));
#56153=CARTESIAN_POINT('Ctrl Pts',(17.2940790801678,0.433188982502828,117.740561406275));
#56154=CARTESIAN_POINT('Ctrl Pts',(17.2549003691858,-0.273508324804743,
117.782766808914));
#56155=CARTESIAN_POINT('Ctrl Pts',(17.5959737510632,-0.889574255288579,
117.824757505323));
#56156=CARTESIAN_POINT('Ctrl Pts',(18.2094168755739,-1.22806570874149,117.866537413039));
#56157=CARTESIAN_POINT('Ctrl Pts',(18.9055013390443,-1.18847566627298,117.908110699435));
#56158=CARTESIAN_POINT('Ctrl Pts',(19.4709991235593,-0.786645501256251,
117.949481800211));
#56159=CARTESIAN_POINT('Ctrl Pts',(19.7349121554302,-0.148494032303403,
117.990655350317));
#56160=CARTESIAN_POINT('Ctrl Pts',(19.6384296844279,0.41595364745626,118.024806143826));
#56161=CARTESIAN_POINT('Ctrl Pts',(19.3912822005401,0.783910465160815,118.052032979065));
#56162=CARTESIAN_POINT('Ctrl Pts',(19.0539455301924,1.06997780245999,118.079198326187));
#56163=CARTESIAN_POINT('Ctrl Pts',(18.5086041618223,1.22692728472169,118.113040992046));
#56164=CARTESIAN_POINT('Ctrl Pts',(17.8570681242743,1.03871258992206,118.153475788182));
#56165=CARTESIAN_POINT('Ctrl Pts',(17.4074661243136,0.535028360348281,118.193739748399));
#56166=CARTESIAN_POINT('Ctrl Pts',(17.295184410072,-0.12802353903353,118.233838994046));
#56167=CARTESIAN_POINT('Ctrl Pts',(17.5518536435643,-0.746678185841251,
118.273779650817));
#56168=CARTESIAN_POINT('Ctrl Pts',(18.09623557474,-1.13252353284961,118.313568149567));
#56169=CARTESIAN_POINT('Ctrl Pts',(18.7600131800788,-1.16944565236424,118.353211038631));
#56170=CARTESIAN_POINT('Ctrl Pts',(19.3396804878931,-0.848740522078599,
118.392715097256));
#56171=CARTESIAN_POINT('Ctrl Pts',(19.6587833880623,-0.270665095166121,
118.432087186673));
#56172=CARTESIAN_POINT('Ctrl Pts',(19.6216208701028,0.386364157140476,118.471334476116));
#56173=CARTESIAN_POINT('Ctrl Pts',(19.2416211971827,0.921545428620454,118.510464030869));
#56174=CARTESIAN_POINT('Ctrl Pts',(18.7378784200697,1.12977499085113,118.542980260458));
#56175=CARTESIAN_POINT('Ctrl Pts',(18.3152260681784,1.11706291748731,118.56894164302));
#56176=CARTESIAN_POINT('Ctrl Pts',(18.013631331558,1.02122659296196,118.588388203893));
#56177=CARTESIAN_POINT('Ctrl Pts',(17.7507020897944,0.845342251383026,118.607810663731));
#56178=CARTESIAN_POINT('Ctrl Pts',(17.5469576086983,0.604112404067775,118.62721063314));
#56179=CARTESIAN_POINT('Ctrl Pts',(17.418115189222,0.316066123273868,118.646588439489));
#56180=CARTESIAN_POINT('Ctrl Pts',(17.3740914074908,0.00406156609269027,
118.665945648007));
#56181=CARTESIAN_POINT('Ctrl Pts',(17.418105330468,-0.307731076500601,118.68528270408));
#56182=CARTESIAN_POINT('Ctrl Pts',(17.5252095909573,-0.546868258948941,
118.701381492349));
#56183=CARTESIAN_POINT('Ctrl Pts',(17.6479384162453,-0.714878730507821,
118.714251085885));
#56184=CARTESIAN_POINT('Ctrl Pts',(17.7929243818857,-0.863723509943578,
118.727115583167));
#56185=CARTESIAN_POINT('Ctrl Pts',(18.0972164483336,-1.06793358028532,118.74961267773));
#56186=CARTESIAN_POINT('Ctrl Pts',(18.6276378637832,-1.15815365828481,118.781712261723));
#56187=CARTESIAN_POINT('Ctrl Pts',(19.2238118827329,-0.91106020954,118.820176086249));
#56188=CARTESIAN_POINT('Ctrl Pts',(19.5340790733567,-0.473298914368946,
118.852189669591));
#56189=CARTESIAN_POINT('Ctrl Pts',(19.6045033571726,-0.115359348913955,
118.874582530202));
#56190=CARTESIAN_POINT('Ctrl Pts',(19.6017475647411,0.0911640829913528,
118.88737350014));
#56191=CARTESIAN_POINT('Ctrl Pts',(19.5700196370974,0.29559108219492,118.900162446911));
#56192=CARTESIAN_POINT('Ctrl Pts',(19.4770780543413,0.538342967989427,118.916143236651));
#56193=CARTESIAN_POINT('Ctrl Pts',(19.2273588011135,0.871529045839169,118.941704029868));
#56194=CARTESIAN_POINT('Ctrl Pts',(18.7588367207674,1.13058490335296,118.973640684375));
#56195=CARTESIAN_POINT('Ctrl Pts',(18.1172887995021,1.09452313569986,119.011950738852));
#56196=CARTESIAN_POINT('Ctrl Pts',(17.593388380079,0.722780783019972,119.050254797413));
#56197=CARTESIAN_POINT('Ctrl Pts',(17.3886684004257,0.228286678671025,119.082177254148));
#56198=CARTESIAN_POINT('Ctrl Pts',(17.4011923319186,-0.187547154371747,
119.107720239302));
#56199=CARTESIAN_POINT('Ctrl Pts',(17.479741012236,-0.43518291567232,119.123688362763));
#56200=CARTESIAN_POINT('Ctrl Pts',(17.5695979738663,-0.592074644579124,
119.134867535548));
#56201=CARTESIAN_POINT('Ctrl Pts',(17.6297289359476,-0.675697287840335,
119.1412564699));
#56202=CARTESIAN_POINT('Ctrl Pts',(17.6957161316275,-0.754921963867992,
119.147645877012));
#56203=CARTESIAN_POINT('Ctrl Pts',(17.7882499830905,-0.84489988474299,119.155633946795));
#56204=CARTESIAN_POINT('Ctrl Pts',(17.9550205699679,-0.966828303763707,
119.168415926821));
#56205=CARTESIAN_POINT('Ctrl Pts',(18.1925073400234,-1.07312652027406,119.184398568056));
#56206=CARTESIAN_POINT('Ctrl Pts',(18.5018237176362,-1.11680179614521,119.203585076302));
#56207=CARTESIAN_POINT('Ctrl Pts',(18.8112727437243,-1.07312083019676,119.222781017226));
#56208=CARTESIAN_POINT('Ctrl Pts',(19.0966922989243,-0.945425429896232,
119.241986576724));
#56209=CARTESIAN_POINT('Ctrl Pts',(19.3357397025375,-0.743574694906012,
119.261203548649));
#56210=CARTESIAN_POINT('Ctrl Pts',(19.5096763702265,-0.483296157484075,
119.280432047793));
#56211=CARTESIAN_POINT('Ctrl Pts',(19.604829263032,-0.184805761734769,119.299674358162));
#56212=CARTESIAN_POINT('Ctrl Pts',(19.6136282032755,0.128548869667553,119.318929822438));
#56213=CARTESIAN_POINT('Ctrl Pts',(19.5483562428395,0.381754662526241,119.334989622353));
#56214=CARTESIAN_POINT('Ctrl Pts',(19.4555027014667,0.567586338753027,119.347844753828));
#56215=CARTESIAN_POINT('Ctrl Pts',(19.3083285466207,0.781707993580481,119.363921119013));
#56216=CARTESIAN_POINT('Ctrl Pts',(19.0213883195784,1.0173014385066,119.386447876364));
#56217=CARTESIAN_POINT('Ctrl Pts',(18.5601806816014,1.14326482672377,119.415452744608));
#56218=CARTESIAN_POINT('Ctrl Pts',(18.0870469004768,1.06976794361554,119.444502870166));
#56219=CARTESIAN_POINT('Ctrl Pts',(17.6845073765261,0.809000046868888,119.473601565479));
#56220=CARTESIAN_POINT('Ctrl Pts',(17.4231181242213,0.405838898540841,119.502752060927));
#56221=CARTESIAN_POINT('Ctrl Pts',(17.3490598832109,-0.0697983875198877,
119.531957712525));
#56222=CARTESIAN_POINT('Ctrl Pts',(17.4759534440631,-0.535171725229621,
119.561221496182));
#56223=CARTESIAN_POINT('Ctrl Pts',(17.7314548399343,-0.846550437506931,
119.58565944407));
#56224=CARTESIAN_POINT('Ctrl Pts',(17.999207559364,-1.0170868157945,119.605241751292));
#56225=CARTESIAN_POINT('Ctrl Pts',(18.2967905723551,-1.12863703662001,119.624846422395));
#56226=CARTESIAN_POINT('Ctrl Pts',(18.701022235534,-1.14581433888424,119.649394327387));
#56227=CARTESIAN_POINT('Ctrl Pts',(19.1533010528138,-0.965969567310355,
119.678922596865));
#56228=CARTESIAN_POINT('Ctrl Pts',(19.4935242230618,-0.616264784255005,
119.708524488639));
#56229=CARTESIAN_POINT('Ctrl Pts',(19.6616806751607,-0.15688731828813,119.738203011753));
#56230=CARTESIAN_POINT('Ctrl Pts',(19.6274500840142,0.332402173060607,119.767961008938));
#56231=CARTESIAN_POINT('Ctrl Pts',(19.3957290628344,0.766238455283539,119.797801335606));
#56232=CARTESIAN_POINT('Ctrl Pts',(19.0059018782433,1.06845895995986,119.827726746298));
#56233=CARTESIAN_POINT('Ctrl Pts',(18.5252515327408,1.18543071772727,119.857739979944));
#56234=CARTESIAN_POINT('Ctrl Pts',(18.037234743022,1.09564506473,119.887843657137));
#56235=CARTESIAN_POINT('Ctrl Pts',(17.6956019306827,0.860470084296629,119.913007640695));
#56236=CARTESIAN_POINT('Ctrl Pts',(17.4972936032911,0.600305772965447,119.93318661626));
#56237=CARTESIAN_POINT('Ctrl Pts',(17.3569038509229,0.304279815543778,119.953397785618));
#56238=CARTESIAN_POINT('Ctrl Pts',(17.3041660284991,-0.109796929925252,
119.978723169803));
#56239=CARTESIAN_POINT('Ctrl Pts',(17.4498994353956,-0.59078091166106,120.009214030095));
#56240=CARTESIAN_POINT('Ctrl Pts',(17.7804655429487,-0.971566966837065,
120.039807705564));
#56241=CARTESIAN_POINT('Ctrl Pts',(18.2393086861239,-1.18486584665598,120.07050641441));
#56242=CARTESIAN_POINT('Ctrl Pts',(18.7470163437987,-1.1921729938516,120.101312384752));
#56243=CARTESIAN_POINT('Ctrl Pts',(19.215087635489,-0.990765643040621,120.132227714623));
#56244=CARTESIAN_POINT('Ctrl Pts',(19.5613155231427,-0.614392148089554,
120.163254460057));
#56245=CARTESIAN_POINT('Ctrl Pts',(19.7242152497417,-0.127659401515012,
120.194394583265));
#56246=CARTESIAN_POINT('Ctrl Pts',(19.6739207775415,0.385049104109546,120.225649979257));
#56247=CARTESIAN_POINT('Ctrl Pts',(19.4176458057697,0.834175476321175,120.257022460356));
#56248=CARTESIAN_POINT('Ctrl Pts',(18.998699632526,1.14061462596676,120.288513762116));
#56249=CARTESIAN_POINT('Ctrl Pts',(18.4891879156563,1.24962833189955,120.320125537776));
#56250=CARTESIAN_POINT('Ctrl Pts',(17.9776202690671,1.14060959036587,120.351859359126));
#56251=CARTESIAN_POINT('Ctrl Pts',(17.5535525982464,0.830952823101709,120.383716714854));
#56252=CARTESIAN_POINT('Ctrl Pts',(17.2919248389954,0.373308289212946,120.415699010712));
#56253=CARTESIAN_POINT('Ctrl Pts',(17.2398314509524,-0.153353235375788,
120.447807567348));
#56254=CARTESIAN_POINT('Ctrl Pts',(17.4080575955601,-0.657352082285856,
120.480043619757));
#56255=CARTESIAN_POINT('Ctrl Pts',(17.7689006127485,-1.05024513051325,120.512408315922));
#56256=CARTESIAN_POINT('Ctrl Pts',(18.2607097297302,-1.26233444597482,120.544902716827));
#56257=CARTESIAN_POINT('Ctrl Pts',(18.7984052352737,-1.25502080659343,120.577527795704));
#56258=CARTESIAN_POINT('Ctrl Pts',(19.2881848794747,-1.0278144553583,120.610284437319));
#56259=CARTESIAN_POINT('Ctrl Pts',(19.6438781749597,-0.61873033468329,120.643173436616));
#56260=CARTESIAN_POINT('Ctrl Pts',(19.8020987090859,-0.0979461688159152,
120.676195498978));
#56261=CARTESIAN_POINT('Ctrl Pts',(19.7335320823132,0.444227716269205,120.709351239055));
#56262=CARTESIAN_POINT('Ctrl Pts',(19.4483480211883,0.912997875362089,120.742641182014));
#56263=CARTESIAN_POINT('Ctrl Pts',(18.9947430992497,1.22566304840365,120.776065760162));
#56264=CARTESIAN_POINT('Ctrl Pts',(18.4508057834443,1.32618611440986,120.809625317582));
#56265=CARTESIAN_POINT('Ctrl Pts',(17.9110852264692,1.19525527808251,120.843320100399));
#56266=CARTESIAN_POINT('Ctrl Pts',(17.4701505494149,0.853917314146234,120.877150274951));
#56267=CARTESIAN_POINT('Ctrl Pts',(17.2060388865232,0.360310149126953,120.911115893666));
#56268=CARTESIAN_POINT('Ctrl Pts',(17.1664153816519,-0.200398871563149,
120.945216959522));
#56269=CARTESIAN_POINT('Ctrl Pts',(17.3116264220795,-0.597882955951257,
120.970894211169));
#56270=CARTESIAN_POINT('Ctrl Pts',(17.4713230749973,-0.824292723162997,
120.988054644643));
#56271=CARTESIAN_POINT('Ctrl Pts',(17.5930295495418,-0.963403094471689,
120.999506127854));
#56272=CARTESIAN_POINT('Ctrl Pts',(17.8429222056168,-1.17180944522949,121.019575839724));
#56273=CARTESIAN_POINT('Ctrl Pts',(18.2831358555107,-1.3472696457857,121.048331046648));
#56274=CARTESIAN_POINT('Ctrl Pts',(18.8536622082132,-1.32345121615729,121.082971735828));
#56275=CARTESIAN_POINT('Ctrl Pts',(19.3666123501032,-1.06776818445665,121.11774633767));
#56276=CARTESIAN_POINT('Ctrl Pts',(19.7318189194698,-0.623135744515387,
121.152654299799));
#56277=CARTESIAN_POINT('Ctrl Pts',(19.8841229814082,-0.0660261383455702,
121.187694946127));
#56278=CARTESIAN_POINT('Ctrl Pts',(19.7952691811095,0.506861240356869,121.22286752838));
#56279=CARTESIAN_POINT('Ctrl Pts',(19.4789909654556,0.995298037449156,121.258171199464));
#56280=CARTESIAN_POINT('Ctrl Pts',(18.9889997447394,1.31312136899922,121.293605027892));
#56281=CARTESIAN_POINT('Ctrl Pts',(18.4098258930854,1.40341469896206,121.329167991327));
#56282=CARTESIAN_POINT('Ctrl Pts',(17.8422514541543,1.2487159173822,121.364858980876));
#56283=CARTESIAN_POINT('Ctrl Pts',(17.3857498366357,0.874358654879244,121.400676801254));
#56284=CARTESIAN_POINT('Ctrl Pts',(17.1210452069084,0.344343613450397,121.436620170121));
#56285=CARTESIAN_POINT('Ctrl Pts',(17.0958251015548,-0.249607404749667,
121.472687721701));
#56286=CARTESIAN_POINT('Ctrl Pts',(17.3161507636215,-0.803935931388206,
121.508878001574));
#56287=CARTESIAN_POINT('Ctrl Pts',(17.7451068582081,-1.22131693446959,121.545189480257));
#56288=CARTESIAN_POINT('Ctrl Pts',(18.3089795239874,-1.42776624833079,121.581620531396));
#56289=CARTESIAN_POINT('Ctrl Pts',(18.9099344796403,-1.38575758159487,121.618169476059));
#56290=CARTESIAN_POINT('Ctrl Pts',(19.443003408243,-1.10105588624391,121.654834501032));
#56291=CARTESIAN_POINT('Ctrl Pts',(19.814447080578,-0.621956720707161,121.691613814933));
#56292=CARTESIAN_POINT('Ctrl Pts',(19.9582412943487,-0.0311460741792062,
121.728505359742));
#56293=CARTESIAN_POINT('Ctrl Pts',(19.8478423707596,0.568675584892993,121.765507307081));
#56294=CARTESIAN_POINT('Ctrl Pts',(19.5010738542693,1.07254435780881,121.802617407826));
#56295=CARTESIAN_POINT('Ctrl Pts',(18.9772465487843,1.39174398963045,121.839833580231));
#56296=CARTESIAN_POINT('Ctrl Pts',(18.3670349923433,1.46935809393124,121.877153590267));
#56297=CARTESIAN_POINT('Ctrl Pts',(17.7767415245785,1.29047771303663,121.91457510912));
#56298=CARTESIAN_POINT('Ctrl Pts',(17.3097639110163,0.88502066898406,121.952095792454));
#56299=CARTESIAN_POINT('Ctrl Pts',(17.0484530789278,0.322744770605088,121.98971320241));
#56300=CARTESIAN_POINT('Ctrl Pts',(17.0395741793232,-0.29877511550778,122.027424807101));
#56301=CARTESIAN_POINT('Ctrl Pts',(17.2859276060077,-0.871100232399064,
122.065228088574));
#56302=CARTESIAN_POINT('Ctrl Pts',(17.7456411246251,-1.29387701195727,122.103120366714));
#56303=CARTESIAN_POINT('Ctrl Pts',(18.3392916665445,-1.49245955151488,122.141098983942));
#56304=CARTESIAN_POINT('Ctrl Pts',(18.9636467540723,-1.43110986029732,122.179161195417));
#56305=CARTESIAN_POINT('Ctrl Pts',(19.5096427527803,-1.11943132446743,122.217304158637));
#56306=CARTESIAN_POINT('Ctrl Pts',(19.8814701962045,-0.610888906864692,
122.255525076564));
#56307=CARTESIAN_POINT('Ctrl Pts',(20.0134084028596,0.00638374819795061,
122.293820960483));
#56308=CARTESIAN_POINT('Ctrl Pts',(19.8814680357448,0.624863883396621,122.332188933733));
#56309=CARTESIAN_POINT('Ctrl Pts',(19.5077372244298,1.13643840843378,122.370625859871));
#56310=CARTESIAN_POINT('Ctrl Pts',(18.9567207702999,1.45127557085421,122.409128868261));
#56311=CARTESIAN_POINT('Ctrl Pts',(18.3241217337611,1.51368240153528,122.447694658652));
#56312=CARTESIAN_POINT('Ctrl Pts',(17.7202826349282,1.31196813537611,122.486320211507));
#56313=CARTESIAN_POINT('Ctrl Pts',(17.2508103246174,0.880536550537675,122.525002285958));
#56314=CARTESIAN_POINT('Ctrl Pts',(16.9981604164449,0.294249197224712,122.563737660687));
#56315=CARTESIAN_POINT('Ctrl Pts',(17.0060423714049,-0.274042958784632,
122.598213625129));
#56316=CARTESIAN_POINT('Ctrl Pts',(17.1818706810392,-0.73303144472968,122.628410343682));
#56317=CARTESIAN_POINT('Ctrl Pts',(17.5191721715142,-1.18310393837461,122.662947355674));
#56318=CARTESIAN_POINT('Ctrl Pts',(18.1531350042187,-1.53390972067408,122.706165522702));
#56319=CARTESIAN_POINT('Ctrl Pts',(19.0227874461394,-1.48519217492529,122.758094642985));
#56320=CARTESIAN_POINT('Ctrl Pts',(19.7338192740336,-0.980774656373063,
122.810082875595));
#56321=CARTESIAN_POINT('Ctrl Pts',(20.067922277282,-0.174626022127283,122.862122158172));
#56322=CARTESIAN_POINT('Ctrl Pts',(19.921708544036,0.68662933685667,122.914204231648));
#56323=CARTESIAN_POINT('Ctrl Pts',(19.4364076102001,1.22943043838242,122.957634782588));
#56324=CARTESIAN_POINT('Ctrl Pts',(18.9192757117743,1.45961435937841,122.992392354061));
#56325=CARTESIAN_POINT('Ctrl Pts',(18.5146998498917,1.51727349960696,123.017500336371));
#56326=CARTESIAN_POINT('Ctrl Pts',(18.1254479581993,1.46800683442712,123.041646590114));
#56327=CARTESIAN_POINT('Ctrl Pts',(17.65765089863,1.28524666288511,123.072557499479));
#56328=CARTESIAN_POINT('Ctrl Pts',(17.1864413110902,0.84817385210292,123.111201426539));
#56329=CARTESIAN_POINT('Ctrl Pts',(16.9818560590682,0.238917012125818,123.149847159061));
#56330=CARTESIAN_POINT('Ctrl Pts',(17.0077477842283,-0.262729802221198,
123.180762273051));
#56331=CARTESIAN_POINT('Ctrl Pts',(17.1549558342261,-0.742832495303323,
123.211674984775));
#56332=CARTESIAN_POINT('Ctrl Pts',(17.5555345576308,-1.24539323375308,123.250310351106));
#56333=CARTESIAN_POINT('Ctrl Pts',(18.2066766855254,-1.51951236558385,123.292795159863));
#56334=CARTESIAN_POINT('Ctrl Pts',(18.8397001520098,-1.49532848220801,123.331402485356));
#56335=CARTESIAN_POINT('Ctrl Pts',(19.361933038917,-1.2676766648096,123.36613474992));
#56336=CARTESIAN_POINT('Ctrl Pts',(19.7646594303858,-0.864798752237798,
123.400850262946));
#56337=CARTESIAN_POINT('Ctrl Pts',(19.992247479715,-0.343129638214644,123.435546682762));
#56338=CARTESIAN_POINT('Ctrl Pts',(20.0134975784261,0.225403110709894,123.470221342828));
#56339=CARTESIAN_POINT('Ctrl Pts',(19.8256820027275,0.761912608646907,123.504872214536));
#56340=CARTESIAN_POINT('Ctrl Pts',(19.516918297423,1.12076930887003,123.533725575818));
#56341=CARTESIAN_POINT('Ctrl Pts',(19.2041810039955,1.32499554631978,123.556794181975));
#56342=CARTESIAN_POINT('Ctrl Pts',(18.8020588760868,1.49233095074489,123.583695662073));
#56343=CARTESIAN_POINT('Ctrl Pts',(18.1960164011262,1.52254678614699,123.620174599657));
#56344=CARTESIAN_POINT('Ctrl Pts',(17.6216673694243,1.24564088295246,123.658522649907));
#56345=CARTESIAN_POINT('Ctrl Pts',(17.2833151529131,0.880111521286915,123.689167672577));
#56346=CARTESIAN_POINT('Ctrl Pts',(17.1050831264071,0.552606139546885,123.712134313292));
#56347=CARTESIAN_POINT('Ctrl Pts',(16.9816547923198,0.0706959663075114,
123.742732173804));
#56348=CARTESIAN_POINT('Ctrl Pts',(17.0529092044043,-0.496279877167484,
123.777112906262));
#56349=CARTESIAN_POINT('Ctrl Pts',(17.3864957981709,-1.02604026133052,123.815255128178));
#56350=CARTESIAN_POINT('Ctrl Pts',(17.857593613417,-1.37397111071324,123.850964243175));
#56351=CARTESIAN_POINT('Ctrl Pts',(18.4515962038669,-1.51829287387834,123.888044644597));
#56352=CARTESIAN_POINT('Ctrl Pts',(19.0746522170704,-1.40326627781162,123.926485479005));
#56353=CARTESIAN_POINT('Ctrl Pts',(19.5520449521414,-1.07433327180886,123.961659739466));
#56354=CARTESIAN_POINT('Ctrl Pts',(19.7870135179904,-0.729922634281818,
123.987199138138));
#56355=CARTESIAN_POINT('Ctrl Pts',(19.9172825726675,-0.412389600249223,
124.008461419526));
#56356=CARTESIAN_POINT('Ctrl Pts',(19.9813821346012,-0.0901260863987032,
124.028642265937));
#56357=CARTESIAN_POINT('Ctrl Pts',(19.9464919895927,0.322871316840072,124.054100150558));
#56358=CARTESIAN_POINT('Ctrl Pts',(19.7988560610193,0.709540527634926,124.079522689038));
#56359=CARTESIAN_POINT('Ctrl Pts',(19.5502809158787,1.03976970882056,124.104909666808));
#56360=CARTESIAN_POINT('Ctrl Pts',(19.2205019215012,1.28789198571529,124.130259814538));
#56361=CARTESIAN_POINT('Ctrl Pts',(18.8675304954949,1.42261786918923,124.153463104108));
#56362=CARTESIAN_POINT('Ctrl Pts',(18.5284830739033,1.46304402439271,124.174529127565));
#56363=CARTESIAN_POINT('Ctrl Pts',(18.1207874834896,1.4260614944801,124.199779233887));
#56364=CARTESIAN_POINT('Ctrl Pts',(17.6438940253866,1.2206283929953,124.231286143554));
#56365=CARTESIAN_POINT('Ctrl Pts',(17.2233006573008,0.762755887841534,124.269003086711));
#56366=CARTESIAN_POINT('Ctrl Pts',(17.0268753162689,0.174604680404742,124.306625880741));
#56367=CARTESIAN_POINT('Ctrl Pts',(17.0876702801681,-0.440949978759675,
124.344152137287));
#56368=CARTESIAN_POINT('Ctrl Pts',(17.3937696919832,-0.976537539345891,
124.381579352596));
#56369=CARTESIAN_POINT('Ctrl Pts',(17.8905867113653,-1.33941486357803,124.41890518565));
#56370=CARTESIAN_POINT('Ctrl Pts',(18.4906153716989,-1.46735186134762,124.456127313473));
#56371=CARTESIAN_POINT('Ctrl Pts',(19.0888593629504,-1.33941777641846,124.493243511411));
#56372=CARTESIAN_POINT('Ctrl Pts',(19.5812312587733,-0.97933823951139,124.530251612046));
#56373=CARTESIAN_POINT('Ctrl Pts',(19.8826841702414,-0.45113379238791,124.567149528264));
#56374=CARTESIAN_POINT('Ctrl Pts',(19.9419184246875,0.15228968271957,124.603935243626));
#56375=CARTESIAN_POINT('Ctrl Pts',(19.7501149544944,0.72549274055214,124.640606820178));
#56376=CARTESIAN_POINT('Ctrl Pts',(19.3422099788232,1.16895227798287,124.677162396834));
#56377=CARTESIAN_POINT('Ctrl Pts',(18.7905344628525,1.4063573661534,124.713600191806));
#56378=CARTESIAN_POINT('Ctrl Pts',(18.1919768114847,1.39775285517752,124.749918502117));
#56379=CARTESIAN_POINT('Ctrl Pts',(17.650949463827,1.14625964667207,124.786115706138));
#56380=CARTESIAN_POINT('Ctrl Pts',(17.2611574231578,0.697245715919318,124.822190264427));
#56381=CARTESIAN_POINT('Ctrl Pts',(17.0893550841156,0.130141700592976,124.858140721292));
#56382=CARTESIAN_POINT('Ctrl Pts',(17.1639091103876,-0.45562104348777,124.893965705161));
#56383=CARTESIAN_POINT('Ctrl Pts',(17.4701273616986,-0.958058662722596,
124.929663929076));
#56384=CARTESIAN_POINT('Ctrl Pts',(17.9531200725725,-1.29040433417455,124.965234192037));
#56385=CARTESIAN_POINT('Ctrl Pts',(18.5276405431088,-1.39610073357796,125.000675380104));
#56386=CARTESIAN_POINT('Ctrl Pts',(19.0931401580165,-1.25842381920182,125.035986467183));
#56387=CARTESIAN_POINT('Ctrl Pts',(19.5513770476802,-0.903101174061878,
125.071166515444));
#56388=CARTESIAN_POINT('Ctrl Pts',(19.8234925261704,-0.393520928653388,
125.106214675531));
#56389=CARTESIAN_POINT('Ctrl Pts',(19.863585446952,0.18057846519377,125.141130187601));
#56390=CARTESIAN_POINT('Ctrl Pts',(19.6664477552688,0.718918428921209,125.175912381995));
#56391=CARTESIAN_POINT('Ctrl Pts',(19.2681597354425,1.12820343239091,125.210560679702));
#56392=CARTESIAN_POINT('Ctrl Pts',(18.7394968083553,1.33829386724977,125.245074592494));
#56393=CARTESIAN_POINT('Ctrl Pts',(18.1733515600056,1.31422440666254,125.279453723019));
#56394=CARTESIAN_POINT('Ctrl Pts',(17.6684072336029,1.06200918227394,125.313697765461));
#56395=CARTESIAN_POINT('Ctrl Pts',(17.3119333434095,0.62727345561428,125.347806505814));
#56396=CARTESIAN_POINT('Ctrl Pts',(17.164703194465,0.0870075502303987,125.381779821996));
#56397=CARTESIAN_POINT('Ctrl Pts',(17.2506394082675,-0.464067284867245,
125.415617683646));
#56398=CARTESIAN_POINT('Ctrl Pts',(17.5529500312885,-0.93010635281992,125.449320152153));
#56399=CARTESIAN_POINT('Ctrl Pts',(18.0173742562096,-1.23080998259887,125.482887380882));
#56400=CARTESIAN_POINT('Ctrl Pts',(18.5619148970354,-1.31525442806852,125.516319615136));
#56401=CARTESIAN_POINT('Ctrl Pts',(19.0913123481237,-1.17050448618906,125.54961719185));
#56402=CARTESIAN_POINT('Ctrl Pts',(19.5137054329361,-0.823554001177106,
125.582780539051));
#56403=CARTESIAN_POINT('Ctrl Pts',(19.7565657136191,-0.336311890299757,
125.615810175785));
#56404=CARTESIAN_POINT('Ctrl Pts',(19.7791421686803,0.205437475860851,125.64870671201));
#56405=CARTESIAN_POINT('Ctrl Pts',(19.5792831503527,0.707131271594729,125.681470848156));
#56406=CARTESIAN_POINT('Ctrl Pts',(19.1934974783569,1.08192650056308,125.714103374504));
#56407=CARTESIAN_POINT('Ctrl Pts',(18.6903000531182,1.26572269937722,125.74660517022));
#56408=CARTESIAN_POINT('Ctrl Pts',(18.1580528586921,1.22811231780654,125.778977203127));
#56409=CARTESIAN_POINT('Ctrl Pts',(17.6894582924859,0.977390643756032,125.811220529498));
#56410=CARTESIAN_POINT('Ctrl Pts',(17.3654249182296,0.55880467658169,125.843336292948));
#56411=CARTESIAN_POINT('Ctrl Pts',(17.2411113552341,0.0464007134562138,
125.875325723779));
#56412=CARTESIAN_POINT('Ctrl Pts',(17.3365525714722,-0.470062155704644,
125.907190137343));
#56413=CARTESIAN_POINT('Ctrl Pts',(17.6334582774054,-0.900821679431447,
125.938930933878));
#56414=CARTESIAN_POINT('Ctrl Pts',(18.078689306533,-1.17169762162142,125.970549597961));
#56415=CARTESIAN_POINT('Ctrl Pts',(18.593754716555,-1.23684923441498,126.002047697117));
#56416=CARTESIAN_POINT('Ctrl Pts',(19.0886338471913,-1.0865147767173,126.033426880753));
#56417=CARTESIAN_POINT('Ctrl Pts',(19.4774918201155,-0.748430497103195,
126.064688878174));
#56418=CARTESIAN_POINT('Ctrl Pts',(19.6935481589647,-0.282732209663939,
126.095835498253));
#56419=CARTESIAN_POINT('Ctrl Pts',(19.7005261381603,0.228725868558277,126.126868628752));
#56420=CARTESIAN_POINT('Ctrl Pts',(19.4987238371462,0.696739517761545,126.157790234506));
#56421=CARTESIAN_POINT('Ctrl Pts',(19.1246955649095,1.04029099805458,126.188602356125));
#56422=CARTESIAN_POINT('Ctrl Pts',(18.6446468213007,1.20055180571536,126.219307107577));
#56423=CARTESIAN_POINT('Ctrl Pts',(18.1427337757278,1.15093580581614,126.24990667576));
#56424=CARTESIAN_POINT('Ctrl Pts',(17.7063324713574,0.901488522300449,126.280403319565));
#56425=CARTESIAN_POINT('Ctrl Pts',(17.4108529526162,0.496892712939118,126.310799367952));
#56426=CARTESIAN_POINT('Ctrl Pts',(17.3067328954843,0.0084812245335301,
126.34109721811));
#56427=CARTESIAN_POINT('Ctrl Pts',(17.4108490145204,-0.47831756693869,126.371299332964));
#56428=CARTESIAN_POINT('Ctrl Pts',(17.7038045321021,-0.878895943230857,
126.401408240409));
#56429=CARTESIAN_POINT('Ctrl Pts',(18.1335240920449,-1.12414442958507,126.431426532286));
#56430=CARTESIAN_POINT('Ctrl Pts',(18.6244919535479,-1.17234924842773,126.461356862258));
#56431=CARTESIAN_POINT('Ctrl Pts',(19.0909970917821,-1.01626672882518,126.491201943604));
#56432=CARTESIAN_POINT('Ctrl Pts',(19.4520665620905,-0.684179402726174,
126.520964546554));
#56433=CARTESIAN_POINT('Ctrl Pts',(19.6454906893739,-0.234786668051046,
126.550647497157));
#56434=CARTESIAN_POINT('Ctrl Pts',(19.6385159835268,0.253149219888882,126.580253676135));
#56435=CARTESIAN_POINT('Ctrl Pts',(19.4333722711128,0.694578566817253,126.609786017081));
#56436=CARTESIAN_POINT('Ctrl Pts',(19.0667063558325,1.01295613554844,126.639247502871));
#56437=CARTESIAN_POINT('Ctrl Pts',(18.6030514946211,1.1534838541102,126.668641164986));
#56438=CARTESIAN_POINT('Ctrl Pts',(18.1234957510667,1.09251755167767,126.697970077986));
#56439=CARTESIAN_POINT('Ctrl Pts',(17.7115308462464,0.841530068193854,126.727237365886));
#56440=CARTESIAN_POINT('Ctrl Pts',(17.4385535098235,0.444964463531077,126.756446186453));
#56441=CARTESIAN_POINT('Ctrl Pts',(17.3515170588706,-0.0276122872710075,
126.785599752877));
#56442=CARTESIAN_POINT('Ctrl Pts',(17.4648884689082,-0.493692017961726,
126.814701285522));
#56443=CARTESIAN_POINT('Ctrl Pts',(17.7582364067503,-0.872180645238306,
126.843754094616));
#56444=CARTESIAN_POINT('Ctrl Pts',(18.1799399597792,-1.09750112430032,126.872761421116));
#56445=CARTESIAN_POINT('Ctrl Pts',(18.6561791423461,-1.13087232076486,126.901726730967));
#56446=CARTESIAN_POINT('Ctrl Pts',(19.1039589342991,-0.967064360638307,
126.930653153623));
#56447=CARTESIAN_POINT('Ctrl Pts',(19.3883902256841,-0.690354148280827,
126.954729317772));
#56448=CARTESIAN_POINT('Ctrl Pts',(19.5332457227074,-0.414056911611768,
126.973973920849));
#56449=CARTESIAN_POINT('Ctrl Pts',(19.6177437769726,-0.113905111418309,
126.993208932229));
#56450=CARTESIAN_POINT('Ctrl Pts',(19.6011038359952,0.281732384417546,127.017234385341));
#56451=CARTESIAN_POINT('Ctrl Pts',(19.3890514321733,0.706565085330299,127.04604027079));
#56452=CARTESIAN_POINT('Ctrl Pts',(19.0223011451343,1.00751421476368,127.074824428941));
#56453=CARTESIAN_POINT('Ctrl Pts',(18.5648792017946,1.13234542273552,127.103590628698));
#56454=CARTESIAN_POINT('Ctrl Pts',(18.0966155583551,1.05950100369092,127.13234222422));
#56455=CARTESIAN_POINT('Ctrl Pts',(17.6990872091144,0.801854248777839,127.161082806753));
#56456=CARTESIAN_POINT('Ctrl Pts',(17.4415305074347,0.404417889894389,127.18981585486));
#56457=CARTESIAN_POINT('Ctrl Pts',(17.3687695530042,-0.0634870235218906,
127.218544916761));
#56458=CARTESIAN_POINT('Ctrl Pts',(17.4934609062107,-0.520295799873725,
127.247273508358));
#56459=CARTESIAN_POINT('Ctrl Pts',(17.7938846953223,-0.886376575644098,
127.276005163098));
#56460=CARTESIAN_POINT('Ctrl Pts',(18.2177247634987,-1.0978765550393,127.304743403475));
#56461=CARTESIAN_POINT('Ctrl Pts',(18.6911508939668,-1.11782834790528,127.333491753923));
#56462=CARTESIAN_POINT('Ctrl Pts',(19.1316465689169,-0.942594483611371,
127.362253727978));
#56463=CARTESIAN_POINT('Ctrl Pts',(19.4623516371648,-0.602527764442204,
127.391032833955));
#56464=CARTESIAN_POINT('Ctrl Pts',(19.6254375334004,-0.156728820867022,
127.419832557726));
#56465=CARTESIAN_POINT('Ctrl Pts',(19.5921943171502,0.317197263638082,127.448656399276));
#56466=CARTESIAN_POINT('Ctrl Pts',(19.368068361135,0.736614311055538,127.477507771776));
#56467=CARTESIAN_POINT('Ctrl Pts',(18.9917822982762,1.02822677014049,127.506390229474));
#56468=CARTESIAN_POINT('Ctrl Pts',(18.5286553795516,1.1408523543525,127.535306988223));
#56469=CARTESIAN_POINT('Ctrl Pts',(18.0593071007243,1.05438854513454,127.564261845145));
#56470=CARTESIAN_POINT('Ctrl Pts',(17.665645179454,0.78337931240486,127.593257348673));
#56471=CARTESIAN_POINT('Ctrl Pts',(17.4166255106301,0.374596672588247,127.622298651964));
#56472=CARTESIAN_POINT('Ctrl Pts',(17.356168808789,-0.10102697056375,127.651385319048));
#56473=CARTESIAN_POINT('Ctrl Pts',(17.4955452283241,-0.560666528004949,
127.680527574784));
#56474=CARTESIAN_POINT('Ctrl Pts',(17.8109503297906,-0.923997881438208,
127.709717292561));
#56475=CARTESIAN_POINT('Ctrl Pts',(18.2483725221223,-1.12713601481138,127.738975362331));
#56476=CARTESIAN_POINT('Ctrl Pts',(18.7311725427411,-1.13411043401417,127.768275574607));
#56477=CARTESIAN_POINT('Ctrl Pts',(19.1762783013378,-0.942422457862223,
127.797675015527));
#56478=CARTESIAN_POINT('Ctrl Pts',(19.5046484170361,-0.585761601815651,
127.827081897376));
#56479=CARTESIAN_POINT('Ctrl Pts',(19.6582495271737,-0.123680562238502,
127.85662756148));
#56480=CARTESIAN_POINT('Ctrl Pts',(19.6201095104048,0.280620801278878,127.881304584504));
#56481=CARTESIAN_POINT('Ctrl Pts',(19.4907597078714,0.572725205601487,127.900977353949));
#56482=CARTESIAN_POINT('Ctrl Pts',(19.3483928135265,0.768967247407983,127.915853796736));
#56483=CARTESIAN_POINT('Ctrl Pts',(19.1686762334047,0.931517072832566,127.930784609013));
#56484=CARTESIAN_POINT('Ctrl Pts',(18.9634686971736,1.051701521621,127.945656286825));
#56485=CARTESIAN_POINT('Ctrl Pts',(18.7395400780403,1.12529086281877,127.960455609962));
#56486=CARTESIAN_POINT('Ctrl Pts',(18.5767277357217,1.14299969027711,127.970442080495));
#56487=CARTESIAN_POINT('Ctrl Pts',(18.491314532458,1.14371857755274,127.975498274504));
#56488=CARTESIAN_POINT('Ctrl Pts',(18.319436888783,1.28857481063387,112.710548866174));
#56489=CARTESIAN_POINT('Ctrl Pts',(18.2367206542011,1.27796812314438,112.715656822746));
#56490=CARTESIAN_POINT('Ctrl Pts',(18.1122722696272,1.24996406005619,112.723602742685));
#56491=CARTESIAN_POINT('Ctrl Pts',(17.9105741471188,1.1715572059241,112.7372275449));
#56492=CARTESIAN_POINT('Ctrl Pts',(17.7147016928909,1.05680544825268,112.75142581384));
#56493=CARTESIAN_POINT('Ctrl Pts',(17.5092914781924,0.870936460786282,112.768496063499));
#56494=CARTESIAN_POINT('Ctrl Pts',(17.3452643787265,0.645338607702756,112.785608543142));
#56495=CARTESIAN_POINT('Ctrl Pts',(17.1949694671818,0.305633664533222,112.808486356608));
#56496=CARTESIAN_POINT('Ctrl Pts',(17.1504041586296,-0.163958059400556,
112.8371493128));
#56497=CARTESIAN_POINT('Ctrl Pts',(17.3295581344551,-0.704127606930189,
112.871679546659));
#56498=CARTESIAN_POINT('Ctrl Pts',(17.7163063911852,-1.12497913550319,112.906352649458));
#56499=CARTESIAN_POINT('Ctrl Pts',(18.2431925961433,-1.35205912276461,112.941152109412));
#56500=CARTESIAN_POINT('Ctrl Pts',(18.8187741112765,-1.34427642838518,112.976089285723));
#56501=CARTESIAN_POINT('Ctrl Pts',(19.3432395618757,-1.10098396627254,113.011156346434));
#56502=CARTESIAN_POINT('Ctrl Pts',(19.7238494382154,-0.663159822701633,
113.046357078694));
#56503=CARTESIAN_POINT('Ctrl Pts',(19.8931314314799,-0.105956319615994,
113.08168722595));
#56504=CARTESIAN_POINT('Ctrl Pts',(19.8197719071333,0.473908286429459,113.117148366555));
#56505=CARTESIAN_POINT('Ctrl Pts',(19.514861434432,0.975046989864885,113.152737815001));
#56506=CARTESIAN_POINT('Ctrl Pts',(19.0301258646803,1.30913564752012,113.188455340763));
#56507=CARTESIAN_POINT('Ctrl Pts',(18.4491549165285,1.416472562517,113.224299311997));
#56508=CARTESIAN_POINT('Ctrl Pts',(17.8730091730699,1.27666467315962,113.260268611474));
#56509=CARTESIAN_POINT('Ctrl Pts',(17.4026034483492,0.912474225359778,113.296361769111));
#56510=CARTESIAN_POINT('Ctrl Pts',(17.1210280345443,0.386131812194797,113.332577359437));
#56511=CARTESIAN_POINT('Ctrl Pts',(17.0788544181136,-0.211299879373549,
113.368913814958));
#56512=CARTESIAN_POINT('Ctrl Pts',(17.2850565553758,-0.775695991436841,
113.405369493798));
#56513=CARTESIAN_POINT('Ctrl Pts',(17.705146965038,-1.20803167965084,113.441942712263));
#56514=CARTESIAN_POINT('Ctrl Pts',(18.2669652505624,-1.43177932086286,113.478631613973));
#56515=CARTESIAN_POINT('Ctrl Pts',(18.8730309513044,-1.40645905314605,113.51543444437));
#56516=CARTESIAN_POINT('Ctrl Pts',(19.4175618056869,-1.13497091574588,113.55234907248));
#56517=CARTESIAN_POINT('Ctrl Pts',(19.8048480383929,-0.663350581086933,
113.589373656825));
#56518=CARTESIAN_POINT('Ctrl Pts',(19.966197057422,-0.0729778537808475,
113.626505971993));
#56519=CARTESIAN_POINT('Ctrl Pts',(19.8720657245217,0.533549954628291,113.663743893195));
#56520=CARTESIAN_POINT('Ctrl Pts',(19.5374817640394,1.0501311842453,113.701085198819));
#56521=CARTESIAN_POINT('Ctrl Pts',(19.0196808505253,1.38594482959087,113.738527490934));
#56522=CARTESIAN_POINT('Ctrl Pts',(18.5101754020758,1.46526119175664,113.769811704289));
#56523=CARTESIAN_POINT('Ctrl Pts',(18.1090240872925,1.39960741569811,113.794887075397));
#56524=CARTESIAN_POINT('Ctrl Pts',(17.729655069815,1.25220225914757,113.819994103033));
#56525=CARTESIAN_POINT('Ctrl Pts',(17.3289300722954,0.923586877948104,113.851436567131));
#56526=CARTESIAN_POINT('Ctrl Pts',(17.0504721252432,0.365805609893722,113.889258509496));
#56527=CARTESIAN_POINT('Ctrl Pts',(17.0240290762783,-0.258477757917008,
113.927168961164));
#56528=CARTESIAN_POINT('Ctrl Pts',(17.2554238425403,-0.840447617959809,
113.965165177094));
#56529=CARTESIAN_POINT('Ctrl Pts',(17.7053131011304,-1.27808626113464,114.003244380208));
#56530=CARTESIAN_POINT('Ctrl Pts',(18.2959641544648,-1.49425702735341,114.041403784502));
#56531=CARTESIAN_POINT('Ctrl Pts',(18.9246622805112,-1.4502272181577,114.079640512388));
#56532=CARTESIAN_POINT('Ctrl Pts',(19.4816239236303,-1.15267110135651,114.117951609114));
#56533=CARTESIAN_POINT('Ctrl Pts',(19.8691907107327,-0.652639427392253,
114.156334167846));
#56534=CARTESIAN_POINT('Ctrl Pts',(20.0189810591327,-0.03683256961316,114.194785080069));
#56535=CARTESIAN_POINT('Ctrl Pts',(19.9039833865991,0.587522999416328,114.2333013558));
#56536=CARTESIAN_POINT('Ctrl Pts',(19.5434230734537,1.11127572106957,114.271879839515));
#56537=CARTESIAN_POINT('Ctrl Pts',(18.9995399107886,1.44259279852258,114.310517384521));
#56538=CARTESIAN_POINT('Ctrl Pts',(18.3668596633944,1.52297273199859,114.349210799966));
#56539=CARTESIAN_POINT('Ctrl Pts',(17.7556977562459,1.33767203016567,114.387956849117));
#56540=CARTESIAN_POINT('Ctrl Pts',(17.272914349715,0.918370107647551,114.426752263094));
#56541=CARTESIAN_POINT('Ctrl Pts',(17.0031861863323,0.337753138207008,114.46559374694));
#56542=CARTESIAN_POINT('Ctrl Pts',(16.9941242219495,-0.303088855509916,
114.504477951706));
#56543=CARTESIAN_POINT('Ctrl Pts',(17.2478715429229,-0.892350566926149,
114.543401543985));
#56544=CARTESIAN_POINT('Ctrl Pts',(17.720592505509,-1.32694200600498,114.582361077963));
#56545=CARTESIAN_POINT('Ctrl Pts',(18.3301332049521,-1.53077558802408,114.621353247865));
#56546=CARTESIAN_POINT('Ctrl Pts',(18.8635057740616,-1.47820468577621,114.653870882415));
#56547=CARTESIAN_POINT('Ctrl Pts',(19.2496685905278,-1.30821665552171,114.679897931973));
#56548=CARTESIAN_POINT('Ctrl Pts',(19.5923918636366,-1.06191387672613,114.705932982827));
#56549=CARTESIAN_POINT('Ctrl Pts',(19.9091081456583,-0.628734129737697,
114.738490494062));
#56550=CARTESIAN_POINT('Ctrl Pts',(20.0436482399265,0.00136013336455928,
114.777578396996));
#56551=CARTESIAN_POINT('Ctrl Pts',(19.9090928165798,0.631655323772199,114.816681421648));
#56552=CARTESIAN_POINT('Ctrl Pts',(19.5286868815429,1.1521949790643,114.855796201813));
#56553=CARTESIAN_POINT('Ctrl Pts',(18.9687372623033,1.47200625927751,114.894919129408));
#56554=CARTESIAN_POINT('Ctrl Pts',(18.3269247722238,1.53523233022917,114.934046750203));
#56555=CARTESIAN_POINT('Ctrl Pts',(17.7152334288248,1.33076841613399,114.973175454517));
#56556=CARTESIAN_POINT('Ctrl Pts',(17.2404725580255,0.894349558877001,115.012301840373));
#56557=CARTESIAN_POINT('Ctrl Pts',(16.9853446354984,0.302108848816737,115.051422158546));
#56558=CARTESIAN_POINT('Ctrl Pts',(16.9934993376988,-0.27079628228924,115.086187634404));
#56559=CARTESIAN_POINT('Ctrl Pts',(17.1704122775008,-0.733300276011371,
115.116598560424));
#56560=CARTESIAN_POINT('Ctrl Pts',(17.3615831320585,-0.98758491633179,115.136144037193));
#56561=CARTESIAN_POINT('Ctrl Pts',(17.5154254407977,-1.13081668225498,115.149171118788));
#56562=CARTESIAN_POINT('Ctrl Pts',(17.5970581795022,-1.19692836165928,115.155684477762));
#56563=CARTESIAN_POINT('Ctrl Pts',(17.6831967780099,-1.25709479715135,115.162197134421));
#56564=CARTESIAN_POINT('Ctrl Pts',(17.8633620834074,-1.36516570458449,115.175222025971));
#56565=CARTESIAN_POINT('Ctrl Pts',(18.1604819038664,-1.47854845945174,115.194753812955));
#56566=CARTESIAN_POINT('Ctrl Pts',(18.582786890695,-1.51417568969967,115.220787745291));
#56567=CARTESIAN_POINT('Ctrl Pts',(18.9983836416472,-1.43149328105734,115.246809679889));
#56568=CARTESIAN_POINT('Ctrl Pts',(19.374473528925,-1.23714016652633,115.27282057109));
#56569=CARTESIAN_POINT('Ctrl Pts',(19.6822598946567,-0.946311359030486,
115.298817689622));
#56570=CARTESIAN_POINT('Ctrl Pts',(19.8967480474023,-0.582015055171165,
115.324801432878));
#56571=CARTESIAN_POINT('Ctrl Pts',(20.0386193688326,-0.0359715504243672,
115.359425895719));
#56572=CARTESIAN_POINT('Ctrl Pts',(19.941536265269,0.535299448860012,115.394018366274));
#56573=CARTESIAN_POINT('Ctrl Pts',(19.6668198938765,0.944384240575756,115.424255526598));
#56574=CARTESIAN_POINT('Ctrl Pts',(19.4671125145751,1.13894829771433,115.44152396901));
#56575=CARTESIAN_POINT('Ctrl Pts',(19.2416596715355,1.3035791132569,115.458786271138));
#56576=CARTESIAN_POINT('Ctrl Pts',(19.0175256336374,1.40399060754221,115.473882214218));
#56577=CARTESIAN_POINT('Ctrl Pts',(18.8150509122225,1.45460978349152,115.486814484407));
#56578=CARTESIAN_POINT('Ctrl Pts',(18.7124011810244,1.4728082953005,115.493279478184));
#56579=CARTESIAN_POINT('Ctrl Pts',(18.6259805295674,1.48196183269604,115.498665769091));
#56580=CARTESIAN_POINT('Ctrl Pts',(18.5565983881251,1.48554743331276,115.502974301951));
#56581=CARTESIAN_POINT('Ctrl Pts',(18.275006635137,1.49093350233563,115.520445423601));
#56582=CARTESIAN_POINT('Ctrl Pts',(17.7643189677256,1.36044159259875,115.552131188091));
#56583=CARTESIAN_POINT('Ctrl Pts',(17.3297966145357,0.957318076594017,115.587783846009));
#56584=CARTESIAN_POINT('Ctrl Pts',(17.1366050542202,0.593850002954031,115.613220643608));
#56585=CARTESIAN_POINT('Ctrl Pts',(17.0708721336454,0.399095376421441,115.625931295202));
#56586=CARTESIAN_POINT('Ctrl Pts',(17.0385717481457,0.238286256682236,115.636095006768));
#56587=CARTESIAN_POINT('Ctrl Pts',(17.0000053948983,-0.0873641069959773,
115.656416799589));
#56588=CARTESIAN_POINT('Ctrl Pts',(17.0954817402936,-0.627463061463085,
115.689403138097));
#56589=CARTESIAN_POINT('Ctrl Pts',(17.5683032047114,-1.2202390337612,115.734986014693));
#56590=CARTESIAN_POINT('Ctrl Pts',(18.2073749791171,-1.48915585063008,115.776682365231));
#56591=CARTESIAN_POINT('Ctrl Pts',(18.827714255502,-1.46536270236631,115.81451460932));
#56592=CARTESIAN_POINT('Ctrl Pts',(19.3387291215206,-1.24252555435953,115.848504801486));
#56593=CARTESIAN_POINT('Ctrl Pts',(19.7323390465761,-0.84870905484788,115.882433969696));
#56594=CARTESIAN_POINT('Ctrl Pts',(19.917317868452,-0.424382854990528,115.910656120296));
#56595=CARTESIAN_POINT('Ctrl Pts',(19.9647758151583,-0.0623666971425709,
115.933200950891));
#56596=CARTESIAN_POINT('Ctrl Pts',(19.9494967945027,0.210678396553568,115.950093741532));
#56597=CARTESIAN_POINT('Ctrl Pts',(19.8946537689314,0.431722595099945,115.964156440341));
#56598=CARTESIAN_POINT('Ctrl Pts',(19.8267524040723,0.599946781165768,115.975398400255));
#56599=CARTESIAN_POINT('Ctrl Pts',(19.7020401592803,0.841706463647344,115.992253058882));
#56600=CARTESIAN_POINT('Ctrl Pts',(19.4317853790293,1.15561589179994,116.017502153899));
#56601=CARTESIAN_POINT('Ctrl Pts',(18.9444409086331,1.41307035879397,116.051097502054));
#56602=CARTESIAN_POINT('Ctrl Pts',(18.3979015457458,1.47453073660614,116.084620132269));
#56603=CARTESIAN_POINT('Ctrl Pts',(18.0004069582635,1.36793073631313,116.1097063674));
#56604=CARTESIAN_POINT('Ctrl Pts',(17.763366663899,1.23962198295239,116.126406802779));
#56605=CARTESIAN_POINT('Ctrl Pts',(17.6140480708204,1.1398854968943,116.137534246267));
#56606=CARTESIAN_POINT('Ctrl Pts',(17.3790836560323,0.929981622126309,116.156989690435));
#56607=CARTESIAN_POINT('Ctrl Pts',(17.2215832331742,0.679602546844773,116.175024509631));
#56608=CARTESIAN_POINT('Ctrl Pts',(17.1450352066694,0.469669982396278,116.188878617737));
#56609=CARTESIAN_POINT('Ctrl Pts',(17.1249441446997,0.405767087289566,116.193033537477));
#56610=CARTESIAN_POINT('Ctrl Pts',(17.1079301441042,0.340970796669862,116.197187251518));
#56611=CARTESIAN_POINT('Ctrl Pts',(17.0939473695056,0.275494153967272,116.201339691278));
#56612=CARTESIAN_POINT('Ctrl Pts',(17.0830227708597,0.209443458520346,116.205490910608));
#56613=CARTESIAN_POINT('Ctrl Pts',(17.0726655652121,0.120824547382831,116.211024197657));
#56614=CARTESIAN_POINT('Ctrl Pts',(17.0610173800014,-0.124379540531134,
116.226234061721));
#56615=CARTESIAN_POINT('Ctrl Pts',(17.1369245229291,-0.5249310381429,116.251084258337));
#56616=CARTESIAN_POINT('Ctrl Pts',(17.4255200195769,-0.984001270082908,
116.284135719174));
#56617=CARTESIAN_POINT('Ctrl Pts',(17.8607605682645,-1.30506353431624,116.317102617813));
#56618=CARTESIAN_POINT('Ctrl Pts',(18.3818866043649,-1.44455243472689,116.349983938512));
#56619=CARTESIAN_POINT('Ctrl Pts',(18.916470350186,-1.38418902476214,116.382777928971));
#56620=CARTESIAN_POINT('Ctrl Pts',(19.3908578736671,-1.13333494037052,116.415483428707));
#56621=CARTESIAN_POINT('Ctrl Pts',(19.662129258784,-0.817824110576332,116.440850810503));
#56622=CARTESIAN_POINT('Ctrl Pts',(19.7921004518703,-0.556121431420674,
116.458936888485));
#56623=CARTESIAN_POINT('Ctrl Pts',(19.8690655500124,-0.335782443963777,
116.473391787428));
#56624=CARTESIAN_POINT('Ctrl Pts',(19.9308282800101,0.0701141608640084,
116.498652513443));
#56625=CARTESIAN_POINT('Ctrl Pts',(19.7975561020439,0.653379656102897,116.534635638022));
#56626=CARTESIAN_POINT('Ctrl Pts',(19.3238121146665,1.18955843336623,116.577647401962));
#56627=CARTESIAN_POINT('Ctrl Pts',(18.6542573597491,1.43288587092525,116.620488268205));
#56628=CARTESIAN_POINT('Ctrl Pts',(17.9525424324882,1.32679118729713,116.663155847902));
#56629=CARTESIAN_POINT('Ctrl Pts',(17.4716228570456,0.961996366384522,116.699450989897));
#56630=CARTESIAN_POINT('Ctrl Pts',(17.2242845453766,0.540894020126181,116.729451046567));
#56631=CARTESIAN_POINT('Ctrl Pts',(17.0944240343639,0.041457592091441,116.761140226464));
#56632=CARTESIAN_POINT('Ctrl Pts',(17.2055334687691,-0.610901669378824,
116.8006093271));
#56633=CARTESIAN_POINT('Ctrl Pts',(17.7327235525077,-1.19996474577183,116.847741724244));
#56634=CARTESIAN_POINT('Ctrl Pts',(18.4886274023919,-1.41711476065944,116.894641370113));
#56635=CARTESIAN_POINT('Ctrl Pts',(19.2403913761961,-1.19999329817096,116.941306241231));
#56636=CARTESIAN_POINT('Ctrl Pts',(19.7589583230562,-0.618976305235332,
116.987734609023));
#56637=CARTESIAN_POINT('Ctrl Pts',(19.866303857657,0.0173456111094613,117.026226666982));
#56638=CARTESIAN_POINT('Ctrl Pts',(19.7405351404932,0.500732911611066,117.05690073817));
#56639=CARTESIAN_POINT('Ctrl Pts',(19.5511427517233,0.822664799957136,117.079846452937));
#56640=CARTESIAN_POINT('Ctrl Pts',(19.2800271222083,1.07822752115069,117.102732140544));
#56641=CARTESIAN_POINT('Ctrl Pts',(18.840099008821,1.30647550082486,117.13316636068));
#56642=CARTESIAN_POINT('Ctrl Pts',(18.2057864265544,1.34185814168128,117.171058787474));
#56643=CARTESIAN_POINT('Ctrl Pts',(17.5421074842011,0.974328602971076,117.216288928054));
#56644=CARTESIAN_POINT('Ctrl Pts',(17.1777038347398,0.313792671011465,117.261278280207));
#56645=CARTESIAN_POINT('Ctrl Pts',(17.2203225463522,-0.435464225919962,
117.306027156934));
#56646=CARTESIAN_POINT('Ctrl Pts',(17.652724667813,-1.04386133116569,117.350536141848));
#56647=CARTESIAN_POINT('Ctrl Pts',(18.3388239098277,-1.32745573236693,117.39480611765));
#56648=CARTESIAN_POINT('Ctrl Pts',(19.0667149711576,-1.20320856043253,117.438838249758));
#56649=CARTESIAN_POINT('Ctrl Pts',(19.6139786084161,-0.713397943859653,
117.482633994782));
#56650=CARTESIAN_POINT('Ctrl Pts',(19.8156811381899,-0.0112791664943189,
117.526195091984));
#56651=CARTESIAN_POINT('Ctrl Pts',(19.6140022601783,0.686784214414896,117.569523562413));
#56652=CARTESIAN_POINT('Ctrl Pts',(19.0747275941947,1.16798331893147,117.612621710931));
#56653=CARTESIAN_POINT('Ctrl Pts',(18.3658643708616,1.28788138840837,117.655492120034));
#56654=CARTESIAN_POINT('Ctrl Pts',(17.7053431257873,1.01371279747136,117.69813764302));
#56655=CARTESIAN_POINT('Ctrl Pts',(17.2940790801678,0.433188982502828,117.740561406275));
#56656=CARTESIAN_POINT('Ctrl Pts',(17.2549003691858,-0.273508324804743,
117.782766808914));
#56657=CARTESIAN_POINT('Ctrl Pts',(17.5959737510632,-0.889574255288579,
117.824757505323));
#56658=CARTESIAN_POINT('Ctrl Pts',(18.2094168755739,-1.22806570874149,117.866537413039));
#56659=CARTESIAN_POINT('Ctrl Pts',(18.9055013390443,-1.18847566627298,117.908110699435));
#56660=CARTESIAN_POINT('Ctrl Pts',(19.4709991235593,-0.786645501256251,
117.949481800211));
#56661=CARTESIAN_POINT('Ctrl Pts',(19.7349121554302,-0.148494032303403,
117.990655350317));
#56662=CARTESIAN_POINT('Ctrl Pts',(19.6384296844279,0.41595364745626,118.024806143826));
#56663=CARTESIAN_POINT('Ctrl Pts',(19.3912822005401,0.783910465160815,118.052032979065));
#56664=CARTESIAN_POINT('Ctrl Pts',(19.0539455301924,1.06997780245999,118.079198326187));
#56665=CARTESIAN_POINT('Ctrl Pts',(18.5086041618223,1.22692728472169,118.113040992046));
#56666=CARTESIAN_POINT('Ctrl Pts',(17.8570681242743,1.03871258992206,118.153475788182));
#56667=CARTESIAN_POINT('Ctrl Pts',(17.4074661243136,0.535028360348281,118.193739748399));
#56668=CARTESIAN_POINT('Ctrl Pts',(17.295184410072,-0.12802353903353,118.233838994046));
#56669=CARTESIAN_POINT('Ctrl Pts',(17.5518536435643,-0.746678185841251,
118.273779650817));
#56670=CARTESIAN_POINT('Ctrl Pts',(18.09623557474,-1.13252353284961,118.313568149567));
#56671=CARTESIAN_POINT('Ctrl Pts',(18.7600131800788,-1.16944565236424,118.353211038631));
#56672=CARTESIAN_POINT('Ctrl Pts',(19.3396804878931,-0.848740522078599,
118.392715097256));
#56673=CARTESIAN_POINT('Ctrl Pts',(19.6587833880623,-0.270665095166121,
118.432087186673));
#56674=CARTESIAN_POINT('Ctrl Pts',(19.6216208701028,0.386364157140476,118.471334476116));
#56675=CARTESIAN_POINT('Ctrl Pts',(19.2416211971827,0.921545428620454,118.510464030869));
#56676=CARTESIAN_POINT('Ctrl Pts',(18.7378784200697,1.12977499085113,118.542980260458));
#56677=CARTESIAN_POINT('Ctrl Pts',(18.3152260681784,1.11706291748731,118.56894164302));
#56678=CARTESIAN_POINT('Ctrl Pts',(18.013631331558,1.02122659296196,118.588388203893));
#56679=CARTESIAN_POINT('Ctrl Pts',(17.7507020897944,0.845342251383026,118.607810663731));
#56680=CARTESIAN_POINT('Ctrl Pts',(17.5469576086983,0.604112404067775,118.62721063314));
#56681=CARTESIAN_POINT('Ctrl Pts',(17.418115189222,0.316066123273868,118.646588439489));
#56682=CARTESIAN_POINT('Ctrl Pts',(17.3740914074908,0.00406156609269027,
118.665945648007));
#56683=CARTESIAN_POINT('Ctrl Pts',(17.418105330468,-0.307731076500601,118.68528270408));
#56684=CARTESIAN_POINT('Ctrl Pts',(17.5252095909573,-0.546868258948941,
118.701381492349));
#56685=CARTESIAN_POINT('Ctrl Pts',(17.6479384162453,-0.714878730507821,
118.714251085885));
#56686=CARTESIAN_POINT('Ctrl Pts',(17.7929243818857,-0.863723509943578,
118.727115583167));
#56687=CARTESIAN_POINT('Ctrl Pts',(18.0972164483336,-1.06793358028532,118.74961267773));
#56688=CARTESIAN_POINT('Ctrl Pts',(18.6276378637832,-1.15815365828481,118.781712261723));
#56689=CARTESIAN_POINT('Ctrl Pts',(19.2238118827329,-0.91106020954,118.820176086249));
#56690=CARTESIAN_POINT('Ctrl Pts',(19.5340790733567,-0.473298914368946,
118.852189669591));
#56691=CARTESIAN_POINT('Ctrl Pts',(19.6045033571726,-0.115359348913955,
118.874582530202));
#56692=CARTESIAN_POINT('Ctrl Pts',(19.6017475647411,0.0911640829913528,
118.88737350014));
#56693=CARTESIAN_POINT('Ctrl Pts',(19.5700196370974,0.29559108219492,118.900162446911));
#56694=CARTESIAN_POINT('Ctrl Pts',(19.4770780543413,0.538342967989427,118.916143236651));
#56695=CARTESIAN_POINT('Ctrl Pts',(19.2273588011135,0.871529045839169,118.941704029868));
#56696=CARTESIAN_POINT('Ctrl Pts',(18.7588367207674,1.13058490335296,118.973640684375));
#56697=CARTESIAN_POINT('Ctrl Pts',(18.1172887995021,1.09452313569986,119.011950738852));
#56698=CARTESIAN_POINT('Ctrl Pts',(17.593388380079,0.722780783019972,119.050254797413));
#56699=CARTESIAN_POINT('Ctrl Pts',(17.3886684004257,0.228286678671025,119.082177254148));
#56700=CARTESIAN_POINT('Ctrl Pts',(17.4011923319186,-0.187547154371747,
119.107720239302));
#56701=CARTESIAN_POINT('Ctrl Pts',(17.479741012236,-0.43518291567232,119.123688362763));
#56702=CARTESIAN_POINT('Ctrl Pts',(17.5695979738663,-0.592074644579124,
119.134867535548));
#56703=CARTESIAN_POINT('Ctrl Pts',(17.6297289359476,-0.675697287840335,
119.1412564699));
#56704=CARTESIAN_POINT('Ctrl Pts',(17.6957161316275,-0.754921963867992,
119.147645877012));
#56705=CARTESIAN_POINT('Ctrl Pts',(17.7882499830905,-0.84489988474299,119.155633946795));
#56706=CARTESIAN_POINT('Ctrl Pts',(17.9550205699679,-0.966828303763707,
119.168415926821));
#56707=CARTESIAN_POINT('Ctrl Pts',(18.1925073400234,-1.07312652027406,119.184398568056));
#56708=CARTESIAN_POINT('Ctrl Pts',(18.5018237176362,-1.11680179614521,119.203585076302));
#56709=CARTESIAN_POINT('Ctrl Pts',(18.8112727437243,-1.07312083019676,119.222781017226));
#56710=CARTESIAN_POINT('Ctrl Pts',(19.0966922989243,-0.945425429896232,
119.241986576724));
#56711=CARTESIAN_POINT('Ctrl Pts',(19.3357397025375,-0.743574694906012,
119.261203548649));
#56712=CARTESIAN_POINT('Ctrl Pts',(19.5096763702265,-0.483296157484075,
119.280432047793));
#56713=CARTESIAN_POINT('Ctrl Pts',(19.604829263032,-0.184805761734769,119.299674358162));
#56714=CARTESIAN_POINT('Ctrl Pts',(19.6136282032755,0.128548869667553,119.318929822438));
#56715=CARTESIAN_POINT('Ctrl Pts',(19.5483562428395,0.381754662526241,119.334989622353));
#56716=CARTESIAN_POINT('Ctrl Pts',(19.4555027014667,0.567586338753027,119.347844753828));
#56717=CARTESIAN_POINT('Ctrl Pts',(19.3083285466207,0.781707993580481,119.363921119013));
#56718=CARTESIAN_POINT('Ctrl Pts',(19.0213883195784,1.0173014385066,119.386447876364));
#56719=CARTESIAN_POINT('Ctrl Pts',(18.5601806816014,1.14326482672377,119.415452744608));
#56720=CARTESIAN_POINT('Ctrl Pts',(18.0870469004768,1.06976794361554,119.444502870166));
#56721=CARTESIAN_POINT('Ctrl Pts',(17.6845073765261,0.809000046868888,119.473601565479));
#56722=CARTESIAN_POINT('Ctrl Pts',(17.4231181242213,0.405838898540841,119.502752060927));
#56723=CARTESIAN_POINT('Ctrl Pts',(17.3490598832109,-0.0697983875198877,
119.531957712525));
#56724=CARTESIAN_POINT('Ctrl Pts',(17.4759534440631,-0.535171725229621,
119.561221496182));
#56725=CARTESIAN_POINT('Ctrl Pts',(17.7314548399343,-0.846550437506931,
119.58565944407));
#56726=CARTESIAN_POINT('Ctrl Pts',(17.999207559364,-1.0170868157945,119.605241751292));
#56727=CARTESIAN_POINT('Ctrl Pts',(18.2967905723551,-1.12863703662001,119.624846422395));
#56728=CARTESIAN_POINT('Ctrl Pts',(18.701022235534,-1.14581433888424,119.649394327387));
#56729=CARTESIAN_POINT('Ctrl Pts',(19.1533010528138,-0.965969567310355,
119.678922596865));
#56730=CARTESIAN_POINT('Ctrl Pts',(19.4935242230618,-0.616264784255005,
119.708524488639));
#56731=CARTESIAN_POINT('Ctrl Pts',(19.6616806751607,-0.15688731828813,119.738203011753));
#56732=CARTESIAN_POINT('Ctrl Pts',(19.6274500840142,0.332402173060607,119.767961008938));
#56733=CARTESIAN_POINT('Ctrl Pts',(19.3957290628344,0.766238455283539,119.797801335606));
#56734=CARTESIAN_POINT('Ctrl Pts',(19.0059018782433,1.06845895995986,119.827726746298));
#56735=CARTESIAN_POINT('Ctrl Pts',(18.5252515327408,1.18543071772727,119.857739979944));
#56736=CARTESIAN_POINT('Ctrl Pts',(18.037234743022,1.09564506473,119.887843657137));
#56737=CARTESIAN_POINT('Ctrl Pts',(17.6956019306827,0.860470084296629,119.913007640695));
#56738=CARTESIAN_POINT('Ctrl Pts',(17.4972936032911,0.600305772965447,119.93318661626));
#56739=CARTESIAN_POINT('Ctrl Pts',(17.3569038509229,0.304279815543778,119.953397785618));
#56740=CARTESIAN_POINT('Ctrl Pts',(17.3041660284991,-0.109796929925252,
119.978723169803));
#56741=CARTESIAN_POINT('Ctrl Pts',(17.4498994353956,-0.59078091166106,120.009214030095));
#56742=CARTESIAN_POINT('Ctrl Pts',(17.7804655429487,-0.971566966837065,
120.039807705564));
#56743=CARTESIAN_POINT('Ctrl Pts',(18.2393086861239,-1.18486584665598,120.07050641441));
#56744=CARTESIAN_POINT('Ctrl Pts',(18.7470163437987,-1.1921729938516,120.101312384752));
#56745=CARTESIAN_POINT('Ctrl Pts',(19.215087635489,-0.990765643040621,120.132227714623));
#56746=CARTESIAN_POINT('Ctrl Pts',(19.5613155231427,-0.614392148089554,
120.163254460057));
#56747=CARTESIAN_POINT('Ctrl Pts',(19.7242152497417,-0.127659401515012,
120.194394583265));
#56748=CARTESIAN_POINT('Ctrl Pts',(19.6739207775415,0.385049104109546,120.225649979257));
#56749=CARTESIAN_POINT('Ctrl Pts',(19.4176458057697,0.834175476321175,120.257022460356));
#56750=CARTESIAN_POINT('Ctrl Pts',(18.998699632526,1.14061462596676,120.288513762116));
#56751=CARTESIAN_POINT('Ctrl Pts',(18.4891879156563,1.24962833189955,120.320125537776));
#56752=CARTESIAN_POINT('Ctrl Pts',(17.9776202690671,1.14060959036587,120.351859359126));
#56753=CARTESIAN_POINT('Ctrl Pts',(17.5535525982464,0.830952823101709,120.383716714854));
#56754=CARTESIAN_POINT('Ctrl Pts',(17.2919248389954,0.373308289212946,120.415699010712));
#56755=CARTESIAN_POINT('Ctrl Pts',(17.2398314509524,-0.153353235375788,
120.447807567348));
#56756=CARTESIAN_POINT('Ctrl Pts',(17.4080575955601,-0.657352082285856,
120.480043619757));
#56757=CARTESIAN_POINT('Ctrl Pts',(17.7689006127485,-1.05024513051325,120.512408315922));
#56758=CARTESIAN_POINT('Ctrl Pts',(18.2607097297302,-1.26233444597482,120.544902716827));
#56759=CARTESIAN_POINT('Ctrl Pts',(18.7984052352737,-1.25502080659343,120.577527795704));
#56760=CARTESIAN_POINT('Ctrl Pts',(19.2881848794747,-1.0278144553583,120.610284437319));
#56761=CARTESIAN_POINT('Ctrl Pts',(19.6438781749597,-0.61873033468329,120.643173436616));
#56762=CARTESIAN_POINT('Ctrl Pts',(19.8020987090859,-0.0979461688159152,
120.676195498978));
#56763=CARTESIAN_POINT('Ctrl Pts',(19.7335320823132,0.444227716269205,120.709351239055));
#56764=CARTESIAN_POINT('Ctrl Pts',(19.4483480211883,0.912997875362089,120.742641182014));
#56765=CARTESIAN_POINT('Ctrl Pts',(18.9947430992497,1.22566304840365,120.776065760162));
#56766=CARTESIAN_POINT('Ctrl Pts',(18.4508057834443,1.32618611440986,120.809625317582));
#56767=CARTESIAN_POINT('Ctrl Pts',(17.9110852264692,1.19525527808251,120.843320100399));
#56768=CARTESIAN_POINT('Ctrl Pts',(17.4701505494149,0.853917314146234,120.877150274951));
#56769=CARTESIAN_POINT('Ctrl Pts',(17.2060388865232,0.360310149126953,120.911115893666));
#56770=CARTESIAN_POINT('Ctrl Pts',(17.1664153816519,-0.200398871563149,
120.945216959522));
#56771=CARTESIAN_POINT('Ctrl Pts',(17.3116264220795,-0.597882955951257,
120.970894211169));
#56772=CARTESIAN_POINT('Ctrl Pts',(17.4713230749973,-0.824292723162997,
120.988054644643));
#56773=CARTESIAN_POINT('Ctrl Pts',(17.5930295495418,-0.963403094471689,
120.999506127854));
#56774=CARTESIAN_POINT('Ctrl Pts',(17.8429222056168,-1.17180944522949,121.019575839724));
#56775=CARTESIAN_POINT('Ctrl Pts',(18.2831358555107,-1.3472696457857,121.048331046648));
#56776=CARTESIAN_POINT('Ctrl Pts',(18.8536622082132,-1.32345121615729,121.082971735828));
#56777=CARTESIAN_POINT('Ctrl Pts',(19.3666123501032,-1.06776818445665,121.11774633767));
#56778=CARTESIAN_POINT('Ctrl Pts',(19.7318189194698,-0.623135744515387,
121.152654299799));
#56779=CARTESIAN_POINT('Ctrl Pts',(19.8841229814082,-0.0660261383455702,
121.187694946127));
#56780=CARTESIAN_POINT('Ctrl Pts',(19.7952691811095,0.506861240356869,121.22286752838));
#56781=CARTESIAN_POINT('Ctrl Pts',(19.4789909654556,0.995298037449156,121.258171199464));
#56782=CARTESIAN_POINT('Ctrl Pts',(18.9889997447394,1.31312136899922,121.293605027892));
#56783=CARTESIAN_POINT('Ctrl Pts',(18.4098258930854,1.40341469896206,121.329167991327));
#56784=CARTESIAN_POINT('Ctrl Pts',(17.8422514541543,1.2487159173822,121.364858980876));
#56785=CARTESIAN_POINT('Ctrl Pts',(17.3857498366357,0.874358654879244,121.400676801254));
#56786=CARTESIAN_POINT('Ctrl Pts',(17.1210452069084,0.344343613450397,121.436620170121));
#56787=CARTESIAN_POINT('Ctrl Pts',(17.0958251015548,-0.249607404749667,
121.472687721701));
#56788=CARTESIAN_POINT('Ctrl Pts',(17.3161507636215,-0.803935931388206,
121.508878001574));
#56789=CARTESIAN_POINT('Ctrl Pts',(17.7451068582081,-1.22131693446959,121.545189480257));
#56790=CARTESIAN_POINT('Ctrl Pts',(18.3089795239874,-1.42776624833079,121.581620531396));
#56791=CARTESIAN_POINT('Ctrl Pts',(18.9099344796403,-1.38575758159487,121.618169476059));
#56792=CARTESIAN_POINT('Ctrl Pts',(19.443003408243,-1.10105588624391,121.654834501032));
#56793=CARTESIAN_POINT('Ctrl Pts',(19.814447080578,-0.621956720707161,121.691613814933));
#56794=CARTESIAN_POINT('Ctrl Pts',(19.9582412943487,-0.0311460741792062,
121.728505359742));
#56795=CARTESIAN_POINT('Ctrl Pts',(19.8478423707596,0.568675584892993,121.765507307081));
#56796=CARTESIAN_POINT('Ctrl Pts',(19.5010738542693,1.07254435780881,121.802617407826));
#56797=CARTESIAN_POINT('Ctrl Pts',(18.9772465487843,1.39174398963045,121.839833580231));
#56798=CARTESIAN_POINT('Ctrl Pts',(18.3670349923433,1.46935809393124,121.877153590267));
#56799=CARTESIAN_POINT('Ctrl Pts',(17.7767415245785,1.29047771303663,121.91457510912));
#56800=CARTESIAN_POINT('Ctrl Pts',(17.3097639110163,0.88502066898406,121.952095792454));
#56801=CARTESIAN_POINT('Ctrl Pts',(17.0484530789278,0.322744770605088,121.98971320241));
#56802=CARTESIAN_POINT('Ctrl Pts',(17.0395741793232,-0.29877511550778,122.027424807101));
#56803=CARTESIAN_POINT('Ctrl Pts',(17.2859276060077,-0.871100232399064,
122.065228088574));
#56804=CARTESIAN_POINT('Ctrl Pts',(17.7456411246251,-1.29387701195727,122.103120366714));
#56805=CARTESIAN_POINT('Ctrl Pts',(18.3392916665445,-1.49245955151488,122.141098983942));
#56806=CARTESIAN_POINT('Ctrl Pts',(18.9636467540723,-1.43110986029732,122.179161195417));
#56807=CARTESIAN_POINT('Ctrl Pts',(19.5096427527803,-1.11943132446743,122.217304158637));
#56808=CARTESIAN_POINT('Ctrl Pts',(19.8814701962045,-0.610888906864692,
122.255525076564));
#56809=CARTESIAN_POINT('Ctrl Pts',(20.0134084028596,0.00638374819795061,
122.293820960483));
#56810=CARTESIAN_POINT('Ctrl Pts',(19.8814680357448,0.624863883396621,122.332188933733));
#56811=CARTESIAN_POINT('Ctrl Pts',(19.5077372244298,1.13643840843378,122.370625859871));
#56812=CARTESIAN_POINT('Ctrl Pts',(18.9567207702999,1.45127557085421,122.409128868261));
#56813=CARTESIAN_POINT('Ctrl Pts',(18.3241217337611,1.51368240153528,122.447694658652));
#56814=CARTESIAN_POINT('Ctrl Pts',(17.7202826349282,1.31196813537611,122.486320211507));
#56815=CARTESIAN_POINT('Ctrl Pts',(17.2508103246174,0.880536550537675,122.525002285958));
#56816=CARTESIAN_POINT('Ctrl Pts',(16.9981604164449,0.294249197224712,122.563737660687));
#56817=CARTESIAN_POINT('Ctrl Pts',(17.0060423714049,-0.274042958784632,
122.598213625129));
#56818=CARTESIAN_POINT('Ctrl Pts',(17.1818706810392,-0.73303144472968,122.628410343682));
#56819=CARTESIAN_POINT('Ctrl Pts',(17.5191721715142,-1.18310393837461,122.662947355674));
#56820=CARTESIAN_POINT('Ctrl Pts',(18.1531350042187,-1.53390972067408,122.706165522702));
#56821=CARTESIAN_POINT('Ctrl Pts',(19.0227874461394,-1.48519217492529,122.758094642985));
#56822=CARTESIAN_POINT('Ctrl Pts',(19.7338192740336,-0.980774656373063,
122.810082875595));
#56823=CARTESIAN_POINT('Ctrl Pts',(20.067922277282,-0.174626022127283,122.862122158172));
#56824=CARTESIAN_POINT('Ctrl Pts',(19.921708544036,0.68662933685667,122.914204231648));
#56825=CARTESIAN_POINT('Ctrl Pts',(19.4364076102001,1.22943043838242,122.957634782588));
#56826=CARTESIAN_POINT('Ctrl Pts',(18.9192757117743,1.45961435937841,122.992392354061));
#56827=CARTESIAN_POINT('Ctrl Pts',(18.5146998498917,1.51727349960696,123.017500336371));
#56828=CARTESIAN_POINT('Ctrl Pts',(18.1254479581993,1.46800683442712,123.041646590114));
#56829=CARTESIAN_POINT('Ctrl Pts',(17.65765089863,1.28524666288511,123.072557499479));
#56830=CARTESIAN_POINT('Ctrl Pts',(17.1864413110902,0.84817385210292,123.111201426539));
#56831=CARTESIAN_POINT('Ctrl Pts',(16.9818560590682,0.238917012125818,123.149847159061));
#56832=CARTESIAN_POINT('Ctrl Pts',(17.0077477842283,-0.262729802221198,
123.180762273051));
#56833=CARTESIAN_POINT('Ctrl Pts',(17.1549558342261,-0.742832495303323,
123.211674984775));
#56834=CARTESIAN_POINT('Ctrl Pts',(17.5555345576308,-1.24539323375308,123.250310351106));
#56835=CARTESIAN_POINT('Ctrl Pts',(18.2066766855254,-1.51951236558385,123.292795159863));
#56836=CARTESIAN_POINT('Ctrl Pts',(18.8397001520098,-1.49532848220801,123.331402485356));
#56837=CARTESIAN_POINT('Ctrl Pts',(19.361933038917,-1.2676766648096,123.36613474992));
#56838=CARTESIAN_POINT('Ctrl Pts',(19.7646594303858,-0.864798752237798,
123.400850262946));
#56839=CARTESIAN_POINT('Ctrl Pts',(19.992247479715,-0.343129638214644,123.435546682762));
#56840=CARTESIAN_POINT('Ctrl Pts',(20.0134975784261,0.225403110709894,123.470221342828));
#56841=CARTESIAN_POINT('Ctrl Pts',(19.8256820027275,0.761912608646907,123.504872214536));
#56842=CARTESIAN_POINT('Ctrl Pts',(19.516918297423,1.12076930887003,123.533725575818));
#56843=CARTESIAN_POINT('Ctrl Pts',(19.2041810039955,1.32499554631978,123.556794181975));
#56844=CARTESIAN_POINT('Ctrl Pts',(18.8020588760868,1.49233095074489,123.583695662073));
#56845=CARTESIAN_POINT('Ctrl Pts',(18.1960164011262,1.52254678614699,123.620174599657));
#56846=CARTESIAN_POINT('Ctrl Pts',(17.6216673694243,1.24564088295246,123.658522649907));
#56847=CARTESIAN_POINT('Ctrl Pts',(17.2833151529131,0.880111521286915,123.689167672577));
#56848=CARTESIAN_POINT('Ctrl Pts',(17.1050831264071,0.552606139546885,123.712134313292));
#56849=CARTESIAN_POINT('Ctrl Pts',(16.9816547923198,0.0706959663075114,
123.742732173804));
#56850=CARTESIAN_POINT('Ctrl Pts',(17.0529092044043,-0.496279877167484,
123.777112906262));
#56851=CARTESIAN_POINT('Ctrl Pts',(17.3864957981709,-1.02604026133052,123.815255128178));
#56852=CARTESIAN_POINT('Ctrl Pts',(17.857593613417,-1.37397111071324,123.850964243175));
#56853=CARTESIAN_POINT('Ctrl Pts',(18.4515962038669,-1.51829287387834,123.888044644597));
#56854=CARTESIAN_POINT('Ctrl Pts',(19.0746522170704,-1.40326627781162,123.926485479005));
#56855=CARTESIAN_POINT('Ctrl Pts',(19.5520449521414,-1.07433327180886,123.961659739466));
#56856=CARTESIAN_POINT('Ctrl Pts',(19.7870135179904,-0.729922634281818,
123.987199138138));
#56857=CARTESIAN_POINT('Ctrl Pts',(19.9172825726675,-0.412389600249223,
124.008461419526));
#56858=CARTESIAN_POINT('Ctrl Pts',(19.9813821346012,-0.0901260863987032,
124.028642265937));
#56859=CARTESIAN_POINT('Ctrl Pts',(19.9464919895927,0.322871316840072,124.054100150558));
#56860=CARTESIAN_POINT('Ctrl Pts',(19.7988560610193,0.709540527634926,124.079522689038));
#56861=CARTESIAN_POINT('Ctrl Pts',(19.5502809158787,1.03976970882056,124.104909666808));
#56862=CARTESIAN_POINT('Ctrl Pts',(19.2205019215012,1.28789198571529,124.130259814538));
#56863=CARTESIAN_POINT('Ctrl Pts',(18.8675304954949,1.42261786918923,124.153463104108));
#56864=CARTESIAN_POINT('Ctrl Pts',(18.5284830739033,1.46304402439271,124.174529127565));
#56865=CARTESIAN_POINT('Ctrl Pts',(18.1207874834896,1.4260614944801,124.199779233887));
#56866=CARTESIAN_POINT('Ctrl Pts',(17.6438940253866,1.2206283929953,124.231286143554));
#56867=CARTESIAN_POINT('Ctrl Pts',(17.2233006573008,0.762755887841534,124.269003086711));
#56868=CARTESIAN_POINT('Ctrl Pts',(17.0268753162689,0.174604680404742,124.306625880741));
#56869=CARTESIAN_POINT('Ctrl Pts',(17.0876702801681,-0.440949978759675,
124.344152137287));
#56870=CARTESIAN_POINT('Ctrl Pts',(17.3937696919832,-0.976537539345891,
124.381579352596));
#56871=CARTESIAN_POINT('Ctrl Pts',(17.8905867113653,-1.33941486357803,124.41890518565));
#56872=CARTESIAN_POINT('Ctrl Pts',(18.4906153716989,-1.46735186134762,124.456127313473));
#56873=CARTESIAN_POINT('Ctrl Pts',(19.0888593629504,-1.33941777641846,124.493243511411));
#56874=CARTESIAN_POINT('Ctrl Pts',(19.5812312587733,-0.97933823951139,124.530251612046));
#56875=CARTESIAN_POINT('Ctrl Pts',(19.8826841702414,-0.45113379238791,124.567149528264));
#56876=CARTESIAN_POINT('Ctrl Pts',(19.9419184246875,0.15228968271957,124.603935243626));
#56877=CARTESIAN_POINT('Ctrl Pts',(19.7501149544944,0.72549274055214,124.640606820178));
#56878=CARTESIAN_POINT('Ctrl Pts',(19.3422099788232,1.16895227798287,124.677162396834));
#56879=CARTESIAN_POINT('Ctrl Pts',(18.7905344628525,1.4063573661534,124.713600191806));
#56880=CARTESIAN_POINT('Ctrl Pts',(18.1919768114847,1.39775285517752,124.749918502117));
#56881=CARTESIAN_POINT('Ctrl Pts',(17.650949463827,1.14625964667207,124.786115706138));
#56882=CARTESIAN_POINT('Ctrl Pts',(17.2611574231578,0.697245715919318,124.822190264427));
#56883=CARTESIAN_POINT('Ctrl Pts',(17.0893550841156,0.130141700592976,124.858140721292));
#56884=CARTESIAN_POINT('Ctrl Pts',(17.1639091103876,-0.45562104348777,124.893965705161));
#56885=CARTESIAN_POINT('Ctrl Pts',(17.4701273616986,-0.958058662722596,
124.929663929076));
#56886=CARTESIAN_POINT('Ctrl Pts',(17.9531200725725,-1.29040433417455,124.965234192037));
#56887=CARTESIAN_POINT('Ctrl Pts',(18.5276405431088,-1.39610073357796,125.000675380104));
#56888=CARTESIAN_POINT('Ctrl Pts',(19.0931401580165,-1.25842381920182,125.035986467183));
#56889=CARTESIAN_POINT('Ctrl Pts',(19.5513770476802,-0.903101174061878,
125.071166515444));
#56890=CARTESIAN_POINT('Ctrl Pts',(19.8234925261704,-0.393520928653388,
125.106214675531));
#56891=CARTESIAN_POINT('Ctrl Pts',(19.863585446952,0.18057846519377,125.141130187601));
#56892=CARTESIAN_POINT('Ctrl Pts',(19.6664477552688,0.718918428921209,125.175912381995));
#56893=CARTESIAN_POINT('Ctrl Pts',(19.2681597354425,1.12820343239091,125.210560679702));
#56894=CARTESIAN_POINT('Ctrl Pts',(18.7394968083553,1.33829386724977,125.245074592494));
#56895=CARTESIAN_POINT('Ctrl Pts',(18.1733515600056,1.31422440666254,125.279453723019));
#56896=CARTESIAN_POINT('Ctrl Pts',(17.6684072336029,1.06200918227394,125.313697765461));
#56897=CARTESIAN_POINT('Ctrl Pts',(17.3119333434095,0.62727345561428,125.347806505814));
#56898=CARTESIAN_POINT('Ctrl Pts',(17.164703194465,0.0870075502303987,125.381779821996));
#56899=CARTESIAN_POINT('Ctrl Pts',(17.2506394082675,-0.464067284867245,
125.415617683646));
#56900=CARTESIAN_POINT('Ctrl Pts',(17.5529500312885,-0.93010635281992,125.449320152153));
#56901=CARTESIAN_POINT('Ctrl Pts',(18.0173742562096,-1.23080998259887,125.482887380882));
#56902=CARTESIAN_POINT('Ctrl Pts',(18.5619148970354,-1.31525442806852,125.516319615136));
#56903=CARTESIAN_POINT('Ctrl Pts',(19.0913123481237,-1.17050448618906,125.54961719185));
#56904=CARTESIAN_POINT('Ctrl Pts',(19.5137054329361,-0.823554001177106,
125.582780539051));
#56905=CARTESIAN_POINT('Ctrl Pts',(19.7565657136191,-0.336311890299757,
125.615810175785));
#56906=CARTESIAN_POINT('Ctrl Pts',(19.7791421686803,0.205437475860851,125.64870671201));
#56907=CARTESIAN_POINT('Ctrl Pts',(19.5792831503527,0.707131271594729,125.681470848156));
#56908=CARTESIAN_POINT('Ctrl Pts',(19.1934974783569,1.08192650056308,125.714103374504));
#56909=CARTESIAN_POINT('Ctrl Pts',(18.6903000531182,1.26572269937722,125.74660517022));
#56910=CARTESIAN_POINT('Ctrl Pts',(18.1580528586921,1.22811231780654,125.778977203127));
#56911=CARTESIAN_POINT('Ctrl Pts',(17.6894582924859,0.977390643756032,125.811220529498));
#56912=CARTESIAN_POINT('Ctrl Pts',(17.3654249182296,0.55880467658169,125.843336292948));
#56913=CARTESIAN_POINT('Ctrl Pts',(17.2411113552341,0.0464007134562138,
125.875325723779));
#56914=CARTESIAN_POINT('Ctrl Pts',(17.3365525714722,-0.470062155704644,
125.907190137343));
#56915=CARTESIAN_POINT('Ctrl Pts',(17.6334582774054,-0.900821679431447,
125.938930933878));
#56916=CARTESIAN_POINT('Ctrl Pts',(18.078689306533,-1.17169762162142,125.970549597961));
#56917=CARTESIAN_POINT('Ctrl Pts',(18.593754716555,-1.23684923441498,126.002047697117));
#56918=CARTESIAN_POINT('Ctrl Pts',(19.0886338471913,-1.0865147767173,126.033426880753));
#56919=CARTESIAN_POINT('Ctrl Pts',(19.4774918201155,-0.748430497103195,
126.064688878174));
#56920=CARTESIAN_POINT('Ctrl Pts',(19.6935481589647,-0.282732209663939,
126.095835498253));
#56921=CARTESIAN_POINT('Ctrl Pts',(19.7005261381603,0.228725868558277,126.126868628752));
#56922=CARTESIAN_POINT('Ctrl Pts',(19.4987238371462,0.696739517761545,126.157790234506));
#56923=CARTESIAN_POINT('Ctrl Pts',(19.1246955649095,1.04029099805458,126.188602356125));
#56924=CARTESIAN_POINT('Ctrl Pts',(18.6446468213007,1.20055180571536,126.219307107577));
#56925=CARTESIAN_POINT('Ctrl Pts',(18.1427337757278,1.15093580581614,126.24990667576));
#56926=CARTESIAN_POINT('Ctrl Pts',(17.7063324713574,0.901488522300449,126.280403319565));
#56927=CARTESIAN_POINT('Ctrl Pts',(17.4108529526162,0.496892712939118,126.310799367952));
#56928=CARTESIAN_POINT('Ctrl Pts',(17.3067328954843,0.0084812245335301,
126.34109721811));
#56929=CARTESIAN_POINT('Ctrl Pts',(17.4108490145204,-0.47831756693869,126.371299332964));
#56930=CARTESIAN_POINT('Ctrl Pts',(17.7038045321021,-0.878895943230857,
126.401408240409));
#56931=CARTESIAN_POINT('Ctrl Pts',(18.1335240920449,-1.12414442958507,126.431426532286));
#56932=CARTESIAN_POINT('Ctrl Pts',(18.6244919535479,-1.17234924842773,126.461356862258));
#56933=CARTESIAN_POINT('Ctrl Pts',(19.0909970917821,-1.01626672882518,126.491201943604));
#56934=CARTESIAN_POINT('Ctrl Pts',(19.4520665620905,-0.684179402726174,
126.520964546554));
#56935=CARTESIAN_POINT('Ctrl Pts',(19.6454906893739,-0.234786668051046,
126.550647497157));
#56936=CARTESIAN_POINT('Ctrl Pts',(19.6385159835268,0.253149219888882,126.580253676135));
#56937=CARTESIAN_POINT('Ctrl Pts',(19.4333722711128,0.694578566817253,126.609786017081));
#56938=CARTESIAN_POINT('Ctrl Pts',(19.0667063558325,1.01295613554844,126.639247502871));
#56939=CARTESIAN_POINT('Ctrl Pts',(18.6030514946211,1.1534838541102,126.668641164986));
#56940=CARTESIAN_POINT('Ctrl Pts',(18.1234957510667,1.09251755167767,126.697970077986));
#56941=CARTESIAN_POINT('Ctrl Pts',(17.7115308462464,0.841530068193854,126.727237365886));
#56942=CARTESIAN_POINT('Ctrl Pts',(17.4385535098235,0.444964463531077,126.756446186453));
#56943=CARTESIAN_POINT('Ctrl Pts',(17.3515170588706,-0.0276122872710075,
126.785599752877));
#56944=CARTESIAN_POINT('Ctrl Pts',(17.4648884689082,-0.493692017961726,
126.814701285522));
#56945=CARTESIAN_POINT('Ctrl Pts',(17.7582364067503,-0.872180645238306,
126.843754094616));
#56946=CARTESIAN_POINT('Ctrl Pts',(18.1799399597792,-1.09750112430032,126.872761421116));
#56947=CARTESIAN_POINT('Ctrl Pts',(18.6561791423461,-1.13087232076486,126.901726730967));
#56948=CARTESIAN_POINT('Ctrl Pts',(19.1039589342991,-0.967064360638307,
126.930653153623));
#56949=CARTESIAN_POINT('Ctrl Pts',(19.3883902256841,-0.690354148280827,
126.954729317772));
#56950=CARTESIAN_POINT('Ctrl Pts',(19.5332457227074,-0.414056911611768,
126.973973920849));
#56951=CARTESIAN_POINT('Ctrl Pts',(19.6177437769726,-0.113905111418309,
126.993208932229));
#56952=CARTESIAN_POINT('Ctrl Pts',(19.6011038359952,0.281732384417546,127.017234385341));
#56953=CARTESIAN_POINT('Ctrl Pts',(19.3890514321733,0.706565085330299,127.04604027079));
#56954=CARTESIAN_POINT('Ctrl Pts',(19.0223011451343,1.00751421476368,127.074824428941));
#56955=CARTESIAN_POINT('Ctrl Pts',(18.5648792017946,1.13234542273552,127.103590628698));
#56956=CARTESIAN_POINT('Ctrl Pts',(18.0966155583551,1.05950100369092,127.13234222422));
#56957=CARTESIAN_POINT('Ctrl Pts',(17.6990872091144,0.801854248777839,127.161082806753));
#56958=CARTESIAN_POINT('Ctrl Pts',(17.4415305074347,0.404417889894389,127.18981585486));
#56959=CARTESIAN_POINT('Ctrl Pts',(17.3687695530042,-0.0634870235218906,
127.218544916761));
#56960=CARTESIAN_POINT('Ctrl Pts',(17.4934609062107,-0.520295799873725,
127.247273508358));
#56961=CARTESIAN_POINT('Ctrl Pts',(17.7938846953223,-0.886376575644098,
127.276005163098));
#56962=CARTESIAN_POINT('Ctrl Pts',(18.2177247634987,-1.0978765550393,127.304743403475));
#56963=CARTESIAN_POINT('Ctrl Pts',(18.6911508939668,-1.11782834790528,127.333491753923));
#56964=CARTESIAN_POINT('Ctrl Pts',(19.1316465689169,-0.942594483611371,
127.362253727978));
#56965=CARTESIAN_POINT('Ctrl Pts',(19.4623516371648,-0.602527764442204,
127.391032833955));
#56966=CARTESIAN_POINT('Ctrl Pts',(19.6254375334004,-0.156728820867022,
127.419832557726));
#56967=CARTESIAN_POINT('Ctrl Pts',(19.5921943171502,0.317197263638082,127.448656399276));
#56968=CARTESIAN_POINT('Ctrl Pts',(19.368068361135,0.736614311055538,127.477507771776));
#56969=CARTESIAN_POINT('Ctrl Pts',(18.9917822982762,1.02822677014049,127.506390229474));
#56970=CARTESIAN_POINT('Ctrl Pts',(18.5286553795516,1.1408523543525,127.535306988223));
#56971=CARTESIAN_POINT('Ctrl Pts',(18.0593071007243,1.05438854513454,127.564261845145));
#56972=CARTESIAN_POINT('Ctrl Pts',(17.665645179454,0.78337931240486,127.593257348673));
#56973=CARTESIAN_POINT('Ctrl Pts',(17.4166255106301,0.374596672588247,127.622298651964));
#56974=CARTESIAN_POINT('Ctrl Pts',(17.356168808789,-0.10102697056375,127.651385319048));
#56975=CARTESIAN_POINT('Ctrl Pts',(17.4955452283241,-0.560666528004949,
127.680527574784));
#56976=CARTESIAN_POINT('Ctrl Pts',(17.8109503297906,-0.923997881438208,
127.709717292561));
#56977=CARTESIAN_POINT('Ctrl Pts',(18.2483725221223,-1.12713601481138,127.738975362331));
#56978=CARTESIAN_POINT('Ctrl Pts',(18.7311725427411,-1.13411043401417,127.768275574607));
#56979=CARTESIAN_POINT('Ctrl Pts',(19.1762783013378,-0.942422457862223,
127.797675015527));
#56980=CARTESIAN_POINT('Ctrl Pts',(19.5046484170361,-0.585761601815651,
127.827081897376));
#56981=CARTESIAN_POINT('Ctrl Pts',(19.6582495271737,-0.123680562238502,
127.85662756148));
#56982=CARTESIAN_POINT('Ctrl Pts',(19.6201095104048,0.280620801278878,127.881304584504));
#56983=CARTESIAN_POINT('Ctrl Pts',(19.4907597078714,0.572725205601487,127.900977353949));
#56984=CARTESIAN_POINT('Ctrl Pts',(19.3483928135265,0.768967247407983,127.915853796736));
#56985=CARTESIAN_POINT('Ctrl Pts',(19.1686762334047,0.931517072832566,127.930784609013));
#56986=CARTESIAN_POINT('Ctrl Pts',(18.9634686971736,1.051701521621,127.945656286825));
#56987=CARTESIAN_POINT('Ctrl Pts',(18.7934282466761,1.10758167118611,127.956894169607));
#56988=CARTESIAN_POINT('Ctrl Pts',(18.692507014378,1.12612980783387,127.963248051465));
#56989=CARTESIAN_POINT('Ctrl Pts',(18.6702756913488,1.12955277882793,127.964633433995));
#71463=UNCERTAINTY_MEASURE_WITH_UNIT(LENGTH_MEASURE(0.001),#71493,
'DISTANCE_ACCURACY_VALUE',
'Maximum model space distance between geometric entities at asserted c
onnectivities');
#71471=UNCERTAINTY_MEASURE_WITH_UNIT(LENGTH_MEASURE(0.001),#71493,
'DISTANCE_ACCURACY_VALUE',
'Maximum model space distance between geometric entities at asserted c
onnectivities');
#71484=(
GEOMETRIC_REPRESENTATION_CONTEXT(3)
GLOBAL_UNCERTAINTY_ASSIGNED_CONTEXT((#71463))
GLOBAL_UNIT_ASSIGNED_CONTEXT((#71493,#71495,#71496))
REPRESENTATION_CONTEXT('','3D')
);
#71492=(
GEOMETRIC_REPRESENTATION_CONTEXT(3)
GLOBAL_UNCERTAINTY_ASSIGNED_CONTEXT((#71471))
GLOBAL_UNIT_ASSIGNED_CONTEXT((#71493,#71495,#71496))
REPRESENTATION_CONTEXT('','3D')
);
#71493=(
LENGTH_UNIT()
NAMED_UNIT(*)
SI_UNIT(.CENTI.,.METRE.)
);
#71495=(
NAMED_UNIT(*)
PLANE_ANGLE_UNIT()
SI_UNIT($,.RADIAN.)
);
#71496=(
NAMED_UNIT(*)
SI_UNIT($,.STERADIAN.)
SOLID_ANGLE_UNIT()
);
#71509=SHAPE_DEFINITION_REPRESENTATION(#71529,#71614);
#71529=PRODUCT_DEFINITION_SHAPE('',$,#71635);
#71614=SHAPE_REPRESENTATION('',(#30164),#71484);
#71622=PRODUCT_DEFINITION_CONTEXT('part definition',#71684,'design');
#71635=PRODUCT_DEFINITION('2026-10-19-03-22-52-363',
'14_Ram_Return_Extension_Spring_D30x4',#71655,#71622);
#71655=PRODUCT_DEFINITION_FORMATION('',$,#71698);
#71684=APPLICATION_CONTEXT(
'Core Data for Automotive Mechanical Design Process');
#71685=PRODUCT_CONTEXT('part definition',#71684,'mechanical');
#71698=PRODUCT('2026-10-19-03-22-52-363',
'14_Ram_Return_Extension_Spring_D30x4',$,(#71685));
#71881=COLOUR_RGB('Grey',0.48,0.52,0.57);
#71882=FILL_AREA_STYLE_COLOUR('',#71881);
#71883=FILL_AREA_STYLE('',(#71882));
#71884=SURFACE_STYLE_FILL_AREA(#71883);
#71885=SURFACE_SIDE_STYLE('',(#71884));
#71886=SURFACE_STYLE_USAGE(.BOTH.,#71885);
#71887=PRESENTATION_STYLE_ASSIGNMENT((#71886));
ENDSEC;
END-ISO-10303-21;
